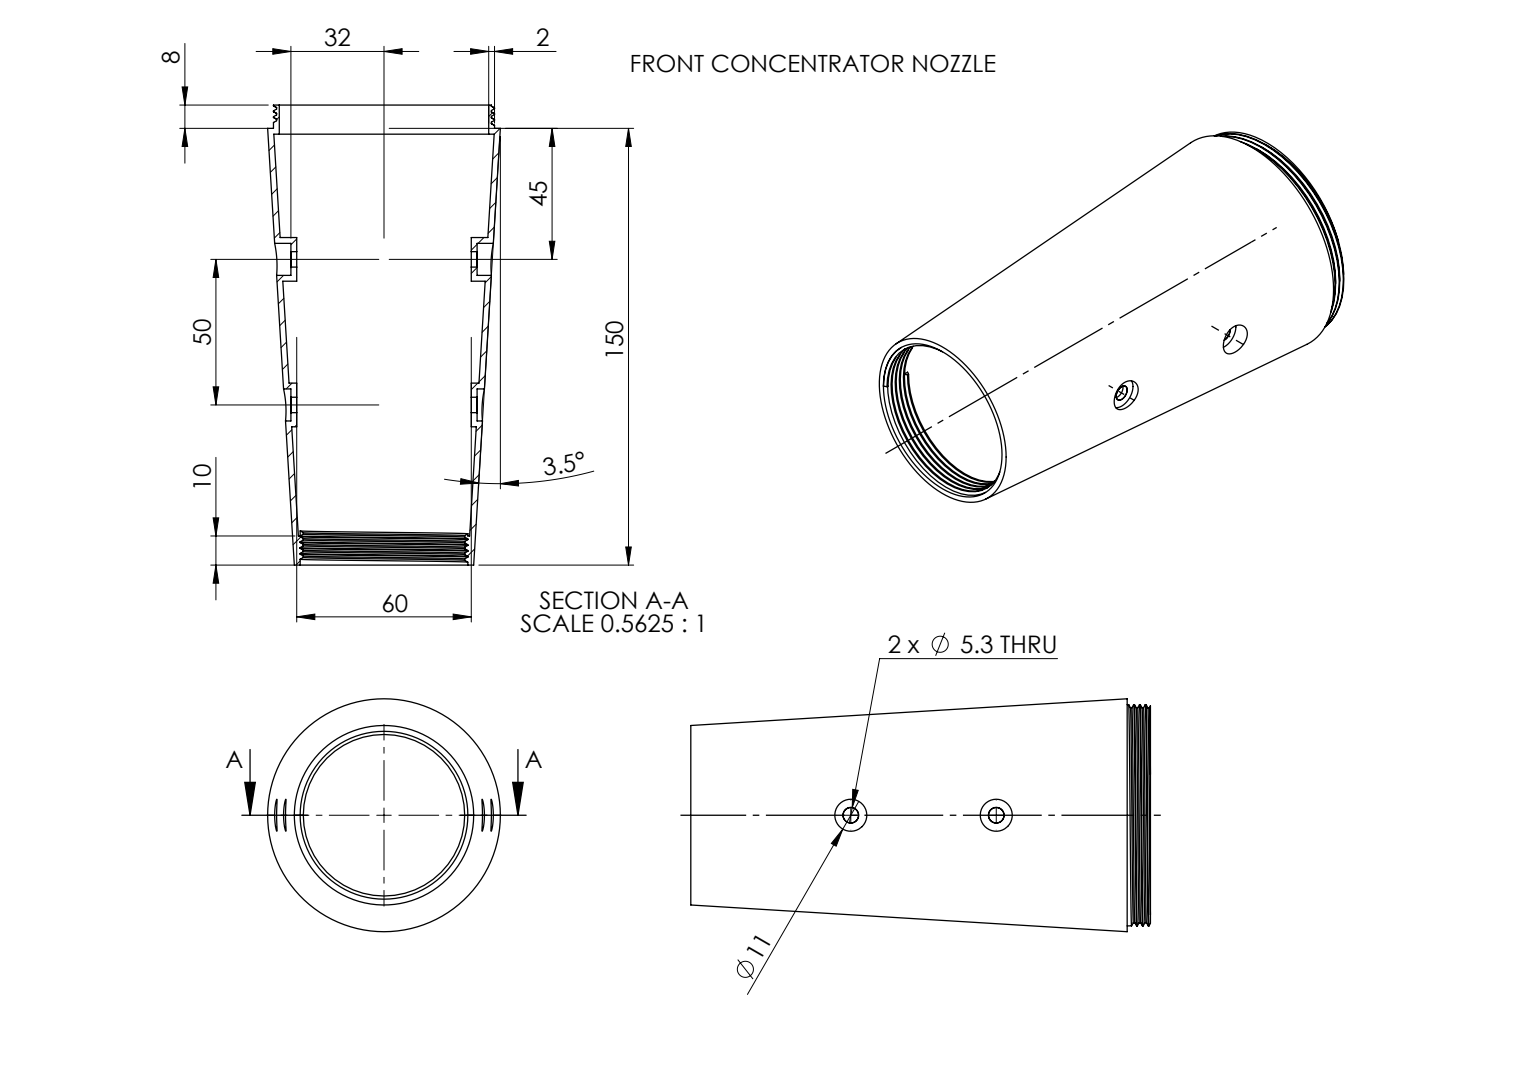
ISO-10303-21;
HEADER;
FILE_DESCRIPTION (('STEP AP214'),
    '1' );
FILE_NAME ('Front Concentrator Nozzle.step',
    '2026-10-04T13:31:42',
    ( '' ),
    ( '' ),
    'SwSTEP 2.0',
    'SolidWorks 2026',
    '' );
FILE_SCHEMA (( 'AUTOMOTIVE_DESIGN' ));
ENDSEC;

DATA;
#86=CARTESIAN_POINT ( 'NONE',  ( -31.23840969660177791, 7.314650797970922547, 96.67552899226033958 ) ) ;
#172=CARTESIAN_POINT ( 'NONE',  ( -11.40812507854755609, 35.11059874428196537, -7.524999997268813523 ) ) ;
#257=CARTESIAN_POINT ( 'NONE',  ( -36.88729982035408739, 1.776435236410510043, 50.21758054017369233 ) ) ;
#263=CARTESIAN_POINT ( 'NONE',  ( 22.44159573604009239, 16.30477369853692693, 146.0750000027311728 ) ) ;
#268=CARTESIAN_POINT ( 'NONE',  ( -5.359611314223446995E-15, 29.16686587814335496, 140.3750000027311842 ) ) ;
#301=EDGE_LOOP ( 'NONE', ( #33851, #130611, #76912, #84363 ) ) ;
#356=CARTESIAN_POINT ( 'NONE',  ( -23.31738231874055245, -16.94106989632524574, 144.4500000054623854 ) ) ;
#375=CYLINDRICAL_SURFACE ( 'NONE', #121053, 37.99626262588765968 ) ;
#425=CARTESIAN_POINT ( 'NONE',  ( 35.67631076299766590, 1.230297745838647261, 37.59750771353019871 ) ) ;
#465=DIRECTION ( 'NONE',  ( 0.000000000000000000, 0.000000000000000000, -1.000000000000000000 ) ) ;
#483=EDGE_LOOP ( 'NONE', ( #165279, #110182, #164294, #124142 ) ) ;
#616=CARTESIAN_POINT ( 'NONE',  ( 36.91746825000000598, -11.99521256947793546, -3.724999997268812812 ) ) ;
#704=CARTESIAN_POINT ( 'NONE',  ( -36.77423900702709858, -4.677204790287845526, 47.89930394225362420 ) ) ;
#735=CARTESIAN_POINT ( 'NONE',  ( 17.14385361876520264, -23.59649016807271238, 146.0750000027311728 ) ) ;
#760=CARTESIAN_POINT ( 'NONE',  ( 28.82186960331499392, -9.364793116373510529, 145.1500000054623456 ) ) ;
#773=EDGE_LOOP ( 'NONE', ( #134371, #137023, #169429, #7764 ) ) ;
#781=CARTESIAN_POINT ( 'NONE',  ( 8.906447517083057264, -27.41122689804191026, 142.5999999999999943 ) ) ;
#823=CARTESIAN_POINT ( 'NONE',  ( 37.99626262588763836, 12.34573411038918955, -2.647842220587803386 ) ) ;
#850=CARTESIAN_POINT ( 'NONE',  ( 8.571926809382603096, -26.38167802310801235, 145.4750000027311785 ) ) ;
#868=CARTESIAN_POINT ( 'NONE',  ( 11.74149087413294268, 36.13659316521247433, -6.602157773949822506 ) ) ;
#904=CARTESIAN_POINT ( 'NONE',  ( -8.906447517083060816, 27.41122689804195645, 149.5999999999999943 ) ) ;
#973=CARTESIAN_POINT ( 'NONE',  ( 3.556970738554033499E-15, -38.81732327939057825, -2.124999997268813612 ) ) ;
#974=CARTESIAN_POINT ( 'NONE',  ( -34.51819068884489639, 0.7175229865516564720, 89.53493623002425750 ) ) ;
#991=CARTESIAN_POINT ( 'NONE',  ( 29.86685920354754487, 21.69954338932564752, -3.924999997268812990 ) ) ;
#1033=ORIENTED_EDGE ( 'NONE', *, *, #63840, .F. ) ;
#1078=CARTESIAN_POINT ( 'NONE',  ( -32.23033374730685807, 4.573250637950163622, 89.03582022910542548 ) ) ;
#1088=CARTESIAN_POINT ( 'NONE',  ( -28.82186960331480208, 9.364793116373830273, 140.1500000054623740 ) ) ;
#1099=CYLINDRICAL_SURFACE ( 'NONE', #19317, 2.649999999999999467 ) ;
#1105=AXIS2_PLACEMENT_3D ( 'NONE', #147719, #164887, #181061 ) ;
#1163=CARTESIAN_POINT ( 'NONE',  ( -36.91746825000000598, 2.428612866367529932E-14, -7.124999997268813168 ) ) ;
#1250=AXIS2_PLACEMENT_3D ( 'NONE', #88283, #13443, #89288 ) ;
#1253=CARTESIAN_POINT ( 'NONE',  ( 22.44159573604009594, -16.30477369853687364, 148.1750000027311671 ) ) ;
#1258=CARTESIAN_POINT ( 'NONE',  ( -27.73933785331498925, -9.013057229001049109, 140.9750000027311501 ) ) ;
#1302=DIRECTION ( 'NONE',  ( 0.000000000000000000, 0.000000000000000000, 1.000000000000000000 ) ) ;
#1348=LINE ( 'NONE', #110523, #66983 ) ;
#1420=CARTESIAN_POINT ( 'NONE',  ( 34.67490207739297148, 3.335485537672782552, 51.73549893453298409 ) ) ;
#1511=ORIENTED_EDGE ( 'NONE', *, *, #22791, .F. ) ;
#1579=DIRECTION ( 'NONE',  ( 1.000000000000000000, -0.000000000000000000, 6.982962677686266711E-15 ) ) ;
#1583=CARTESIAN_POINT ( 'NONE',  ( 34.02657648861390527, -4.769071838117370454, 92.23683055719311596 ) ) ;
#1616=CARTESIAN_POINT ( 'NONE',  ( -29.86685920354755197, -21.69954338932560134, -4.424999997268812990 ) ) ;
#1692=DIRECTION ( 'NONE',  ( 0.000000000000000000, 0.000000000000000000, -1.000000000000000000 ) ) ;
#1709=CARTESIAN_POINT ( 'NONE',  ( -36.91128768240056957, -0.3593773198236934197, 50.50000000000003553 ) ) ;
#1739=CARTESIAN_POINT ( 'NONE',  ( -28.82186960331499037, 2.428612866367529932E-14, 150.0000000000000000 ) ) ;
#1764=CARTESIAN_POINT ( 'NONE',  ( -8.906447517083060816, 27.41122689804195645, 147.8500000054623627 ) ) ;
#1781=DIRECTION ( 'NONE',  ( 0.000000000000000000, -0.000000000000000000, -1.000000000000000000 ) ) ;
#1853=CARTESIAN_POINT ( 'NONE',  ( 27.73933785331498569, 2.768321779492822058E-14, 145.8750000027311842 ) ) ;
#1864=ADVANCED_FACE ( 'NONE', ( #142724 ), #159574, .T. ) ;
#1947=VERTEX_POINT ( 'NONE', #111400 ) ;
#1982=CARTESIAN_POINT ( 'NONE',  ( 11.40812507854755253, -35.11059874428192273, -10.52499999726881263 ) ) ;
#1987=EDGE_CURVE ( 'NONE', #137596, #48134, #24393, .T. ) ;
#1988=CARTESIAN_POINT ( 'NONE',  ( 33.68482864984028424, 4.779698632210292786, 97.74495643025990432 ) ) ;
#1999=CARTESIAN_POINT ( 'NONE',  ( -29.86685920354755552, 21.69954338932564397, -5.324999997268814234 ) ) ;
#2032=CARTESIAN_POINT ( 'NONE',  ( 34.45224964297659653, -5.970420695714325099, 49.56603145559587631 ) ) ;
#2046=AXIS2_PLACEMENT_3D ( 'NONE', #73162, #149985, #85294 ) ;
#2171=CARTESIAN_POINT ( 'NONE',  ( 11.40812507854754365, 35.11059874428196537, -7.724999997268813701 ) ) ;
#2215=DIRECTION ( 'NONE',  ( 0.000000000000000000, 0.000000000000000000, 1.000000000000000000 ) ) ;
#2256=CARTESIAN_POINT ( 'NONE',  ( 8.571926809382597767, 26.38167802310806209, 142.2750000027311899 ) ) ;
#2261=CARTESIAN_POINT ( 'NONE',  ( 1.784210473542230573E-15, -29.16686587814331588, 139.3750000027311842 ) ) ;
#2283=CIRCLE ( 'NONE', #5446, 0.2000000000000057288 ) ;
#2296=VERTEX_POINT ( 'NONE', #80063 ) ;
#2331=CARTESIAN_POINT ( 'NONE',  ( 8.571926809382603096, -26.38167802310801235, 143.9750000027312069 ) ) ;
#2582=CARTESIAN_POINT ( 'NONE',  ( 34.37111623004059169, -2.754365613946268443, 90.23597232697532888 ) ) ;
#2613=ORIENTED_EDGE ( 'NONE', *, *, #47794, .T. ) ;
#2618=CARTESIAN_POINT ( 'NONE',  ( -11.40812507854755609, 35.11059874428196537, -3.024999997268813523 ) ) ;
#2707=CARTESIAN_POINT ( 'NONE',  ( -37.99626262588766679, 2.428612866367529932E-14, -5.747842220587803475 ) ) ;
#2708=CARTESIAN_POINT ( 'NONE',  ( -37.19790397533368775, -4.369830079088519170, 41.64077531718623248 ) ) ;
#2736=CARTESIAN_POINT ( 'NONE',  ( 28.82186960331499392, -9.364793116373510529, 148.9000000000000057 ) ) ;
#2760=CARTESIAN_POINT ( 'NONE',  ( -27.73933785331498925, 9.013057229001089965, 148.7750000027311899 ) ) ;
#2851=CARTESIAN_POINT ( 'NONE',  ( -5.359611314223446995E-15, 29.16686587814335851, 144.3750000027311842 ) ) ;
#2869=CARTESIAN_POINT ( 'NONE',  ( 28.82186960331518222, 9.364793116373306248, 141.3500000054623911 ) ) ;
#2899=ORIENTED_EDGE ( 'NONE', *, *, #115308, .F. ) ;
#2975=CARTESIAN_POINT ( 'NONE',  ( 29.86685920354754487, 21.69954338932564752, -5.424999997268813878 ) ) ;
#2987=EDGE_CURVE ( 'NONE', #118975, #96409, #59563, .T. ) ;
#2993=CARTESIAN_POINT ( 'NONE',  ( 22.81625015709509441, 31.40387420917330275, -7.824999997268813345 ) ) ;
#3002=EDGE_LOOP ( 'NONE', ( #73351, #153883, #149706, #79021 ) ) ;
#3031=CARTESIAN_POINT ( 'NONE',  ( 34.75592306271658316, -1.707766843171824478, 52.30709029423474732 ) ) ;
#3169=CARTESIAN_POINT ( 'NONE',  ( 11.40812507854755253, -35.11059874428192273, -10.52499999726881263 ) ) ;
#3184=ORIENTED_EDGE ( 'NONE', *, *, #51790, .T. ) ;
#3210=CARTESIAN_POINT ( 'NONE',  ( -28.82186960331499037, 2.428612866367529932E-14, 149.1250000027311842 ) ) ;
#3216=CARTESIAN_POINT ( 'NONE',  ( -33.83559363775140838, -1.430799499857056789, 100.3228003899267975 ) ) ;
#3219=LINE ( 'NONE', #11975, #188941 ) ;
#3253=CARTESIAN_POINT ( 'NONE',  ( 17.14385361876520264, 23.59649016807275856, 148.6750000027311387 ) ) ;
#3325=CARTESIAN_POINT ( 'NONE',  ( -22.44159573604010305, 16.30477369853692338, 145.1750000027311671 ) ) ;
#3369=CARTESIAN_POINT ( 'NONE',  ( -28.82186960331494419, 9.364793116373629545, 147.8999999999999773 ) ) ;
#3373=DIRECTION ( 'NONE',  ( -1.000000000000000000, 0.000000000000000000, 0.000000000000000000 ) ) ;
#3407=ORIENTED_EDGE ( 'NONE', *, *, #43390, .F. ) ;
#3481=CARTESIAN_POINT ( 'NONE',  ( -36.91746825000000598, 2.428612866367529932E-14, -4.624999997268814056 ) ) ;
#3519=DIRECTION ( 'NONE',  ( 0.000000000000000000, 0.000000000000000000, 1.000000000000000000 ) ) ;
#3567=CARTESIAN_POINT ( 'NONE',  ( 33.68444218968561188, -5.327119193238885053, 96.41491933019777605 ) ) ;
#3600=CARTESIAN_POINT ( 'NONE',  ( 3.556970738554033499E-15, -38.81732327939057825, -8.124999997268814056 ) ) ;
#3673=CARTESIAN_POINT ( 'NONE',  ( -3.573655867282028392E-15, 2.428612866367529932E-14, 2.000000000000000000 ) ) ;
#3703=EDGE_CURVE ( 'NONE', #70870, #68071, #179075, .T. ) ;
#3721=CARTESIAN_POINT ( 'NONE',  ( -28.82186960331499037, 2.428612866367529932E-14, 148.0000000000000000 ) ) ;
#3743=CARTESIAN_POINT ( 'NONE',  ( 27.73933785331498569, 2.768321779492822058E-14, 147.8750000027311842 ) ) ;
#3833=CARTESIAN_POINT ( 'NONE',  ( 22.44159573604009594, -16.30477369853687364, 145.6750000027311671 ) ) ;
#3852=LINE ( 'NONE', #20027, #140137 ) ;
#3854=CARTESIAN_POINT ( 'NONE',  ( -37.99626262588766679, 2.428612866367529932E-14, -6.002157773949822861 ) ) ;
#3890=CARTESIAN_POINT ( 'NONE',  ( 23.31738231874054534, 16.94106989632529192, 149.1999999999999886 ) ) ;
#3957=CARTESIAN_POINT ( 'NONE',  ( 36.91746824999999887, 11.99521256947799053, -3.524999997268813079 ) ) ;
#3958=CARTESIAN_POINT ( 'NONE',  ( -33.83915642739259511, 1.250096592814743612, 100.3591031859434395 ) ) ;
#4011=CARTESIAN_POINT ( 'NONE',  ( 34.36934878537046956, -7.254149193659900519, 46.92043707032848943 ) ) ;
#4175=FACE_OUTER_BOUND ( 'NONE', #83053, .T. ) ;
#4234=CARTESIAN_POINT ( 'NONE',  ( -27.73933785331498925, 2.428612866367529932E-14, 138.8750000027311842 ) ) ;
#4242=CARTESIAN_POINT ( 'NONE',  ( -67.00000000000000000, -1.096058885236868847E-14, 100.5000000000010232 ) ) ;
#4305=CARTESIAN_POINT ( 'NONE',  ( 27.73933785331498569, 9.013057229001093518, 142.4750000027312069 ) ) ;
#4359=EDGE_CURVE ( 'NONE', #122084, #114881, #130090, .T. ) ;
#4381=CARTESIAN_POINT ( 'NONE',  ( 30.74264578624799782, 22.33583958711400541, -2.549999994537626602 ) ) ;
#4431=CARTESIAN_POINT ( 'NONE',  ( 32.00000000000000000, -1.230770033143102596E-14, 100.5000000000010232 ) ) ;
#4461=CARTESIAN_POINT ( 'NONE',  ( -22.81625015709510507, 31.40387420917330275, -6.924999997268812990 ) ) ;
#4548=CARTESIAN_POINT ( 'NONE',  ( 34.11707783341799427, -4.368959606072635005, 91.63974055655047835 ) ) ;
#4555=CLOSED_SHELL ( 'NONE', ( #90232, #12376, #39790, #49765, #196807, #195802, #5067, #178847, #90906, #29062, #71683, #37608, #132806, #83460, #86746, #142950, #9900, #188345, #21736, #102737, #129324, #36223, #83487, #180359, #110651, #151179, #135829, #116056, #163838, #21395, #184629, #66098, #113969, #161198, #91600, #44781, #54625, #152525, #139324, #99460, #181205, #19000, #32262, #11988, #77426, #192893, #49369, #139173, #138390, #165381, #24013, #108264, #157224, #194354, #83980, #9700, #103342, #135698, #72433, #186703, #66135, #146997, #103745, #47351, #199677, #22379, #63505, #38617, #191100, #189772, #111561, #137258, #44759, #98675, #18130, #51870, #110625, #156274, #9092, #133714, #77296, #1864 ) ) ;
#4582=CARTESIAN_POINT ( 'NONE',  ( -36.91746825000001309, 11.99521256947798342, -6.724999997268813701 ) ) ;
#4674=CARTESIAN_POINT ( 'NONE',  ( 31.26372923869871201, -6.750542664803641735, 98.30470173274461843 ) ) ;
#4689=VERTEX_POINT ( 'NONE', #24962 ) ;
#4691=AXIS2_PLACEMENT_3D ( 'NONE', #148800, #166959, #28461 ) ;
#4705=CARTESIAN_POINT ( 'NONE',  ( -28.82186960331499392, -9.364793116373526516, 146.1000000000000227 ) ) ;
#4727=CARTESIAN_POINT ( 'NONE',  ( -8.571926809382608425, 26.38167802310805854, 148.4750000027311785 ) ) ;
#4754=CARTESIAN_POINT ( 'NONE',  ( -28.82186960331499037, 2.428612866367529932E-14, 146.2500000054623683 ) ) ;
#4758=EDGE_CURVE ( 'NONE', #21601, #200018, #57632, .T. ) ;
#4944=CARTESIAN_POINT ( 'NONE',  ( 11.40812507854755253, -35.11059874428192273, -8.024999997268814411 ) ) ;
#4945=CARTESIAN_POINT ( 'NONE',  ( -33.81930014798969353, 1.942787237620518859, 100.1485738335251341 ) ) ;
#5003=ORIENTED_EDGE ( 'NONE', *, *, #126225, .F. ) ;
#5021=PLANE ( 'NONE',  #137868 ) ;
#5067=ADVANCED_FACE ( 'NONE', ( #165492 ), #104804, .F. ) ;
#5133=B_SPLINE_CURVE_WITH_KNOTS ( 'NONE', 3,
 ( #22604, #131776, #54935, #86265, #72103, #147955, #191443, #116607, #40770, #39759, #83256, #37764, #55931, #53938, #100430, #146946, #84250, #144931, #164126, #101422, #38774, #161108, #145931, #9442, #71107, #117606, #162111, #23608, #7413, #163114, #115613, #85254, #24617, #69096, #148953, #133776, #180309, #132773, #8435, #194460, #179306, #103443, #102439, #68094 ),
 .UNSPECIFIED., .F., .F.,
 ( 4, 2, 2, 2, 2, 2, 2, 2, 2, 2, 2, 2, 2, 2, 2, 2, 2, 2, 2, 2, 2, 4 ),
 ( 0.01750047681075387815, 0.01897230708297379873, 0.01970822221908375901, 0.02044413735519371930, 0.02191596762741363988, 0.02338779789963356393, 0.02485962817185348450, 0.02559554330796346561, 0.02633145844407343977, 0.02706737358018342088, 0.02780328871629339851, 0.02927511898851335725, 0.03074694926073331253, 0.03221877953295326780, 0.03295469466906326972, 0.03369060980517327164, 0.03516244007739326854, 0.03663427034961326545, 0.03737018548572325349, 0.03810610062183324154, 0.03957793089405323150, 0.04104976116627322147 ),
 .UNSPECIFIED. ) ;
#5169=DIRECTION ( 'NONE',  ( -1.000000000000000000, 0.000000000000000000, 0.000000000000000000 ) ) ;
#5174=EDGE_CURVE ( 'NONE', #71503, #154069, #101569, .T. ) ;
#5201=AXIS2_PLACEMENT_3D ( 'NONE', #184358, #1302, #42874 ) ;
#5229=CARTESIAN_POINT ( 'NONE',  ( 17.14385361876520264, -23.59649016807271238, 141.5750000027312012 ) ) ;
#5242=ORIENTED_EDGE ( 'NONE', *, *, #113163, .T. ) ;
#5303=CARTESIAN_POINT ( 'NONE',  ( -17.14385361876520975, 23.59649016807275856, 147.0750000027312012 ) ) ;
#5382=CARTESIAN_POINT ( 'NONE',  ( 23.48529157249600630, -32.32473071737749137, -7.049999994537626158 ) ) ;
#5402=ORIENTED_EDGE ( 'NONE', *, *, #181788, .T. ) ;
#5432=CARTESIAN_POINT ( 'NONE',  ( 11.40812507854754365, 35.11059874428196537, -3.724999997268813701 ) ) ;
#5446=AXIS2_PLACEMENT_3D ( 'NONE', #181467, #58113, #41956 ) ;
#5466=CARTESIAN_POINT ( 'NONE',  ( 11.40812507854755253, -35.11059874428192273, -2.024999997268813079 ) ) ;
#5554=CARTESIAN_POINT ( 'NONE',  ( 33.67956615508441587, -5.223713096473153072, 96.75862529643663379 ) ) ;
#5586=CARTESIAN_POINT ( 'NONE',  ( -29.86685920354755552, 21.69954338932564397, -8.824999997268815122 ) ) ;
#5680=CARTESIAN_POINT ( 'NONE',  ( 31.34418352700886601, -5.970234417100042101, 99.56646813413777863 ) ) ;
#5710=CARTESIAN_POINT ( 'NONE',  ( -23.31738231874055600, 16.94106989632528837, 149.7999999999999829 ) ) ;
#5731=CARTESIAN_POINT ( 'NONE',  ( -8.906447517083060816, 27.41122689804195645, 139.8500000054623911 ) ) ;
#5760=CARTESIAN_POINT ( 'NONE',  ( -17.81289503416611097, -24.51734667627696496, 146.5500000054623513 ) ) ;
#5769=ORIENTED_EDGE ( 'NONE', *, *, #148652, .F. ) ;
#5827=CARTESIAN_POINT ( 'NONE',  ( -17.14385361876520264, -23.59649016807271238, 139.1750000027311671 ) ) ;
#5946=CARTESIAN_POINT ( 'NONE',  ( 36.91746825000000598, -11.99521256947793546, -5.724999997268813701 ) ) ;
#5947=CARTESIAN_POINT ( 'NONE',  ( -33.90110335395768715, 5.206480924673157595, 93.21819085016213080 ) ) ;
#6003=DIRECTION ( 'NONE',  ( -7.709882115452472644E-15, 0.000000000000000000, 1.000000000000000000 ) ) ;
#6011=ORIENTED_EDGE ( 'NONE', *, *, #13792, .F. ) ;
#6026=CARTESIAN_POINT ( 'NONE',  ( -30.73962218707678673, 22.33364281372846705, -4.202157773949823927 ) ) ;
#6033=CARTESIAN_POINT ( 'NONE',  ( -40.00200000000003087, -1.071565949253934124E-14, 102.5000000000000142 ) ) ;
#6193=CARTESIAN_POINT ( 'NONE',  ( 14.18669005401828187, -34.08280046153741694, -8.000000000000001776 ) ) ;
#6232=CARTESIAN_POINT ( 'NONE',  ( 22.44159573604009239, 16.30477369853692693, 146.5750000027312012 ) ) ;
#6301=CARTESIAN_POINT ( 'NONE',  ( -32.00000000000000711, -5.510910596163089556E-15, 45.00000000000000000 ) ) ;
#6303=CARTESIAN_POINT ( 'NONE',  ( -5.359611314223446995E-15, 29.16686587814335851, 144.8750000027311842 ) ) ;
#6343=CARTESIAN_POINT ( 'NONE',  ( -31.80000000000000782, -1.130348995613007185E-14, 97.69999999999998863 ) ) ;
#6378=CARTESIAN_POINT ( 'NONE',  ( 30.74264578624799782, 22.33583958711400541, -6.549999994537627046 ) ) ;
#6427=CARTESIAN_POINT ( 'NONE',  ( -22.81625015709509441, -31.40387420917324590, -6.824999997268814234 ) ) ;
#6429=DIRECTION ( 'NONE',  ( 0.000000000000000000, 0.000000000000000000, -1.000000000000000000 ) ) ;
#6440=AXIS2_PLACEMENT_3D ( 'NONE', #168862, #94012, #61681 ) ;
#6459=CARTESIAN_POINT ( 'NONE',  ( -29.86685920354755552, 21.69954338932564397, -2.824999997268813345 ) ) ;
#6551=EDGE_CURVE ( 'NONE', #147696, #97386, #74235, .T. ) ;
#6582=CARTESIAN_POINT ( 'NONE',  ( -22.81625015709510507, 31.40387420917330275, -6.924999997268812990 ) ) ;
#6646=ORIENTED_EDGE ( 'NONE', *, *, #14461, .F. ) ;
#6703=CARTESIAN_POINT ( 'NONE',  ( -8.906447517083053711, -27.41122689804191026, 144.4000000000000057 ) ) ;
#6726=CARTESIAN_POINT ( 'NONE',  ( -8.906447517083053711, -27.41122689804191026, 142.6500000054623740 ) ) ;
#6736=SURFACE_STYLE_FILL_AREA ( #179627 ) ;
#6834=CARTESIAN_POINT ( 'NONE',  ( 23.31738231874054890, -16.94106989632523508, 148.7999999999999829 ) ) ;
#6838=CARTESIAN_POINT ( 'NONE',  ( 32.00000000000000000, -1.163414459189985801E-14, 92.35000000000000853 ) ) ;
#6875=ORIENTED_EDGE ( 'NONE', *, *, #116835, .F. ) ;
#6939=CARTESIAN_POINT ( 'NONE',  ( -29.86685920354755552, 21.69954338932564397, -8.824999997268815122 ) ) ;
#7104=ORIENTED_EDGE ( 'NONE', *, *, #128488, .T. ) ;
#7139=DIRECTION ( 'NONE',  ( 1.000000000000000000, 0.000000000000000000, 0.000000000000000000 ) ) ;
#7143=CARTESIAN_POINT ( 'NONE',  ( 36.44859680441125960, 5.987861874135487206, -7.999999999999996447 ) ) ;
#7191=CARTESIAN_POINT ( 'NONE',  ( 9.138071159678322175, -35.85733837751254782, -7.999999999999996447 ) ) ;
#7202=ORIENTED_EDGE ( 'NONE', *, *, #67479, .F. ) ;
#7228=CARTESIAN_POINT ( 'NONE',  ( 27.73933785331498214, 9.013057229001095294, 142.4750000027311785 ) ) ;
#7301=CARTESIAN_POINT ( 'NONE',  ( 17.14385361876520264, -23.59649016807270883, 142.0750000027311444 ) ) ;
#7304=DIRECTION ( 'NONE',  ( -1.000000000000000000, 0.000000000000000000, 0.000000000000000000 ) ) ;
#7377=CARTESIAN_POINT ( 'NONE',  ( -11.74264578624799782, -36.14014761921581709, -3.349999994537626868 ) ) ;
#7392=ORIENTED_EDGE ( 'NONE', *, *, #132031, .F. ) ;
#7413=CARTESIAN_POINT ( 'NONE',  ( 31.68669428337295102, 6.716517432552111977, 91.65365426639641555 ) ) ;
#7416=ORIENTED_EDGE ( 'NONE', *, *, #68419, .F. ) ;
#7428=CARTESIAN_POINT ( 'NONE',  ( -36.91746825000000598, 2.428612866367529932E-14, -5.124999997268813168 ) ) ;
#7459=CARTESIAN_POINT ( 'NONE',  ( -22.81625015709509441, -31.40387420917324590, -2.324999997268813345 ) ) ;
#7498=CARTESIAN_POINT ( 'NONE',  ( -30.00000000000000000, -1.130961319012580892E-14, 92.35000000000000853 ) ) ;
#7581=CARTESIAN_POINT ( 'NONE',  ( 36.91746825000000598, -11.99521256947793546, -5.724999997268813701 ) ) ;
#7615=AXIS2_PLACEMENT_3D ( 'NONE', #110151, #93979, #124319 ) ;
#7703=CARTESIAN_POINT ( 'NONE',  ( -28.82186960331499037, 2.428612866367529932E-14, 139.9999999999999716 ) ) ;
#7762=SHAPE_DEFINITION_REPRESENTATION ( #187433, #31381 ) ;
#7764=ORIENTED_EDGE ( 'NONE', *, *, #187248, .F. ) ;
#7876=DIRECTION ( 'NONE',  ( 0.000000000000000000, 0.000000000000000000, -1.000000000000000000 ) ) ;
#7934=EDGE_CURVE ( 'NONE', #98202, #176832, #121982, .T. ) ;
#7945=CARTESIAN_POINT ( 'NONE',  ( -17.14385361876520619, 23.59649016807275856, 149.0750000027311728 ) ) ;
#7982=CIRCLE ( 'NONE', #120998, 0.1999999999999987899 ) ;
#8002=DIRECTION ( 'NONE',  ( -0.000000000000000000, -0.000000000000000000, -1.000000000000000000 ) ) ;
#8146=CARTESIAN_POINT ( 'NONE',  ( 37.99626262588765258, -12.34573411038911672, -5.102157773949822506 ) ) ;
#8153=CARTESIAN_POINT ( 'NONE',  ( 29.32033176666156393, -22.46488766722420749, -8.000000000000003553 ) ) ;
#8154=EDGE_CURVE ( 'NONE', #53763, #106856, #120793, .T. ) ;
#8167=EDGE_LOOP ( 'NONE', ( #3184, #164472 ) ) ;
#8243=CARTESIAN_POINT ( 'NONE',  ( -22.44159573604010305, 16.30477369853692338, 143.1750000027311671 ) ) ;
#8248=CARTESIAN_POINT ( 'NONE',  ( -37.99626262588765968, -12.34573411038913626, -5.647842220587802942 ) ) ;
#8255=ORIENTED_EDGE ( 'NONE', *, *, #28811, .T. ) ;
#8281=VERTEX_POINT ( 'NONE', #97815 ) ;
#8320=CARTESIAN_POINT ( 'NONE',  ( -27.73933785331498925, 9.013057229001088189, 141.2750000027311899 ) ) ;
#8397=CARTESIAN_POINT ( 'NONE',  ( -30.74264578624800492, -22.33583958711396278, -7.549999994537627934 ) ) ;
#8406=ORIENTED_EDGE ( 'NONE', *, *, #70616, .F. ) ;
#8435=CARTESIAN_POINT ( 'NONE',  ( 32.45668260148360673, 3.101559039593180689, 88.16695215365970739 ) ) ;
#8605=CARTESIAN_POINT ( 'NONE',  ( 30.74264578624800137, -22.33583958711395212, -3.200000000000000178 ) ) ;
#8657=VECTOR ( 'NONE', #192387, 1000.000000000000000 ) ;
#8719=FACE_BOUND ( 'NONE', #63868, .T. ) ;
#8727=CARTESIAN_POINT ( 'NONE',  ( -28.82186960331499392, 9.364793116373565596, 148.1500000054624024 ) ) ;
#8729=CARTESIAN_POINT ( 'NONE',  ( 17.81289503416610742, 24.51734667627700404, 143.5500000054623513 ) ) ;
#8760=SURFACE_SIDE_STYLE ('',( #6736 ) ) ;
#8850=CIRCLE ( 'NONE', #154180, 35.99626262588765258 ) ;
#8921=EDGE_CURVE ( 'NONE', #11483, #170159, #195880, .T. ) ;
#8934=CARTESIAN_POINT ( 'NONE',  ( 28.83912964652353494, 23.35006605898203347, -8.000000000000001776 ) ) ;
#8944=AXIS2_PLACEMENT_3D ( 'NONE', #117188, #55516, #86851 ) ;
#8966=CARTESIAN_POINT ( 'NONE',  ( 11.40812507854754365, 35.11059874428196537, -9.224999997268813701 ) ) ;
#8977=AXIS2_PLACEMENT_3D ( 'NONE', #29250, #183915, #153562 ) ;
#8990=CARTESIAN_POINT ( 'NONE',  ( -34.40742850069382541, 7.501893140248845349, 45.46088305597102419 ) ) ;
#8996=CARTESIAN_POINT ( 'NONE',  ( 30.00000000000000000, -1.130961319012580892E-14, 97.65000000000000568 ) ) ;
#9032=VERTEX_POINT ( 'NONE', #57353 ) ;
#9083=AXIS2_PLACEMENT_3D ( 'NONE', #99154, #180038, #22332 ) ;
#9092=ADVANCED_FACE ( 'NONE', ( #165528 ), #46870, .T. ) ;
#9217=CARTESIAN_POINT ( 'NONE',  ( -34.40553910806575999, -2.436532241128162468, 90.06585364601160393 ) ) ;
#9219=CARTESIAN_POINT ( 'NONE',  ( -6.782741387738352223, -36.64508735834520081, -7.999999999999996447 ) ) ;
#9257=CARTESIAN_POINT ( 'NONE',  ( 17.14385361876520264, -23.59649016807271238, 146.0750000027311728 ) ) ;
#9332=CARTESIAN_POINT ( 'NONE',  ( 22.44159573604009594, -16.30477369853687364, 147.6750000027311671 ) ) ;
#9405=CARTESIAN_POINT ( 'NONE',  ( -38.00000000000001421, 12.34694845685046438, -7.849999994537626868 ) ) ;
#9442=CARTESIAN_POINT ( 'NONE',  ( 31.33330333603523954, 7.497710212630238402, 94.47580324309009825 ) ) ;
#9445=ORIENTED_EDGE ( 'NONE', *, *, #103944, .F. ) ;
#9449=CARTESIAN_POINT ( 'NONE',  ( 31.31738933903719513, -7.498949511226639331, 94.72411213025004884 ) ) ;
#9613=CARTESIAN_POINT ( 'NONE',  ( 38.00000000000000000, 12.34694845685046616, -2.900000000000000355 ) ) ;
#9665=AXIS2_PLACEMENT_3D ( 'NONE', #94111, #58812, #184156 ) ;
#9675=ORIENTED_EDGE ( 'NONE', *, *, #13792, .T. ) ;
#9700=ADVANCED_FACE ( 'NONE', ( #80442 ), #71788, .T. ) ;
#9732=CARTESIAN_POINT ( 'NONE',  ( -23.31738231874055600, 16.94106989632528837, 143.7999999999999829 ) ) ;
#9785=CARTESIAN_POINT ( 'NONE',  ( -6.019987952026120409E-15, 39.95163481335720235, -0.5021577739498228610 ) ) ;
#9796=ORIENTED_EDGE ( 'NONE', *, *, #93300, .F. ) ;
#9847=CARTESIAN_POINT ( 'NONE',  ( -28.82186960331499037, 2.781578969918950771E-14, 139.9999999999999716 ) ) ;
#9900=ADVANCED_FACE ( 'NONE', ( #169233 ), #375, .T. ) ;
#9940=CARTESIAN_POINT ( 'NONE',  ( 8.906447517083057264, -27.41122689804191026, 144.5999999999999943 ) ) ;
#9967=CARTESIAN_POINT ( 'NONE',  ( -11.40812507854754720, -35.11059874428192273, -10.22499999726881548 ) ) ;
#9990=CARTESIAN_POINT ( 'NONE',  ( -34.57898328185102343, 4.579095689294062410, 50.94499274836915248 ) ) ;
#10067=CARTESIAN_POINT ( 'NONE',  ( 32.00000000000000000, -6.184466335694137604E-15, 50.50000000000002842 ) ) ;
#10100=CARTESIAN_POINT ( 'NONE',  ( 11.74149087413294268, 36.13659316521247433, -2.602157773949823394 ) ) ;
#10216=CARTESIAN_POINT ( 'NONE',  ( -34.48725679702496194, -1.430676605895445430, 89.67714645826994513 ) ) ;
#10218=CARTESIAN_POINT ( 'NONE',  ( -34.63926591227897234, -15.08268834117409973, -8.000000000000003553 ) ) ;
#10251=ORIENTED_EDGE ( 'NONE', *, *, #50509, .T. ) ;
#10256=CARTESIAN_POINT ( 'NONE',  ( -8.571926809382608425, 26.38167802310805854, 144.9750000027312069 ) ) ;
#10261=( NAMED_UNIT ( * ) PLANE_ANGLE_UNIT ( ) SI_UNIT ( $, .RADIAN. ) );
#10405=CARTESIAN_POINT ( 'NONE',  ( -22.81625015709510507, 31.40387420917330275, -1.424999997268813212 ) ) ;
#10499=CARTESIAN_POINT ( 'NONE',  ( -8.571926809382608425, 26.38167802310805854, 146.4750000027311785 ) ) ;
#10532=ORIENTED_EDGE ( 'NONE', *, *, #7934, .F. ) ;
#10570=CARTESIAN_POINT ( 'NONE',  ( -31.23718726401125068, 7.254977440570235636, 96.91727682732809512 ) ) ;
#10571=CARTESIAN_POINT ( 'NONE',  ( 17.81289503416611453, -24.51734667627695785, 146.6999999999999886 ) ) ;
#10614=CARTESIAN_POINT ( 'NONE',  ( -38.00000000000001421, -12.34694845685042708, -5.900000000000000355 ) ) ;
#10674=EDGE_LOOP ( 'NONE', ( #77033, #138944, #32774, #21666 ) ) ;
#10732=CARTESIAN_POINT ( 'NONE',  ( 8.906447517083057264, -27.41122689804191026, 140.5999999999999943 ) ) ;
#10829=CONICAL_SURFACE ( 'NONE', #7615, 38.00373040315628259, 0.06108652381980166773 ) ;
#10936=CARTESIAN_POINT ( 'NONE',  ( -30.00000000000000000, -1.163414459189985801E-14, 87.50000000000000000 ) ) ;
#10962=CARTESIAN_POINT ( 'NONE',  ( 8.571926809382597767, 26.38167802310806209, 148.7750000027311899 ) ) ;
#10987=CARTESIAN_POINT ( 'NONE',  ( -34.77757469352546593, 0.9858555240219201155, 52.45108825929359142 ) ) ;
#11017=FACE_OUTER_BOUND ( 'NONE', #161873, .T. ) ;
#11100=CARTESIAN_POINT ( 'NONE',  ( -23.48298174826590667, 32.32155151706776053, -2.302157773949822683 ) ) ;
#11133=ORIENTED_EDGE ( 'NONE', *, *, #149523, .F. ) ;
#11213=CARTESIAN_POINT ( 'NONE',  ( 36.91746825000000598, -11.99521256947793546, -4.224999997268812812 ) ) ;
#11221=CARTESIAN_POINT ( 'NONE',  ( -37.99533089065118219, -0.2660902954431525469, -7.999999999999996447 ) ) ;
#11262=CARTESIAN_POINT ( 'NONE',  ( 8.571926809382603096, -26.38167802310801235, 139.9750000027311785 ) ) ;
#11410=CARTESIAN_POINT ( 'NONE',  ( 23.48529157249600630, -32.32473071737749137, -11.04999999453762527 ) ) ;
#11467=CARTESIAN_POINT ( 'NONE',  ( -34.74703293042581009, -1.945922946419438082, 52.24735972161445829 ) ) ;
#11483=VERTEX_POINT ( 'NONE', #13342 ) ;
#11496=CARTESIAN_POINT ( 'NONE',  ( -37.11214605083871731, 4.768680519348648339, 42.23634591622183621 ) ) ;
#11508=CARTESIAN_POINT ( 'NONE',  ( 17.14385361876520264, -23.59649016807271238, 145.5750000027312012 ) ) ;
#11622=CARTESIAN_POINT ( 'NONE',  ( -23.48529157249600985, 32.32473071737754111, -6.300000000000000711 ) ) ;
#11628=CARTESIAN_POINT ( 'NONE',  ( -30.00000000000000000, -1.163414459189985801E-14, 95.00000000000000000 ) ) ;
#11713=LINE ( 'NONE', #73380, #83913 ) ;
#11876=CARTESIAN_POINT ( 'NONE',  ( -32.00000000000000000, -1.163414459189985801E-14, 97.65000000000000568 ) ) ;
#11878=CARTESIAN_POINT ( 'NONE',  ( 37.57652299961964104, -0.7251171387572892257, 39.53617709569549277 ) ) ;
#11945=CARTESIAN_POINT ( 'NONE',  ( -3.573655867282028392E-15, 2.428612866367529932E-14, 139.9999999999999716 ) ) ;
#11973=CARTESIAN_POINT ( 'NONE',  ( 8.571926809382603096, -26.38167802310801235, 141.9750000027312069 ) ) ;
#11975=CARTESIAN_POINT ( 'NONE',  ( 37.99626262588765258, 2.893932880411085066E-14, 2.000000000000000000 ) ) ;
#11980=CARTESIAN_POINT ( 'NONE',  ( 30.00000000000000000, -5.186379194389041255E-15, 47.64999999999999858 ) ) ;
#11988=ADVANCED_FACE ( 'NONE', ( #52612 ), #20278, .T. ) ;
#12108=CARTESIAN_POINT ( 'NONE',  ( -11.74149087413295511, 36.13659316521247433, -4.147842220587803830 ) ) ;
#12202=AXIS2_PLACEMENT_3D ( 'NONE', #109134, #184987, #46471 ) ;
#12219=CARTESIAN_POINT ( 'NONE',  ( -29.86685920354755197, -21.69954338932560134, -4.924999997268813878 ) ) ;
#12225=CARTESIAN_POINT ( 'NONE',  ( -2.219726742498586258, -37.13270733954487213, -7.999999999999996447 ) ) ;
#12284=AXIS2_PLACEMENT_3D ( 'NONE', #126369, #112200, #6003 ) ;
#12376=ADVANCED_FACE ( 'NONE', ( #83104 ), #169393, .T. ) ;
#12407=CARTESIAN_POINT ( 'NONE',  ( 11.40812507854754365, 35.11059874428196537, -1.724999997268813479 ) ) ;
#12491=CARTESIAN_POINT ( 'NONE',  ( -37.43947335741456328, 2.756686112915582854, 40.22705064412460274 ) ) ;
#12497=CARTESIAN_POINT ( 'NONE',  ( 8.571926809382603096, -26.38167802310801235, 143.4750000027312069 ) ) ;
#12502=CARTESIAN_POINT ( 'NONE',  ( -8.571926809382608425, 26.38167802310805854, 142.4750000027312069 ) ) ;
#12591=EDGE_CURVE ( 'NONE', #81412, #115964, #185427, .T. ) ;
#12610=CARTESIAN_POINT ( 'NONE',  ( -23.48529157249599919, -32.32473071737750558, -5.700000000000000178 ) ) ;
#12659=CARTESIAN_POINT ( 'NONE',  ( 34.78522506798721992, 2.428612866353961525E-14, 52.50000000000000000 ) ) ;
#12807=CARTESIAN_POINT ( 'NONE',  ( -67.00000000000000000, -5.510910596163089556E-15, 45.00000000000000000 ) ) ;
#12852=EDGE_CURVE ( 'NONE', #70870, #34628, #145778, .T. ) ;
#12924=CARTESIAN_POINT ( 'NONE',  ( -16.59625950682774231, 33.98852600706017313, -7.999999999999994671 ) ) ;
#12927=CARTESIAN_POINT ( 'NONE',  ( -28.82186960331518932, -9.364793116373263615, 140.3500000054623627 ) ) ;
#12942=ORIENTED_EDGE ( 'NONE', *, *, #95173, .F. ) ;
#12956=CARTESIAN_POINT ( 'NONE',  ( -17.14385361876520264, -23.59649016807271593, 141.6750000027311103 ) ) ;
#12981=CARTESIAN_POINT ( 'NONE',  ( 28.82186960331498327, 2.781578969918950771E-14, 145.2500000054623683 ) ) ;
#13004=CARTESIAN_POINT ( 'NONE',  ( -40.00200000000003087, -5.510910596163089556E-15, 45.00000000000000000 ) ) ;
#13057=DIRECTION ( 'NONE',  ( 1.000000000000000000, 0.000000000000000000, 3.709348145883536076E-20 ) ) ;
#13120=ORIENTED_EDGE ( 'NONE', *, *, #12852, .T. ) ;
#13198=CARTESIAN_POINT ( 'NONE',  ( 29.86685920354754842, -21.69954338932559068, -10.32499999726881335 ) ) ;
#13204=CARTESIAN_POINT ( 'NONE',  ( 34.35276339089875108, 2.907959671212061004, 90.32815265678038941 ) ) ;
#13242=CARTESIAN_POINT ( 'NONE',  ( -17.14385361876520264, -23.59649016807271593, 139.6750000027311955 ) ) ;
#13270=DIRECTION ( 'NONE',  ( 0.000000000000000000, 0.000000000000000000, -1.000000000000000000 ) ) ;
#13305=ORIENTED_EDGE ( 'NONE', *, *, #168447, .F. ) ;
#13342=CARTESIAN_POINT ( 'NONE',  ( -28.82186960331499037, 2.428612866367529932E-14, 148.0000000000000000 ) ) ;
#13380=CARTESIAN_POINT ( 'NONE',  ( -36.91746825000001309, 11.99521256947798342, -1.224999997268813035 ) ) ;
#13443=DIRECTION ( 'NONE',  ( -1.000000000000000000, 0.000000000000000000, 0.000000000000000000 ) ) ;
#13461=CARTESIAN_POINT ( 'NONE',  ( -36.90816834587730000, 0.7173862878750039140, 50.46507289210754266 ) ) ;
#13466=EDGE_CURVE ( 'NONE', #80486, #64642, #91865, .T. ) ;
#13468=CARTESIAN_POINT ( 'NONE',  ( 27.73933785331498569, 2.768321779492822058E-14, 145.8750000027311842 ) ) ;
#13473=CARTESIAN_POINT ( 'NONE',  ( 22.44159573604009594, -16.30477369853687364, 141.6750000027311671 ) ) ;
#13541=CARTESIAN_POINT ( 'NONE',  ( -23.31738231874055245, -16.94106989632524574, 146.1999999999999886 ) ) ;
#13579=CARTESIAN_POINT ( 'NONE',  ( 23.48529157249600630, -32.32473071737749137, -9.300000000000002487 ) ) ;
#13582=FACE_OUTER_BOUND ( 'NONE', #190809, .T. ) ;
#13631=CARTESIAN_POINT ( 'NONE',  ( 34.64436006561229675, 3.766901597203519803, 51.50401746017936944 ) ) ;
#13792=EDGE_CURVE ( 'NONE', #56681, #90959, #182815, .T. ) ;
#13885=CIRCLE ( 'NONE', #126873, 37.87393738558669298 ) ;
#13929=CARTESIAN_POINT ( 'NONE',  ( -5.359611314223446995E-15, 29.16686587814335496, 144.8750000027311557 ) ) ;
#13953=CARTESIAN_POINT ( 'NONE',  ( 17.81289503416611453, -24.51734667627695785, 144.9500000054623854 ) ) ;
#13961=EDGE_CURVE ( 'NONE', #82818, #68886, #72967, .T. ) ;
#13982=CARTESIAN_POINT ( 'NONE',  ( -37.99626262588766679, 2.428612866367529932E-14, -1.747842220587805251 ) ) ;
#14016=CARTESIAN_POINT ( 'NONE',  ( -40.00200000000003087, -1.071565949253934124E-14, 102.5000000000000142 ) ) ;
#14041=CARTESIAN_POINT ( 'NONE',  ( -17.14385361876520975, 23.59649016807275856, 141.0750000027311728 ) ) ;
#14053=CIRCLE ( 'NONE', #127048, 2.700000000000001066 ) ;
#14075=B_SPLINE_CURVE_WITH_KNOTS ( 'NONE', 3,
 ( #94989, #75843, #108166, #63667, #47511, #78820, #74867, #169848, #13204, #167868, #137520, #199202, #186029, #198210, #184033, #14174, #59681, #77829, #140499, #168841, #155672, #44530, #123327, #60669, #122344, #93991, #1988, #31342, #109167, #106185, #183046, #138508, #45515, #92993, #121353, #29368, #17167, #154679, #30346, #90999 ),
 .UNSPECIFIED., .F., .F.,
 ( 4, 2, 2, 2, 2, 2, 2, 2, 2, 2, 2, 2, 2, 2, 2, 2, 2, 2, 2, 4 ),
 ( 0.004339806180219612543, 0.005417599276633671204, 0.006495392373047728998, 0.007034288921254766569, 0.007573185469461804140, 0.008650978565875881016, 0.009728771662289961361, 0.01080656475870404171, 0.01134546130691106020, 0.01188435785511808215, 0.01296215095153212260, 0.01403994404794615958, 0.01511773714436020002, 0.01619553024077424047, 0.01727332333718827745, 0.01835111643360231790, 0.01942890953001635487, 0.01996780607822336642, 0.02050670262643038144, 0.02158449572284441148 ),
 .UNSPECIFIED. ) ;
#14124=CARTESIAN_POINT ( 'NONE',  ( -37.58407650405589351, 1.968340676919130544E-14, 39.49999999999996447 ) ) ;
#14168=CARTESIAN_POINT ( 'NONE',  ( -22.81625015709510507, 31.40387420917330275, -9.424999997268812990 ) ) ;
#14174=CARTESIAN_POINT ( 'NONE',  ( 33.92112623720979059, 5.144804392130072124, 93.04721607740081879 ) ) ;
#14186=CARTESIAN_POINT ( 'NONE',  ( 11.40812507854754365, 35.11059874428196537, -5.724999997268812812 ) ) ;
#14250=VERTEX_POINT ( 'NONE', #128020 ) ;
#14259=( BOUNDED_CURVE ( )  B_SPLINE_CURVE ( 2, ( #54227, #8727, #193753, #106697, #135079, #181576, #168370, #91503, #150246, #45039, #29866 ),
 .UNSPECIFIED., .F., .F. ) 
 B_SPLINE_CURVE_WITH_KNOTS ( ( 3, 2, 2, 2, 2, 3 ),
 ( 0.000000000000000000, 0.02000000000000001776, 0.04000000000000003553, 0.06000000000000005329, 0.08000000000000007105, 0.1000000000000000888 ),
 .UNSPECIFIED. ) 
 CURVE ( )  GEOMETRIC_REPRESENTATION_ITEM ( )  RATIONAL_B_SPLINE_CURVE ( ( 1.000000000000000000, 0.9510565162951535312, 1.000000000000000000, 0.9510565162951535312, 1.000000000000000000, 0.9510565162951535312, 1.000000000000000000, 0.9510565162951535312, 1.000000000000000000, 0.9510565162951533091, 1.000000000000000222 ) ) 
 REPRESENTATION_ITEM ( '' )  );
#14262=CARTESIAN_POINT ( 'NONE',  ( -28.82186960331514669, -9.364793116373306248, 142.3500000054623911 ) ) ;
#14274=CARTESIAN_POINT ( 'NONE',  ( -31.64616484836360755, 2.655180720736634026, 102.0186121717492824 ) ) ;
#14328=CARTESIAN_POINT ( 'NONE',  ( -30.00000000000000000, -5.510910596163089556E-15, 45.00000000000000000 ) ) ;
#14363=CARTESIAN_POINT ( 'NONE',  ( 11.40812507854755253, -35.11059874428192273, -6.524999997268813523 ) ) ;
#14453=CARTESIAN_POINT ( 'NONE',  ( -5.359611314223446995E-15, 29.16686587814335496, 146.3750000027311842 ) ) ;
#14458=CARTESIAN_POINT ( 'NONE',  ( 17.14385361876520264, 23.59649016807275856, 142.1750000027311671 ) ) ;
#14461=EDGE_CURVE ( 'NONE', #89527, #45563, #88726, .T. ) ;
#14676=AXIS2_PLACEMENT_3D ( 'NONE', #64731, #192053, #127378 ) ;
#14682=EDGE_LOOP ( 'NONE', ( #50120, #17366 ) ) ;
#14703=AXIS2_PLACEMENT_3D ( 'NONE', #109409, #112392, #48747 ) ;
#14781=DIRECTION ( 'NONE',  ( -1.000000000000000000, -0.000000000000000000, -3.709348145883536076E-20 ) ) ;
#14817=CARTESIAN_POINT ( 'NONE',  ( 36.91746824999999887, 11.99521256947799053, -1.524999997268813745 ) ) ;
#14934=CARTESIAN_POINT ( 'NONE',  ( 27.73933785331498569, 2.768321779492822058E-14, 144.3750000027311842 ) ) ;
#14957=CARTESIAN_POINT ( 'NONE',  ( -35.68624576866248788, 0.9837712456775835612, 37.56068211393102274 ) ) ;
#15045=CARTESIAN_POINT ( 'NONE',  ( -17.14385361876520264, -23.59649016807271238, 141.1750000027311671 ) ) ;
#15089=( BOUNDED_SURFACE ( )  B_SPLINE_SURFACE ( 1, 2, ( 
 ( #135831, #169116, #91264, #151979, #58967, #46786, #104489, #42825, #166172, #106456, #92274, #61931, #199478, #78096, #44801, #152955, #15455, #151006, #28660, #197500, #182332, #119664, #153958, #77112, #43811, #14453, #45790, #105474, #263, #123600, #13468, #168135, #29631, #167161, #74159, #76116, #27673, #198485, #137793, #30621, #185295, #108445, #60944, #170121, #107442, #31616, #89313, #75131, #90295, #59957, #121624, #93265, #154951, #122619, #12497, #184309, #183320, #139765, #65914, #111430, #32609, #172112, #79094, #112422, #34592, #95262, #2256, #190269, #47786, #186305, #109437, #49764, #35583, #5229, #142754, #21413, #188288, #96250, #158917, #94262, #33599, #140767, #63939, #62930, #97229, #20407, #187306, #157937, #189286, #48776, #82056, #143750, #156945, #173117, #19428, #125607, #17438, #81075, #171119, #80093, #4234 ),
 ( #113407, #50764, #174113, #124610, #18442, #110431, #141761, #3253, #175098, #64926, #126586, #127586, #1253, #66911, #155942, #128575, #51746, #36566, #98221, #159924, #83070, #23418, #179118, #195278, #69921, #131587, #180125, #86079, #6232, #70923, #41593, #67911, #101234, #9257, #26432, #129564, #176105, #54745, #87082, #191262, #52737, #40586, #117420, #114404, #10256, #146748, #39575, #103257, #22418, #37575, #116418, #115426, #193272, #132590, #102257, #99238, #85066, #25442, #178107, #24431, #144747, #160926, #8243, #84068, #147770, #55746, #162923, #145747, #194279, #7228, #56760, #118432, #130575, #163944, #68913, #164939, #192270, #148767, #71915, #53752, #177116, #38586, #133587, #100242, #161924, #149758, #184072, #60707, #57759, #153722, #90067, #183086, #46549, #165933, #11262, #198249, #58730, #13242, #152725, #45556, #72934 ) ),
 .UNSPECIFIED., .F., .F., .F. ) 
 B_SPLINE_SURFACE_WITH_KNOTS ( ( 2, 2 ),
 ( 3, 2, 2, 2, 2, 2, 2, 2, 2, 2, 2, 2, 2, 2, 2, 2, 2, 2, 2, 2, 2, 2, 2, 2, 2, 2, 2, 2, 2, 2, 2, 2, 2, 2, 2, 2, 2, 2, 2, 2, 2, 2, 2, 2, 2, 2, 2, 2, 2, 2, 3 ),
 ( 0.000000000000000000, 1.000000000000000000 ),
 ( 0.000000000000000000, 0.02000000000000000042, 0.04000000000000000083, 0.05999999999999999778, 0.08000000000000000167, 0.1000000000000000056, 0.1199999999999999956, 0.1400000000000000133, 0.1600000000000000033, 0.1799999999999999933, 0.2000000000000000111, 0.2200000000000000011, 0.2399999999999999911, 0.2600000000000000089, 0.2800000000000000266, 0.2999999999999999889, 0.3200000000000000067, 0.3400000000000000244, 0.3599999999999999867, 0.3800000000000000044, 0.4000000000000000222, 0.4199999999999999845, 0.4400000000000000022, 0.4600000000000000200, 0.4799999999999999822, 0.5000000000000000000, 0.5200000000000000178, 0.5400000000000000355, 0.5600000000000000533, 0.5799999999999999600, 0.5999999999999999778, 0.6199999999999999956, 0.6400000000000000133, 0.6600000000000000311, 0.6800000000000000488, 0.6999999999999999556, 0.7199999999999999734, 0.7399999999999999911, 0.7600000000000000089, 0.7800000000000000266, 0.8000000000000000444, 0.8199999999999999512, 0.8399999999999999689, 0.8599999999999999867, 0.8800000000000000044, 0.9000000000000000222, 0.9200000000000000400, 0.9399999999999999467, 0.9599999999999999645, 0.9799999999999999822, 1.000000000000000000 ),
 .UNSPECIFIED. ) 
 GEOMETRIC_REPRESENTATION_ITEM ( )  RATIONAL_B_SPLINE_SURFACE ( (
 ( 1.000000000000000000, 0.9510565162951535312, 1.000000000000000000, 0.9510565162951535312, 1.000000000000000000, 0.9510565162951535312, 1.000000000000000000, 0.9510565162951535312, 1.000000000000000000, 0.9510565162951535312, 1.000000000000000000, 0.9510565162951535312, 1.000000000000000000, 0.9510565162951535312, 1.000000000000000000, 0.9510565162951535312, 1.000000000000000000, 0.9510565162951535312, 1.000000000000000000, 0.9510565162951535312, 1.000000000000000000, 0.9510565162951535312, 1.000000000000000000, 0.9510565162951535312, 1.000000000000000000, 0.9510565162951535312, 1.000000000000000000, 0.9510565162951535312, 1.000000000000000000, 0.9510565162951535312, 1.000000000000000000, 0.9510565162951535312, 1.000000000000000000, 0.9510565162951535312, 1.000000000000000000, 0.9510565162951535312, 1.000000000000000000, 0.9510565162951535312, 1.000000000000000000, 0.9510565162951535312, 1.000000000000000000, 0.9510565162951535312, 1.000000000000000000, 0.9510565162951535312, 1.000000000000000000, 0.9510565162951535312, 1.000000000000000000, 0.9510565162951535312, 1.000000000000000000, 0.9510565162951535312, 1.000000000000000000, 0.9510565162951535312, 1.000000000000000000, 0.9510565162951535312, 1.000000000000000000, 0.9510565162951535312, 1.000000000000000000, 0.9510565162951535312, 1.000000000000000000, 0.9510565162951535312, 1.000000000000000000, 0.9510565162951535312, 1.000000000000000000, 0.9510565162951535312, 1.000000000000000000, 0.9510565162951535312, 1.000000000000000000, 0.9510565162951535312, 1.000000000000000000, 0.9510565162951535312, 1.000000000000000000, 0.9510565162951535312, 1.000000000000000000, 0.9510565162951535312, 1.000000000000000000, 0.9510565162951535312, 1.000000000000000000, 0.9510565162951535312, 1.000000000000000000, 0.9510565162951535312, 1.000000000000000000, 0.9510565162951535312, 1.000000000000000000, 0.9510565162951535312, 1.000000000000000000, 0.9510565162951535312, 1.000000000000000000, 0.9510565162951535312, 1.000000000000000000, 0.9510565162951535312, 1.000000000000000000, 0.9510565162951535312, 1.000000000000000000, 0.9510565162951535312, 1.000000000000000000, 0.9510565162951535312, 1.000000000000000000, 0.9510565162951535312, 1.000000000000000000, 0.9510565162951535312, 1.000000000000000000),
 ( 1.000000000000000000, 0.9510565162951535312, 1.000000000000000000, 0.9510565162951535312, 1.000000000000000000, 0.9510565162951535312, 1.000000000000000000, 0.9510565162951535312, 1.000000000000000000, 0.9510565162951535312, 1.000000000000000000, 0.9510565162951535312, 1.000000000000000000, 0.9510565162951535312, 1.000000000000000000, 0.9510565162951535312, 1.000000000000000000, 0.9510565162951535312, 1.000000000000000000, 0.9510565162951535312, 1.000000000000000000, 0.9510565162951535312, 1.000000000000000000, 0.9510565162951535312, 1.000000000000000000, 0.9510565162951535312, 1.000000000000000000, 0.9510565162951535312, 1.000000000000000000, 0.9510565162951535312, 1.000000000000000000, 0.9510565162951535312, 1.000000000000000000, 0.9510565162951535312, 1.000000000000000000, 0.9510565162951535312, 1.000000000000000000, 0.9510565162951535312, 1.000000000000000000, 0.9510565162951535312, 1.000000000000000000, 0.9510565162951535312, 1.000000000000000000, 0.9510565162951535312, 1.000000000000000000, 0.9510565162951535312, 1.000000000000000000, 0.9510565162951535312, 1.000000000000000000, 0.9510565162951535312, 1.000000000000000000, 0.9510565162951535312, 1.000000000000000000, 0.9510565162951535312, 1.000000000000000000, 0.9510565162951535312, 1.000000000000000000, 0.9510565162951535312, 1.000000000000000000, 0.9510565162951535312, 1.000000000000000000, 0.9510565162951535312, 1.000000000000000000, 0.9510565162951535312, 1.000000000000000000, 0.9510565162951535312, 1.000000000000000000, 0.9510565162951535312, 1.000000000000000000, 0.9510565162951535312, 1.000000000000000000, 0.9510565162951535312, 1.000000000000000000, 0.9510565162951535312, 1.000000000000000000, 0.9510565162951535312, 1.000000000000000000, 0.9510565162951535312, 1.000000000000000000, 0.9510565162951535312, 1.000000000000000000, 0.9510565162951535312, 1.000000000000000000, 0.9510565162951535312, 1.000000000000000000, 0.9510565162951535312, 1.000000000000000000, 0.9510565162951535312, 1.000000000000000000, 0.9510565162951535312, 1.000000000000000000, 0.9510565162951535312, 1.000000000000000000, 0.9510565162951535312, 1.000000000000000000, 0.9510565162951535312, 1.000000000000000000, 0.9510565162951535312, 1.000000000000000000, 0.9510565162951535312, 1.000000000000000000) ) ) 
 REPRESENTATION_ITEM ( '' )  SURFACE ( )  );
#15172=CARTESIAN_POINT ( 'NONE',  ( 22.81625015709509441, 31.40387420917330275, -7.824999997268813345 ) ) ;
#15173=CARTESIAN_POINT ( 'NONE',  ( -33.92112623720979059, 5.144804392130072124, 93.04721607740081879 ) ) ;
#15189=CARTESIAN_POINT ( 'NONE',  ( 29.86685920354754487, 21.69954338932564752, -7.924999997268814766 ) ) ;
#15197=ORIENTED_EDGE ( 'NONE', *, *, #79032, .F. ) ;
#15250=EDGE_CURVE ( 'NONE', #50775, #1947, #163067, .T. ) ;
#15363=CARTESIAN_POINT ( 'NONE',  ( 29.86685920354754487, 21.69954338932564752, -7.924999997268814766 ) ) ;
#15413=CARTESIAN_POINT ( 'NONE',  ( -5.429308488886486681E-15, 30.30510711980690175, 143.4999999999999716 ) ) ;
#15415=CARTESIAN_POINT ( 'NONE',  ( 17.81289503416610742, 24.51734667627700404, 145.5500000054623797 ) ) ;
#15454=AXIS2_PLACEMENT_3D ( 'NONE', #90767, #73645, #87788 ) ;
#15455=CARTESIAN_POINT ( 'NONE',  ( -8.571926809382601320, -26.38167802310801591, 147.2750000027311899 ) ) ;
#15568=DIRECTION ( 'NONE',  ( 0.000000000000000000, 0.000000000000000000, -1.000000000000000000 ) ) ;
#15618=ORIENTED_EDGE ( 'NONE', *, *, #124331, .F. ) ;
#15731=ORIENTED_EDGE ( 'NONE', *, *, #141788, .F. ) ;
#15808=CARTESIAN_POINT ( 'NONE',  ( -29.86685920354755197, -21.69954338932560134, -2.424999997268813434 ) ) ;
#15853=EDGE_LOOP ( 'NONE', ( #182017, #104263, #40510 ) ) ;
#15899=CARTESIAN_POINT ( 'NONE',  ( -36.85371136276476278, -2.758154363750441096, 49.76185830465988147 ) ) ;
#15929=CARTESIAN_POINT ( 'NONE',  ( 8.571926809382603096, -26.38167802310801235, 143.9750000027312069 ) ) ;
#15953=FACE_OUTER_BOUND ( 'NONE', #53154, .T. ) ;
#15991=VERTEX_POINT ( 'NONE', #158132 ) ;
#15998=ORIENTED_EDGE ( 'NONE', *, *, #8921, .F. ) ;
#16043=CARTESIAN_POINT ( 'NONE',  ( 8.571926809382597767, 26.38167802310806209, 142.2750000027311899 ) ) ;
#16080=CYLINDRICAL_SURFACE ( 'NONE', #60174, 28.82186960331498682 ) ;
#16140=CARTESIAN_POINT ( 'NONE',  ( 30.00000000000000000, -1.163414459189985801E-14, 92.35000000000000853 ) ) ;
#16168=CARTESIAN_POINT ( 'NONE',  ( -36.91746825000000598, 2.428612866367529932E-14, -9.124999997268814056 ) ) ;
#16186=CARTESIAN_POINT ( 'NONE',  ( 11.40812507854755253, -35.11059874428192273, -6.524999997268813523 ) ) ;
#16222=CARTESIAN_POINT ( 'NONE',  ( 28.82186960331498327, 2.781578969918950771E-14, 149.0000000000000000 ) ) ;
#16273=DIRECTION ( 'NONE',  ( 1.000000000000000000, 0.000000000000000000, 0.000000000000000000 ) ) ;
#16286=EDGE_CURVE ( 'NONE', #15991, #14250, #130721, .T. ) ;
#16348=AXIS2_PLACEMENT_3D ( 'NONE', #65120, #110626, #168334 ) ;
#16360=CARTESIAN_POINT ( 'NONE',  ( 29.86685920354754842, -21.69954338932559068, -6.324999997268814234 ) ) ;
#16452=CARTESIAN_POINT ( 'NONE',  ( -8.571926809382601320, -26.38167802310801591, 139.2750000027311899 ) ) ;
#16497=CARTESIAN_POINT ( 'NONE',  ( 28.82186960331498327, 2.428612866367529932E-14, 139.9999999999999716 ) ) ;
#16611=FACE_OUTER_BOUND ( 'NONE', #95008, .T. ) ;
#16626=EDGE_CURVE ( 'NONE', #184655, #68071, #74756, .T. ) ;
#16667=ORIENTED_EDGE ( 'NONE', *, *, #171253, .T. ) ;
#16767=DIRECTION ( 'NONE',  ( 0.000000000000000000, 0.000000000000000000, -1.000000000000000000 ) ) ;
#16801=CARTESIAN_POINT ( 'NONE',  ( -36.91746825000000598, 2.428612866367529932E-14, -2.624999997268813168 ) ) ;
#16890=CARTESIAN_POINT ( 'NONE',  ( -36.88736642480385797, -1.774289666830922485, 50.21844423102493948 ) ) ;
#16920=CARTESIAN_POINT ( 'NONE',  ( -5.429308488886486681E-15, 30.30510711980690175, 147.5000000000000000 ) ) ;
#16944=CARTESIAN_POINT ( 'NONE',  ( 23.31738231874054890, -16.94106989632523508, 145.0500000054623513 ) ) ;
#17010=CARTESIAN_POINT ( 'NONE',  ( 23.48298174826589246, 32.32155151706776053, -2.447842220587803652 ) ) ;
#17035=CARTESIAN_POINT ( 'NONE',  ( -27.73933785331498925, 9.013057229001088189, 144.7750000027311614 ) ) ;
#17049=CARTESIAN_POINT ( 'NONE',  ( 32.00000000000000000, -5.186379194389041255E-15, 47.64999999999999858 ) ) ;
#17098=AXIS2_PLACEMENT_3D ( 'NONE', #199310, #153787, #73992 ) ;
#17134=FACE_OUTER_BOUND ( 'NONE', #126071, .T. ) ;
#17162=CARTESIAN_POINT ( 'NONE',  ( 22.81625015709509441, 31.40387420917330275, -9.824999997268811569 ) ) ;
#17167=CARTESIAN_POINT ( 'NONE',  ( 33.83915642739259511, 1.250096592814747165, 100.3591031859434395 ) ) ;
#17203=AXIS2_PLACEMENT_3D ( 'NONE', #13004, #46305, #77633 ) ;
#17306=LINE ( 'NONE', #170983, #63499 ) ;
#17349=CARTESIAN_POINT ( 'NONE',  ( -11.40812507854755609, 35.11059874428196537, -3.524999997268813523 ) ) ;
#17366=ORIENTED_EDGE ( 'NONE', *, *, #64977, .T. ) ;
#17413=CARTESIAN_POINT ( 'NONE',  ( -37.90990184318192036, -12.46459953034305101, -7.900967680773318236 ) ) ;
#17438=CARTESIAN_POINT ( 'NONE',  ( -8.571926809382601320, -26.38167802310801591, 139.2750000027311899 ) ) ;
#17451=ORIENTED_EDGE ( 'NONE', *, *, #68080, .T. ) ;
#17552=CARTESIAN_POINT ( 'NONE',  ( 3.766062262543149401E-15, -39.95556452105413570, -9.500000000000001776 ) ) ;
#17662=EDGE_CURVE ( 'NONE', #60305, #126834, #52285, .T. ) ;
#17663=VERTEX_POINT ( 'NONE', #183281 ) ;
#17679=CARTESIAN_POINT ( 'NONE',  ( 28.82186960331498327, 2.781578969918950771E-14, 145.0000000000000000 ) ) ;
#17723=VERTEX_POINT ( 'NONE', #29596 ) ;
#17768=CARTESIAN_POINT ( 'NONE',  ( 34.35275354914907098, -2.907972467998146460, 90.32821402270533895 ) ) ;
#17802=CARTESIAN_POINT ( 'NONE',  ( -5.950531402560715689E-15, 38.81732327939063509, -1.124999997268812946 ) ) ;
#17879=CYLINDRICAL_SURFACE ( 'NONE', #60326, 28.82186960331498682 ) ;
#17911=ORIENTED_EDGE ( 'NONE', *, *, #27194, .F. ) ;
#17923=CARTESIAN_POINT ( 'NONE',  ( -8.906447517083060816, 27.41122689804195645, 145.5999999999999943 ) ) ;
#17948=CARTESIAN_POINT ( 'NONE',  ( 23.31738231874054890, -16.94106989632523508, 139.0500000054623513 ) ) ;
#18040=CARTESIAN_POINT ( 'NONE',  ( 27.73933785331498569, 2.768321779492822058E-14, 141.8750000027311842 ) ) ;
#18043=ORIENTED_EDGE ( 'NONE', *, *, #68656, .F. ) ;
#18090=CIRCLE ( 'NONE', #2046, 7.500000000000007105 ) ;
#18130=ADVANCED_FACE ( 'NONE', ( #67874 ), #173079, .F. ) ;
#18158=CARTESIAN_POINT ( 'NONE',  ( -31.99364916731038022, -1.163414459189985801E-14, 95.00000000000000000 ) ) ;
#18164=CARTESIAN_POINT ( 'NONE',  ( 11.40812507854755253, -35.11059874428192273, -6.024999997268814411 ) ) ;
#18167=CARTESIAN_POINT ( 'NONE',  ( 23.48298174826590667, -32.32155151706770368, -3.047842220587803741 ) ) ;
#18181=CARTESIAN_POINT ( 'NONE',  ( 22.81625015709510151, -31.40387420917324590, -6.424999997268811214 ) ) ;
#18216=CARTESIAN_POINT ( 'NONE',  ( 34.71415419550759651, -2.652640888949069797, 52.01956328305328014 ) ) ;
#18351=CARTESIAN_POINT ( 'NONE',  ( 67.00000000000000000, -6.184466335694137604E-15, 50.50000000000002842 ) ) ;
#18354=CARTESIAN_POINT ( 'NONE',  ( -22.81625015709510507, 31.40387420917330275, -5.424999997268812990 ) ) ;
#18367=EDGE_CURVE ( 'NONE', #43523, #157920, #76737, .T. ) ;
#18382=AXIS2_PLACEMENT_3D ( 'NONE', #66188, #143019, #3519 ) ;
#18408=CARTESIAN_POINT ( 'NONE',  ( -23.31738231874055600, 16.94106989632528837, 146.0500000054623797 ) ) ;
#18419=CARTESIAN_POINT ( 'NONE',  ( 11.74149087413295156, -36.13659316521243881, -7.402157773949824104 ) ) ;
#18442=CARTESIAN_POINT ( 'NONE',  ( -8.571926809382608425, 26.38167802310805854, 148.9750000027311785 ) ) ;
#18446=CARTESIAN_POINT ( 'NONE',  ( 27.73933785331498925, -9.013057229001033122, 139.7750000027311899 ) ) ;
#18454=ORIENTED_EDGE ( 'NONE', *, *, #40331, .T. ) ;
#18512=DIRECTION ( 'NONE',  ( 0.000000000000000000, 0.000000000000000000, -1.000000000000000000 ) ) ;
#18514=CARTESIAN_POINT ( 'NONE',  ( 27.73933785331498569, 9.013057229001093518, 144.4750000027311785 ) ) ;
#18559=CARTESIAN_POINT ( 'NONE',  ( -5.429308488886486681E-15, 30.30510711980690175, 147.5000000000000000 ) ) ;
#18566=EDGE_CURVE ( 'NONE', #4689, #117112, #165893, .T. ) ;
#18654=DIRECTION ( 'NONE',  ( -1.000000000000000000, 0.000000000000000000, 0.000000000000000000 ) ) ;
#18674=CARTESIAN_POINT ( 'NONE',  ( 22.81625015709509441, 31.40387420917330275, -3.324999997268812901 ) ) ;
#18782=DIRECTION ( 'NONE',  ( 0.000000000000000000, 0.000000000000000000, 1.000000000000000000 ) ) ;
#18797=CARTESIAN_POINT ( 'NONE',  ( 22.81625015709509441, 31.40387420917330275, -5.324999997268812457 ) ) ;
#18810=EDGE_CURVE ( 'NONE', #189055, #21601, #98913, .T. ) ;
#18887=CARTESIAN_POINT ( 'NONE',  ( 31.99650548583503351, -5.647492055662687527, 90.04056618753070040 ) ) ;
#18916=CARTESIAN_POINT ( 'NONE',  ( 1.784210473542230573E-15, -29.16686587814331588, 139.8750000027311842 ) ) ;
#18940=CARTESIAN_POINT ( 'NONE',  ( -17.81289503416611097, -24.51734667627696496, 138.5500000054623229 ) ) ;
#19000=ADVANCED_FACE ( 'NONE', ( #147732 ), #194242, .F. ) ;
#19031=CARTESIAN_POINT ( 'NONE',  ( -17.14385361876520264, -23.59649016807271238, 145.1750000027311387 ) ) ;
#19152=CARTESIAN_POINT ( 'NONE',  ( 29.86685920354754487, 21.69954338932564752, -3.424999997268813434 ) ) ;
#19153=CARTESIAN_POINT ( 'NONE',  ( -33.86350577294170705, 5.311679113341315706, 93.56182321589967898 ) ) ;
#19196=ORIENTED_EDGE ( 'NONE', *, *, #82089, .T. ) ;
#19206=CARTESIAN_POINT ( 'NONE',  ( 34.80541354469661286, -6.720605140086532536, 41.66184804092134186 ) ) ;
#19230=CARTESIAN_POINT ( 'NONE',  ( 30.73962218707677607, 22.33364281372847060, -4.802157773949822683 ) ) ;
#19233=EDGE_CURVE ( 'NONE', #70870, #163891, #14075, .T. ) ;
#19317=AXIS2_PLACEMENT_3D ( 'NONE', #122463, #154798, #153803 ) ;
#19392=CARTESIAN_POINT ( 'NONE',  ( -33.85315667487628843, -0.3599896029658122276, 100.5000000000010232 ) ) ;
#19422=AXIS2_PLACEMENT_3D ( 'NONE', #80291, #465, #79307 ) ;
#19428=CARTESIAN_POINT ( 'NONE',  ( 8.571926809382603096, -26.38167802310801235, 139.4750000027311785 ) ) ;
#19432=CARTESIAN_POINT ( 'NONE',  ( 27.73933785331498569, 2.768321779492822058E-14, 139.8750000027311842 ) ) ;
#19440=ORIENTED_EDGE ( 'NONE', *, *, #127434, .F. ) ;
#19453=AXIS2_PLACEMENT_3D ( 'NONE', #116758, #151103, #71263 ) ;
#19463=ORIENTED_EDGE ( 'NONE', *, *, #40331, .F. ) ;
#19474=LINE ( 'NONE', #109491, #182511 ) ;
#19499=CARTESIAN_POINT ( 'NONE',  ( 27.73933785331498569, 9.013057229001093518, 146.4750000027311501 ) ) ;
#19575=CARTESIAN_POINT ( 'NONE',  ( -38.00000000000000711, 2.428612866367529932E-14, -3.749999994537626780 ) ) ;
#19594=AXIS2_PLACEMENT_3D ( 'NONE', #124218, #65533, #93882 ) ;
#19597=ORIENTED_EDGE ( 'NONE', *, *, #112389, .F. ) ;
#19627=CARTESIAN_POINT ( 'NONE',  ( -35.31558682697089324, -4.577067960279682879, 39.03840433125809994 ) ) ;
#19658=CARTESIAN_POINT ( 'NONE',  ( 11.40812507854754365, 35.11059874428196537, -5.224999997268813701 ) ) ;
#19776=CARTESIAN_POINT ( 'NONE',  ( -11.40812507854754720, -35.11059874428192273, -8.224999997268813701 ) ) ;
#19875=CARTESIAN_POINT ( 'NONE',  ( -3.573655867282028392E-15, 2.428612866367529932E-14, 0.000000000000000000 ) ) ;
#19895=CARTESIAN_POINT ( 'NONE',  ( 8.906447517083057264, -27.41122689804191026, 146.5999999999999943 ) ) ;
#19916=CARTESIAN_POINT ( 'NONE',  ( -22.44159573604010305, 16.30477369853692338, 148.6750000027311671 ) ) ;
#19938=CARTESIAN_POINT ( 'NONE',  ( -8.906447517083053711, -27.41122689804191026, 142.4000000000000057 ) ) ;
#19984=CARTESIAN_POINT ( 'NONE',  ( -67.00000000000000000, -4.837354856632041508E-15, 50.50000000000002842 ) ) ;
#20025=CARTESIAN_POINT ( 'NONE',  ( -23.31738231874055245, -16.94106989632524574, 148.1999999999999886 ) ) ;
#20027=CARTESIAN_POINT ( 'NONE',  ( -38.00373040315628970, 1.963201398428686990E-14, -0.1220970790697140096 ) ) ;
#20086=DIRECTION ( 'NONE',  ( -1.000000000000000000, 0.000000000000000000, -6.982962677686266711E-15 ) ) ;
#20128=CARTESIAN_POINT ( 'NONE',  ( 11.40812507854754365, 35.11059874428196537, -5.224999997268813701 ) ) ;
#20181=CARTESIAN_POINT ( 'NONE',  ( 35.70266437024449147, -0.4905633046376201012, 37.50000000000000000 ) ) ;
#20209=DIRECTION ( 'NONE',  ( -1.000000000000000000, 0.000000000000000000, 0.000000000000000000 ) ) ;
#20250=VECTOR ( 'NONE', #119732, 1000.000000000000000 ) ;
#20278=CYLINDRICAL_SURFACE ( 'NONE', #162906, 7.500000000000000000 ) ;
#20372=( BOUNDED_CURVE ( )  B_SPLINE_CURVE ( 2, ( #65569, #76761, #80733, #138435, #904, #139422, #123253, #140422, #3890, #200116, #50421 ),
 .UNSPECIFIED., .F., .T. ) 
 B_SPLINE_CURVE_WITH_KNOTS ( ( 3, 2, 2, 2, 2, 3 ),
 ( 0.000000000000000000, 0.02000000000000001776, 0.04000000000000003553, 0.06000000000000005329, 0.08000000000000007105, 0.1000000000000000888 ),
 .UNSPECIFIED. ) 
 CURVE ( )  GEOMETRIC_REPRESENTATION_ITEM ( )  RATIONAL_B_SPLINE_CURVE ( ( 1.000000000000000000, 0.9510565162951535312, 1.000000000000000000, 0.9510565162951535312, 1.000000000000000000, 0.9510565162951535312, 1.000000000000000000, 0.9510565162951535312, 1.000000000000000000, 0.9510565162951533091, 1.000000000000000222 ) ) 
 REPRESENTATION_ITEM ( '' )  );
#20407=CARTESIAN_POINT ( 'NONE',  ( -5.359611314223446995E-15, 29.16686587814335496, 140.3750000027311842 ) ) ;
#20418=ORIENTED_EDGE ( 'NONE', *, *, #116795, .T. ) ;
#20479=CARTESIAN_POINT ( 'NONE',  ( -8.571926809382601320, -26.38167802310801591, 147.7750000027311899 ) ) ;
#20529=FACE_OUTER_BOUND ( 'NONE', #10674, .T. ) ;
#20558=CARTESIAN_POINT ( 'NONE',  ( 11.74264578624799427, 36.14014761921585972, -6.349999994537625980 ) ) ;
#20598=DIRECTION ( 'NONE',  ( 1.000000000000000000, 0.000000000000000000, 0.000000000000000000 ) ) ;
#20606=DIRECTION ( 'NONE',  ( 0.000000000000000000, 0.000000000000000000, -1.000000000000000000 ) ) ;
#20608=CARTESIAN_POINT ( 'NONE',  ( -22.81625015709510507, 31.40387420917330275, -5.424999997268812990 ) ) ;
#20641=CARTESIAN_POINT ( 'NONE',  ( 22.81625015709510151, -31.40387420917324590, -5.924999997268812990 ) ) ;
#20728=CARTESIAN_POINT ( 'NONE',  ( 33.98208146068711244, -4.940236926081949420, 92.55634382532313964 ) ) ;
#20762=CARTESIAN_POINT ( 'NONE',  ( -36.91746825000001309, -11.99521256947794789, -6.524999997268810858 ) ) ;
#20855=CARTESIAN_POINT ( 'NONE',  ( 32.33375351741884174, -3.966103829525456259, 88.62974963220464986 ) ) ;
#20886=CARTESIAN_POINT ( 'NONE',  ( -8.571926809382608425, 26.38167802310805854, 140.9750000027312069 ) ) ;
#20907=CARTESIAN_POINT ( 'NONE',  ( -23.31738231874055600, 16.94106989632528837, 142.0500000054623513 ) ) ;
#21015=CARTESIAN_POINT ( 'NONE',  ( 28.82186960331496905, -9.364793116373544279, 148.8999999999999773 ) ) ;
#21020=CARTESIAN_POINT ( 'NONE',  ( 37.11169547541890523, -4.770708601134445281, 42.23953901806349620 ) ) ;
#21080=DIRECTION ( 'NONE',  ( 1.000000000000000000, -0.000000000000000000, -0.000000000000000000 ) ) ;
#21124=CARTESIAN_POINT ( 'NONE',  ( -36.91746825000001309, 11.99521256947798342, -4.724999997268811924 ) ) ;
#21176=LINE ( 'NONE', #82831, #188792 ) ;
#21183=DIRECTION ( 'NONE',  ( 0.000000000000000000, 0.000000000000000000, -1.000000000000000000 ) ) ;
#21201=FACE_OUTER_BOUND ( 'NONE', #139480, .T. ) ;
#21326=CARTESIAN_POINT ( 'NONE',  ( -36.91746825000001309, -11.99521256947794789, -11.02499999726881263 ) ) ;
#21353=AXIS2_PLACEMENT_3D ( 'NONE', #190463, #159104, #20598 ) ;
#21375=CARTESIAN_POINT ( 'NONE',  ( -33.67973855159211638, -4.949490125723493783, 97.42538428767439029 ) ) ;
#21395=ADVANCED_FACE ( 'NONE', ( #80861 ), #48559, .F. ) ;
#21407=EDGE_LOOP ( 'NONE', ( #199457, #55147, #162322, #160514, #189917, #90510 ) ) ;
#21413=CARTESIAN_POINT ( 'NONE',  ( 1.784210473542230573E-15, -29.16686587814331588, 141.3750000027311557 ) ) ;
#21447=VERTEX_POINT ( 'NONE', #110212 ) ;
#21468=EDGE_CURVE ( 'NONE', #17663, #172412, #30396, .T. ) ;
#21483=CARTESIAN_POINT ( 'NONE',  ( 22.44159573604009594, -16.30477369853687364, 142.1750000027311671 ) ) ;
#21561=CARTESIAN_POINT ( 'NONE',  ( 38.00000000000000000, 12.34694845685046616, -2.649999994537626247 ) ) ;
#21601=VERTEX_POINT ( 'NONE', #124386 ) ;
#21612=CARTESIAN_POINT ( 'NONE',  ( 37.57676386873052365, 0.7175261378074928587, 39.53500980800842513 ) ) ;
#21614=CARTESIAN_POINT ( 'NONE',  ( 11.40812507854755253, -35.11059874428192273, -6.524999997268813523 ) ) ;
#21628=AXIS2_PLACEMENT_3D ( 'NONE', #11628, #163294, #150127 ) ;
#21649=CARTESIAN_POINT ( 'NONE',  ( -36.91746825000000598, -11.99521256947794789, -2.524999997268813523 ) ) ;
#21666=ORIENTED_EDGE ( 'NONE', *, *, #68776, .T. ) ;
#21736=ADVANCED_FACE ( 'NONE', ( #79878 ), #141547, .T. ) ;
#21771=CARTESIAN_POINT ( 'NONE',  ( -23.48529157249600985, 32.32473071737754111, -0.2999999999999999334 ) ) ;
#21832=ORIENTED_EDGE ( 'NONE', *, *, #168639, .T. ) ;
#21892=CARTESIAN_POINT ( 'NONE',  ( 17.81289503416610742, 24.51734667627700404, 145.2999999999999829 ) ) ;
#21914=CARTESIAN_POINT ( 'NONE',  ( 28.82186960331498327, 2.781578969918950771E-14, 141.2500000054623683 ) ) ;
#21921=DIRECTION ( 'NONE',  ( 0.000000000000000000, 0.000000000000000000, -1.000000000000000000 ) ) ;
#22085=AXIS2_PLACEMENT_3D ( 'NONE', #187246, #127524, #5169 ) ;
#22127=CARTESIAN_POINT ( 'NONE',  ( -36.91746825000001309, -11.99521256947794789, -6.524999997268810858 ) ) ;
#22178=FACE_OUTER_BOUND ( 'NONE', #67549, .T. ) ;
#22263=DIRECTION ( 'NONE',  ( -1.000000000000000000, -0.000000000000000000, -0.000000000000000000 ) ) ;
#22332=DIRECTION ( 'NONE',  ( 1.000000000000000000, 0.000000000000000000, 0.000000000000000000 ) ) ;
#22358=CARTESIAN_POINT ( 'NONE',  ( -3.573655867282028392E-15, 2.428612866367529932E-14, 139.9999999999999716 ) ) ;
#22366=ORIENTED_EDGE ( 'NONE', *, *, #158172, .F. ) ;
#22379=ADVANCED_FACE ( 'NONE', ( #45321 ), #74667, .T. ) ;
#22380=CARTESIAN_POINT ( 'NONE',  ( -33.71409597518589152, -4.151718627496499892, 98.62556914322647117 ) ) ;
#22414=CARTESIAN_POINT ( 'NONE',  ( -31.40318257579882655, -7.397807925419286335, 93.74221852110633790 ) ) ;
#22418=CARTESIAN_POINT ( 'NONE',  ( 22.44159573604009239, 16.30477369853692693, 144.5750000027311728 ) ) ;
#22489=ORIENTED_EDGE ( 'NONE', *, *, #137048, .F. ) ;
#22492=CARTESIAN_POINT ( 'NONE',  ( 27.73933785331498569, 2.768321779492822058E-14, 144.3750000027311842 ) ) ;
#22537=CARTESIAN_POINT ( 'NONE',  ( -3.573655867282028392E-15, 2.428612866367529932E-14, 2.000000000000000000 ) ) ;
#22568=CARTESIAN_POINT ( 'NONE',  ( -38.00000000000001421, 12.34694845685046438, -3.849999994537626868 ) ) ;
#22604=CARTESIAN_POINT ( 'NONE',  ( 31.72709406046299918, -1.071565338629617092E-14, 102.5000000000000142 ) ) ;
#22621=CARTESIAN_POINT ( 'NONE',  ( -34.87614885797844977, -6.488895056989333554, 41.23117619273099876 ) ) ;
#22651=CARTESIAN_POINT ( 'NONE',  ( -36.91746825000000598, 2.428612866367529932E-14, -6.624999997268814056 ) ) ;
#22772=CARTESIAN_POINT ( 'NONE',  ( 37.99999999999999289, 2.893978650043524126E-14, -1.000000000000000000 ) ) ;
#22791=EDGE_CURVE ( 'NONE', #48134, #137596, #13885, .T. ) ;
#22892=CARTESIAN_POINT ( 'NONE',  ( 28.82186960331498327, 2.781578969918950771E-14, 141.0000000000000000 ) ) ;
#22915=CARTESIAN_POINT ( 'NONE',  ( -8.571926809382601320, -26.38167802310801591, 143.2750000027311899 ) ) ;
#22926=LINE ( 'NONE', #162427, #85530 ) ;
#23010=CARTESIAN_POINT ( 'NONE',  ( -22.44159573604010305, 16.30477369853692338, 140.6750000027311671 ) ) ;
#23024=CARTESIAN_POINT ( 'NONE',  ( -8.906447517083053711, -27.41122689804191026, 148.4000000000000057 ) ) ;
#23129=FACE_OUTER_BOUND ( 'NONE', #118201, .T. ) ;
#23131=DIRECTION ( 'NONE',  ( -0.06104853953485701173, -7.476289853398329258E-18, -0.9981347984218670311 ) ) ;
#23178=ORIENTED_EDGE ( 'NONE', *, *, #77338, .T. ) ;
#23326=CARTESIAN_POINT ( 'NONE',  ( -11.74149087413294623, -36.13659316521243881, -5.602157773949822506 ) ) ;
#23333=CARTESIAN_POINT ( 'NONE',  ( 36.62451201681301427, 4.795837538146646928, -8.000000000000001776 ) ) ;
#23414=CARTESIAN_POINT ( 'NONE',  ( -32.45678934495599322, -3.100610132747052550, 88.16656412605021842 ) ) ;
#23418=CARTESIAN_POINT ( 'NONE',  ( -27.73933785331498925, 9.013057229001089965, 147.2750000027311614 ) ) ;
#23514=DIRECTION ( 'NONE',  ( 1.000000000000000000, 0.000000000000000000, 0.000000000000000000 ) ) ;
#23569=CARTESIAN_POINT ( 'NONE',  ( -11.74264578624799782, -36.14014761921581709, -7.349999994537626868 ) ) ;
#23584=ORIENTED_EDGE ( 'NONE', *, *, #45012, .T. ) ;
#23600=VECTOR ( 'NONE', #193587, 1000.000000000000000 ) ;
#23608=CARTESIAN_POINT ( 'NONE',  ( 31.64990063023044442, 6.823060802858333496, 91.87658598274001065 ) ) ;
#23621=CARTESIAN_POINT ( 'NONE',  ( 37.55508611250748174, 1.249935417488353906, 39.64085810587564396 ) ) ;
#23777=CARTESIAN_POINT ( 'NONE',  ( 36.91746824999999177, 2.880721459617395097E-14, -7.624999997268813168 ) ) ;
#23825=DIRECTION ( 'NONE',  ( 0.000000000000000000, 0.000000000000000000, -1.000000000000000000 ) ) ;
#23896=CARTESIAN_POINT ( 'NONE',  ( -23.31738231874055600, 16.94106989632528837, 141.7999999999999829 ) ) ;
#23933=EDGE_CURVE ( 'NONE', #130647, #131569, #146223, .T. ) ;
#23998=VECTOR ( 'NONE', #40008, 1000.000000000000000 ) ;
#24013=ADVANCED_FACE ( 'NONE', ( #100706, #8719 ), #194742, .T. ) ;
#24030=CARTESIAN_POINT ( 'NONE',  ( 36.77186724307695442, -4.769522647520276770, 47.74487706083471039 ) ) ;
#24089=CARTESIAN_POINT ( 'NONE',  ( 17.81289503416610742, 24.51734667627700404, 145.2999999999999829 ) ) ;
#24105=CARTESIAN_POINT ( 'NONE',  ( 21.10861677039925866, 30.68312529381453757, -8.000000000000003553 ) ) ;
#24138=CARTESIAN_POINT ( 'NONE',  ( -17.14385361876520264, -23.59649016807271593, 147.6750000027311671 ) ) ;
#24168=DIRECTION ( 'NONE',  ( 0.000000000000000000, 0.000000000000000000, 1.000000000000000000 ) ) ;
#24198=ORIENTED_EDGE ( 'NONE', *, *, #114298, .F. ) ;
#24393=CIRCLE ( 'NONE', #14703, 37.87393738558669298 ) ;
#24406=CARTESIAN_POINT ( 'NONE',  ( -36.91746825000000598, 11.99521256947798520, -1.224999997268813257 ) ) ;
#24427=CARTESIAN_POINT ( 'NONE',  ( -31.25074303019346189, -7.456059982492099891, 95.94898436327792979 ) ) ;
#24431=CARTESIAN_POINT ( 'NONE',  ( -27.73933785331498925, -9.013057229001049109, 143.4750000027311785 ) ) ;
#24505=CARTESIAN_POINT ( 'NONE',  ( -5.359611314223446995E-15, 29.16686587814335851, 148.3750000027311842 ) ) ;
#24580=CARTESIAN_POINT ( 'NONE',  ( -6.020228577223754586E-15, 39.95556452105416412, -8.249999994537628112 ) ) ;
#24617=CARTESIAN_POINT ( 'NONE',  ( 31.99745974829802719, 5.643669518723337220, 90.03617080843918075 ) ) ;
#24630=CARTESIAN_POINT ( 'NONE',  ( 36.82860559483758323, 3.362349505172660624, 49.36759404993755851 ) ) ;
#24649=ORIENTED_EDGE ( 'NONE', *, *, #61842, .T. ) ;
#24708=VERTEX_POINT ( 'NONE', #151227 ) ;
#24744=CIRCLE ( 'NONE', #147407, 5.500000000000032863 ) ;
#24788=CARTESIAN_POINT ( 'NONE',  ( -11.74264578624800670, 36.14014761921585972, -6.400000000000000355 ) ) ;
#24907=CARTESIAN_POINT ( 'NONE',  ( 8.906447517083057264, -27.41122689804191026, 144.5999999999999943 ) ) ;
#24946=ORIENTED_EDGE ( 'NONE', *, *, #2987, .F. ) ;
#24958=CARTESIAN_POINT ( 'NONE',  ( -23.31738231874055245, -16.94106989632524574, 146.4500000054623854 ) ) ;
#24962=CARTESIAN_POINT ( 'NONE',  ( -36.91746825000000598, 2.428612866367529932E-14, -1.124999997268813390 ) ) ;
#25038=CARTESIAN_POINT ( 'NONE',  ( -37.99626262588762415, 12.34573411038923219, -7.847842220587805784 ) ) ;
#25115=DIRECTION ( 'NONE',  ( 0.000000000000000000, 0.000000000000000000, 1.000000000000000000 ) ) ;
#25118=CARTESIAN_POINT ( 'NONE',  ( -17.81289503416611097, -24.51734667627696496, 140.5500000054623513 ) ) ;
#25126=AXIS2_PLACEMENT_3D ( 'NONE', #120644, #182342, #163175 ) ;
#25147=CARTESIAN_POINT ( 'NONE',  ( 36.91746825000000598, -11.99521256947793546, -9.724999997268813701 ) ) ;
#25171=CARTESIAN_POINT ( 'NONE',  ( -34.74703179323500279, 1.946018278951686442, 52.24735473369669592 ) ) ;
#25401=CARTESIAN_POINT ( 'NONE',  ( -33.79565148458098633, -5.463178417057487302, 94.26852713616584367 ) ) ;
#25403=CARTESIAN_POINT ( 'NONE',  ( -22.19900124254457907, -30.24112288620522904, -8.000000000000000000 ) ) ;
#25415=CARTESIAN_POINT ( 'NONE',  ( -29.86685920354755197, -21.69954338932560134, -2.924999997268813878 ) ) ;
#25442=CARTESIAN_POINT ( 'NONE',  ( -17.14385361876520264, -23.59649016807271593, 143.6750000027311671 ) ) ;
#25514=CARTESIAN_POINT ( 'NONE',  ( -17.14385361876520264, -23.59649016807271238, 147.1750000027311671 ) ) ;
#25589=CARTESIAN_POINT ( 'NONE',  ( 22.81625015709509441, 31.40387420917330275, -1.824999997268813567 ) ) ;
#25600=CARTESIAN_POINT ( 'NONE',  ( -32.00000000000000000, -5.510910596163089556E-15, 47.64999999999999147 ) ) ;
#25651=CYLINDRICAL_SURFACE ( 'NONE', #1250, 5.500000000001017852 ) ;
#25751=CARTESIAN_POINT ( 'NONE',  ( -31.34393194264162830, 5.972569355670991342, 99.56318414118020144 ) ) ;
#25792=CARTESIAN_POINT ( 'NONE',  ( 30.74264578624800137, -22.33583958711395212, -5.200000000000001066 ) ) ;
#25910=CARTESIAN_POINT ( 'NONE',  ( 8.906447517083050158, 27.41122689804195645, 141.4000000000000057 ) ) ;
#25912=CARTESIAN_POINT ( 'NONE',  ( 8.906447517083057264, -27.41122689804191026, 138.8500000054623911 ) ) ;
#26109=CARTESIAN_POINT ( 'NONE',  ( 17.23098935283880095, 33.12085103290880284, -7.999999999999992895 ) ) ;
#26140=CARTESIAN_POINT ( 'NONE',  ( -8.571926809382608425, 26.38167802310805854, 148.9750000027311785 ) ) ;
#26142=CARTESIAN_POINT ( 'NONE',  ( -20.34036572606774484, 20.41983568886641365, 139.9999999999999716 ) ) ;
#26164=CARTESIAN_POINT ( 'NONE',  ( -34.98624150382332232, 6.090157606732317319, 40.61607269374898266 ) ) ;
#26243=CARTESIAN_POINT ( 'NONE',  ( 37.99626262588773074, -12.34573411038900126, -3.102157773949822062 ) ) ;
#26356=VERTEX_POINT ( 'NONE', #56796 ) ;
#26387=CARTESIAN_POINT ( 'NONE',  ( -22.81625015709510507, 31.40387420917330275, -1.424999997268813212 ) ) ;
#26394=CARTESIAN_POINT ( 'NONE',  ( -16.24461471443676430, -33.67505824103404422, -7.999999999999998224 ) ) ;
#26404=CARTESIAN_POINT ( 'NONE',  ( 67.00000000000000000, -1.230770033143102596E-14, 100.5000000000010232 ) ) ;
#26406=CARTESIAN_POINT ( 'NONE',  ( -29.86685920354755552, 21.69954338932564397, -3.324999997268813345 ) ) ;
#26427=ORIENTED_EDGE ( 'NONE', *, *, #148652, .T. ) ;
#26428=CARTESIAN_POINT ( 'NONE',  ( -31.37893600750393830, -5.659358439387607298, 99.94586368981258317 ) ) ;
#26432=CARTESIAN_POINT ( 'NONE',  ( 8.571926809382603096, -26.38167802310801235, 145.9750000027311785 ) ) ;
#26544=CARTESIAN_POINT ( 'NONE',  ( 28.82186960331507208, 9.364793116373459014, 147.1000000000000227 ) ) ;
#26576=CARTESIAN_POINT ( 'NONE',  ( 3.766062262543149401E-15, -39.95556452105413570, -9.249999994537628112 ) ) ;
#26593=CARTESIAN_POINT ( 'NONE',  ( -28.28060372831499336, 2.428612866367529932E-14, 139.6875000013656063 ) ) ;
#26617=VERTEX_POINT ( 'NONE', #188095 ) ;
#26627=CARTESIAN_POINT ( 'NONE',  ( 36.77885060843719600, 5.319724886534320518, 46.40826345025691069 ) ) ;
#26630=CARTESIAN_POINT ( 'NONE',  ( -34.64437015671237674, -3.766696895669992884, 51.50405731776596951 ) ) ;
#26673=CARTESIAN_POINT ( 'NONE',  ( 8.571926809382603096, -26.38167802310801235, 147.4750000027311785 ) ) ;
#26739=CARTESIAN_POINT ( 'NONE',  ( -3.573655867282028392E-15, 2.428612866367529932E-14, 0.000000000000000000 ) ) ;
#26743=CARTESIAN_POINT ( 'NONE',  ( -31.69373074887817765, 1.710217150889093984, 102.3065243757511098 ) ) ;
#26785=CARTESIAN_POINT ( 'NONE',  ( -11.74264578624800670, 36.14014761921585972, -2.400000000000000355 ) ) ;
#26905=LINE ( 'NONE', #138032, #75540 ) ;
#26907=CARTESIAN_POINT ( 'NONE',  ( 28.82186960331511827, 9.364793116373395065, 143.3500000054623911 ) ) ;
#26971=ORIENTED_EDGE ( 'NONE', *, *, #93425, .F. ) ;
#27020=ORIENTED_EDGE ( 'NONE', *, *, #119343, .T. ) ;
#27024=DIRECTION ( 'NONE',  ( 1.000000000000000000, 0.000000000000000000, 0.000000000000000000 ) ) ;
#27110=CARTESIAN_POINT ( 'NONE',  ( 3.444780402933648400, 37.36484951828411738, -8.000000000000003553 ) ) ;
#27183=DIRECTION ( 'NONE',  ( 1.000000000000000000, -0.000000000000000000, 6.982962677686266711E-15 ) ) ;
#27194=EDGE_CURVE ( 'NONE', #17663, #130010, #45803, .T. ) ;
#27214=DIRECTION ( 'NONE',  ( -1.000000000000000000, -0.000000000000000000, -3.709348145883536076E-20 ) ) ;
#27248=AXIS2_PLACEMENT_3D ( 'NONE', #90715, #185727, #152398 ) ;
#27271=CARTESIAN_POINT ( 'NONE',  ( -37.99626262588765968, 12.34573411038917179, -2.102157773949823394 ) ) ;
#27273=VECTOR ( 'NONE', #87400, 1000.000000000000000 ) ;
#27310=CIRCLE ( 'NONE', #30597, 2.649999999999999467 ) ;
#27343=CARTESIAN_POINT ( 'NONE',  ( 18.54787882382429487, -32.01089502393746500, -8.000000000000000000 ) ) ;
#27383=CARTESIAN_POINT ( 'NONE',  ( -22.81625015709509441, -31.40387420917324590, -2.824999997268812901 ) ) ;
#27393=AXIS2_PLACEMENT_3D ( 'NONE', #34112, #145255, #133092 ) ;
#27403=CARTESIAN_POINT ( 'NONE',  ( -11.40812507854754720, -35.11059874428192273, -2.724999997268813257 ) ) ;
#27437=SURFACE_SIDE_STYLE ('',( #88078 ) ) ;
#27544=DIRECTION ( 'NONE',  ( 1.000000000000000000, 0.000000000000000000, 3.709348145883536076E-20 ) ) ;
#27553=COLOUR_RGB ( '', 0.66274510, 0.83137255, 0.94901961) ;
#27582=CARTESIAN_POINT ( 'NONE',  ( -23.48529157249600985, 32.32473071737754111, -10.04999999453762705 ) ) ;
#27598=EDGE_LOOP ( 'NONE', ( #27020, #125207, #145675, #94863 ) ) ;
#27635=CARTESIAN_POINT ( 'NONE',  ( 36.86305638906669202, 5.498848518248650841, 44.61989603102466617 ) ) ;
#27667=CARTESIAN_POINT ( 'NONE',  ( 40.00000000000001421, 2.428612866367529932E-14, 0.000000000000000000 ) ) ;
#27673=CARTESIAN_POINT ( 'NONE',  ( -8.571926809382601320, -26.38167802310801591, 145.2750000027311899 ) ) ;
#27678=CARTESIAN_POINT ( 'NONE',  ( -8.571926809382608425, 26.38167802310805854, 144.4750000027312069 ) ) ;
#27787=CARTESIAN_POINT ( 'NONE',  ( -6.020228577223754586E-15, 39.95556452105416412, -4.500000000000000888 ) ) ;
#27839=CARTESIAN_POINT ( 'NONE',  ( 35.02332884957463932, 5.945191563609818708, 40.42135061281683761 ) ) ;
#27873=DIRECTION ( 'NONE',  ( 0.000000000000000000, 0.000000000000000000, -1.000000000000000000 ) ) ;
#27895=ORIENTED_EDGE ( 'NONE', *, *, #15250, .T. ) ;
#28042=CARTESIAN_POINT ( 'NONE',  ( 37.52651979737520094, -1.772832052285338689, 39.78107084225509027 ) ) ;
#28109=( BOUNDED_CURVE ( )  B_SPLINE_CURVE ( 2, ( #42276, #72609, #40262, #74591, #55427, #120090, #103934, #25118, #28116, #12927, #73612 ),
 .UNSPECIFIED., .F., .F. ) 
 B_SPLINE_CURVE_WITH_KNOTS ( ( 3, 2, 2, 2, 2, 3 ),
 ( 0.7000000000000006217, 0.7200000000000006395, 0.7400000000000006573, 0.7600000000000006750, 0.7800000000000006928, 0.8000000000000007105 ),
 .UNSPECIFIED. ) 
 CURVE ( )  GEOMETRIC_REPRESENTATION_ITEM ( )  RATIONAL_B_SPLINE_CURVE ( ( 0.9999999999999983347, 0.9510565162951551965, 1.000000000000000000, 0.9510565162951535312, 1.000000000000000000, 0.9510565162951535312, 1.000000000000000000, 0.9510565162951535312, 1.000000000000000000, 0.9510565162951518658, 1.000000000000001554 ) ) 
 REPRESENTATION_ITEM ( '' )  );
#28116=CARTESIAN_POINT ( 'NONE',  ( -23.31738231874055245, -16.94106989632524574, 140.4500000054623854 ) ) ;
#28142=CARTESIAN_POINT ( 'NONE',  ( -8.571926809382601320, -26.38167802310801591, 141.7750000027311899 ) ) ;
#28166=CARTESIAN_POINT ( 'NONE',  ( -35.02332884957466064, 5.945191563609817820, 40.42135061281684472 ) ) ;
#28176=DIRECTION ( 'NONE',  ( 0.000000000000000000, 0.000000000000000000, -1.000000000000000000 ) ) ;
#28222=CIRCLE ( 'NONE', #112169, 30.82560697742735556 ) ;
#28252=ORIENTED_EDGE ( 'NONE', *, *, #58814, .T. ) ;
#28260=ORIENTED_EDGE ( 'NONE', *, *, #60978, .T. ) ;
#28360=DIRECTION ( 'NONE',  ( 1.000000000000000000, 0.000000000000000000, 0.000000000000000000 ) ) ;
#28384=CARTESIAN_POINT ( 'NONE',  ( 29.86685920354754487, 21.69954338932564752, -9.924999997268812990 ) ) ;
#28390=CARTESIAN_POINT ( 'NONE',  ( 30.73962218707677962, -22.33364281372841376, -1.202157773949823039 ) ) ;
#28461=DIRECTION ( 'NONE',  ( 1.000000000000000000, 0.000000000000000000, 0.000000000000000000 ) ) ;
#28493=CYLINDRICAL_SURFACE ( 'NONE', #17098, 5.500000000001017852 ) ;
#28570=CARTESIAN_POINT ( 'NONE',  ( -29.86685920354755197, -21.69954338932560134, -2.924999997268813878 ) ) ;
#28582=ORIENTED_EDGE ( 'NONE', *, *, #49370, .F. ) ;
#28660=CARTESIAN_POINT ( 'NONE',  ( -22.44159573604009950, -16.30477369853688430, 147.0750000027312012 ) ) ;
#28665=CARTESIAN_POINT ( 'NONE',  ( 27.73933785331498214, 9.013057229001095294, 141.9750000027311501 ) ) ;
#28772=CARTESIAN_POINT ( 'NONE',  ( 38.00000000000000711, -12.34694845685040754, -1.099999999999999645 ) ) ;
#28811=EDGE_CURVE ( 'NONE', #189747, #83417, #46820, .T. ) ;
#28824=CARTESIAN_POINT ( 'NONE',  ( 34.40742850069380410, 7.501893140248843572, 45.46088305597103130 ) ) ;
#28948=CARTESIAN_POINT ( 'NONE',  ( 30.73962218707677607, 22.33364281372847060, -0.8021577739498229054 ) ) ;
#29005=EDGE_LOOP ( 'NONE', ( #150930, #57009 ) ) ;
#29062=ADVANCED_FACE ( 'NONE', ( #126894 ), #63248, .T. ) ;
#29090=CARTESIAN_POINT ( 'NONE',  ( -37.47059448506522727, -2.437326220201143201, 40.06626038917661248 ) ) ;
#29103=PRODUCT ( 'Front Concentrator Nozzle', 'Front Concentrator Nozzle', '', ( #84596 ) ) ;
#29122=CARTESIAN_POINT ( 'NONE',  ( -8.571926809382601320, -26.38167802310801591, 145.7750000027311899 ) ) ;
#29146=CARTESIAN_POINT ( 'NONE',  ( -28.82186960331499037, 2.428612866367529932E-14, 146.2500000054623683 ) ) ;
#29166=CARTESIAN_POINT ( 'NONE',  ( -30.00000000000000000, -5.186379194389042044E-15, 42.35000000000000853 ) ) ;
#29235=CARTESIAN_POINT ( 'NONE',  ( -17.14385361876520264, -23.59649016807271238, 141.6750000027311387 ) ) ;
#29250=CARTESIAN_POINT ( 'NONE',  ( -32.00000000000000000, -1.163414459189985801E-14, 95.00000000000000000 ) ) ;
#29362=CARTESIAN_POINT ( 'NONE',  ( -22.81625015709509441, -31.40387420917324590, -2.324999997268813789 ) ) ;
#29363=CARTESIAN_POINT ( 'NONE',  ( -34.46456012332993168, 1.775814316247263713, 89.78225565739067804 ) ) ;
#29368=CARTESIAN_POINT ( 'NONE',  ( 33.83483822987808765, 1.427510505796701690, 100.3145928531378672 ) ) ;
#29380=CARTESIAN_POINT ( 'NONE',  ( -36.91746825000000598, 11.99521256947798520, -5.224999997268812812 ) ) ;
#29546=CARTESIAN_POINT ( 'NONE',  ( -22.81625015709509441, -31.40387420917324590, -8.824999997268811569 ) ) ;
#29596=CARTESIAN_POINT ( 'NONE',  ( 30.00000000000000711, -5.510910596163089556E-15, 37.50000000000000000 ) ) ;
#29625=CARTESIAN_POINT ( 'NONE',  ( -36.77100073307799022, 4.779104515855422619, 47.74589100149062659 ) ) ;
#29631=CARTESIAN_POINT ( 'NONE',  ( 22.44159573604009594, -16.30477369853687364, 145.6750000027311671 ) ) ;
#29636=CARTESIAN_POINT ( 'NONE',  ( 27.73933785331498214, 9.013057229001095294, 145.9750000027311785 ) ) ;
#29667=CARTESIAN_POINT ( 'NONE',  ( -32.00000000000000000, -1.163414459189985801E-14, 89.49999999999897682 ) ) ;
#29669=EDGE_LOOP ( 'NONE', ( #85230, #152997, #142160, #142681 ) ) ;
#29673=ORIENTED_EDGE ( 'NONE', *, *, #139182, .T. ) ;
#29683=EDGE_CURVE ( 'NONE', #154069, #83417, #19474, .T. ) ;
#29746=CARTESIAN_POINT ( 'NONE',  ( 23.48529157249599919, 32.32473071737754111, -8.700000000000002842 ) ) ;
#29798=CARTESIAN_POINT ( 'NONE',  ( 35.31606782002515388, 4.574060259307362486, 39.03637847775443248 ) ) ;
#29866=CARTESIAN_POINT ( 'NONE',  ( 28.82186960331498327, 2.781578969918950771E-14, 147.2500000054623683 ) ) ;
#29989=CARTESIAN_POINT ( 'NONE',  ( 3.556970738554033499E-15, -38.81732327939057825, -2.124999997268813612 ) ) ;
#30101=CARTESIAN_POINT ( 'NONE',  ( 27.73933785331498925, -9.013057229001033122, 146.2750000027311899 ) ) ;
#30124=CARTESIAN_POINT ( 'NONE',  ( 23.31738231874054534, 16.94106989632529192, 145.4500000054623854 ) ) ;
#30213=CARTESIAN_POINT ( 'NONE',  ( 27.73933785331498569, 9.013057229001093518, 143.9750000027312069 ) ) ;
#30306=ORIENTED_EDGE ( 'NONE', *, *, #193551, .F. ) ;
#30340=CARTESIAN_POINT ( 'NONE',  ( -11.40812507854755609, 35.11059874428196537, -7.524999997268813523 ) ) ;
#30341=CARTESIAN_POINT ( 'NONE',  ( -34.11680238834244960, 4.370175642590067966, 91.64155955192003944 ) ) ;
#30343=CARTESIAN_POINT ( 'NONE',  ( 37.99626262588767389, -12.34573411038910251, -2.847842220587804007 ) ) ;
#30346=CARTESIAN_POINT ( 'NONE',  ( 33.85315667487626712, 0.3602237081833412069, 100.5000000000009948 ) ) ;
#30380=CARTESIAN_POINT ( 'NONE',  ( -31.72709406046301339, 2.040068635034919209E-14, 102.5000000000000142 ) ) ;
#30396=LINE ( 'NONE', #94042, #134214 ) ;
#30433=CARTESIAN_POINT ( 'NONE',  ( 28.82186960331498327, 2.781578969918950771E-14, 143.2500000054623683 ) ) ;
#30445=CARTESIAN_POINT ( 'NONE',  ( -32.33351994418283937, 3.967450966133711177, 88.63067128610950363 ) ) ;
#30528=CARTESIAN_POINT ( 'NONE',  ( -11.40812507854754720, -35.11059874428192273, -6.724999997268813701 ) ) ;
#30597=AXIS2_PLACEMENT_3D ( 'NONE', #53506, #132355, #55511 ) ;
#30621=CARTESIAN_POINT ( 'NONE',  ( -27.73933785331498925, -9.013057229001049109, 144.9750000027312069 ) ) ;
#30721=CARTESIAN_POINT ( 'NONE',  ( -8.906447517083053711, -27.41122689804191026, 144.6500000054623740 ) ) ;
#30791=CARTESIAN_POINT ( 'NONE',  ( 35.13534055906293929, 5.469967203781499698, 39.86293573631996878 ) ) ;
#30819=EDGE_CURVE ( 'NONE', #128112, #172412, #141459, .T. ) ;
#31052=DIRECTION ( 'NONE',  ( 0.000000000000000000, 0.000000000000000000, 1.000000000000000000 ) ) ;
#31068=CARTESIAN_POINT ( 'NONE',  ( -36.80065496640119704, -5.465942522010068139, 45.70922642070194541 ) ) ;
#31074=VECTOR ( 'NONE', #167212, 1000.000000000000000 ) ;
#31099=CARTESIAN_POINT ( 'NONE',  ( -22.44159573604009950, -16.30477369853688430, 145.5750000027311728 ) ) ;
#31123=CARTESIAN_POINT ( 'NONE',  ( -28.82186960331499392, -9.364793116373526516, 144.3500000054623627 ) ) ;
#31145=CARTESIAN_POINT ( 'NONE',  ( -37.99626262588769521, -12.34573411038907764, -7.647842220587804718 ) ) ;
#31159=EDGE_LOOP ( 'NONE', ( #100520, #49126, #110587, #197677 ) ) ;
#31210=CARTESIAN_POINT ( 'NONE',  ( -27.73933785331498925, 9.013057229001088189, 140.7750000027311899 ) ) ;
#31227=CARTESIAN_POINT ( 'NONE',  ( 37.99626262588765258, 2.893932880411085066E-14, -4.747842220587804363 ) ) ;
#31336=CARTESIAN_POINT ( 'NONE',  ( -29.86685920354755552, 21.69954338932564397, -0.8249999972688133454 ) ) ;
#31337=CARTESIAN_POINT ( 'NONE',  ( -34.16333257229422316, 4.138830072290156536, 91.36021987110632381 ) ) ;
#31339=CARTESIAN_POINT ( 'NONE',  ( -23.48298174826589602, -32.32155151706771790, -3.447842220587803652 ) ) ;
#31342=CARTESIAN_POINT ( 'NONE',  ( 33.70206089117255743, 4.379927107397421082, 98.34612363080974262 ) ) ;
#31354=CARTESIAN_POINT ( 'NONE',  ( 36.91746824999999177, 11.99521256947799230, -4.024999997268814411 ) ) ;
#31358=AXIS2_PLACEMENT_3D ( 'NONE', #125878, #27183, #63207 ) ;
#31381=SHAPE_REPRESENTATION ( 'Front Concentrator Nozzle', ( #82054 ), #62737 ) ;
#31396=ORIENTED_EDGE ( 'NONE', *, *, #43889, .T. ) ;
#31438=CARTESIAN_POINT ( 'NONE',  ( -32.64453336272028139, 0.4913919212617717247, 87.50000000000000000 ) ) ;
#31498=AXIS2_PLACEMENT_3D ( 'NONE', #158380, #145193, #187753 ) ;
#31524=CARTESIAN_POINT ( 'NONE',  ( 29.86685920354754487, 21.69954338932564752, -3.924999997268812990 ) ) ;
#31542=VERTEX_POINT ( 'NONE', #171926 ) ;
#31610=CARTESIAN_POINT ( 'NONE',  ( -36.87151287952131185, 2.273789158011777722, 50.01119746921813913 ) ) ;
#31616=CARTESIAN_POINT ( 'NONE',  ( -5.359611314223446995E-15, 29.16686587814335496, 144.3750000027311842 ) ) ;
#31630=EDGE_LOOP ( 'NONE', ( #177392, #24946 ) ) ;
#31712=CARTESIAN_POINT ( 'NONE',  ( -17.81289503416611097, -24.51734667627696496, 144.5500000054623513 ) ) ;
#31971=CARTESIAN_POINT ( 'NONE',  ( 22.81625015709509441, 31.40387420917330275, -1.324999997268813123 ) ) ;
#32016=CARTESIAN_POINT ( 'NONE',  ( 38.00000000000000711, -12.34694845685040754, -6.849999994537626868 ) ) ;
#32062=CARTESIAN_POINT ( 'NONE',  ( -36.99122028029232467, -5.215067209438918105, 43.21662174228439568 ) ) ;
#32092=CARTESIAN_POINT ( 'NONE',  ( 17.14385361876520264, -23.59649016807271238, 142.0750000027311444 ) ) ;
#32115=CARTESIAN_POINT ( 'NONE',  ( 17.81289503416611453, -24.51734667627695785, 140.6999999999999602 ) ) ;
#32116=CARTESIAN_POINT ( 'NONE',  ( 17.81289503416610742, 24.51734667627700404, 143.5500000054623513 ) ) ;
#32152=ORIENTED_EDGE ( 'NONE', *, *, #146342, .T. ) ;
#32179=CARTESIAN_POINT ( 'NONE',  ( -37.99626262588765968, 12.34573411038917179, -1.847842220587803341 ) ) ;
#32206=CARTESIAN_POINT ( 'NONE',  ( 27.73933785331498569, 9.013057229001093518, 145.9750000027311785 ) ) ;
#32262=ADVANCED_FACE ( 'NONE', ( #192072, #38394 ), #52550, .F. ) ;
#32333=CARTESIAN_POINT ( 'NONE',  ( -29.86685920354755552, 21.69954338932564397, -7.324999997268814234 ) ) ;
#32338=DIRECTION ( 'NONE',  ( 0.000000000000000000, 0.000000000000000000, 1.000000000000000000 ) ) ;
#32382=CARTESIAN_POINT ( 'NONE',  ( 34.67490716095262826, -3.335491994402099092, 51.73554620185606012 ) ) ;
#32387=DIRECTION ( 'NONE',  ( 1.000000000000000000, 0.000000000000000000, 0.000000000000000000 ) ) ;
#32434=CARTESIAN_POINT ( 'NONE',  ( -31.49214409296861916, 4.585214664522601069, 100.9553921309669562 ) ) ;
#32476=CARTESIAN_POINT ( 'NONE',  ( 37.99626262588765258, 2.893932880411085066E-14, -4.747842220587804363 ) ) ;
#32497=EDGE_CURVE ( 'NONE', #17723, #55000, #88682, .T. ) ;
#32521=CARTESIAN_POINT ( 'NONE',  ( 29.86685920354754487, 21.69954338932564752, -5.924999997268813878 ) ) ;
#32572=CARTESIAN_POINT ( 'NONE',  ( -28.82186960331494419, 9.364793116373629545, 146.1500000054623456 ) ) ;
#32574=LINE ( 'NONE', #83780, #150133 ) ;
#32604=CARTESIAN_POINT ( 'NONE',  ( -36.76795047837064345, 4.947931209100015160, 47.42876213711301858 ) ) ;
#32609=CARTESIAN_POINT ( 'NONE',  ( -27.73933785331498925, 2.428612866367529932E-14, 142.8750000027311842 ) ) ;
#32644=EDGE_LOOP ( 'NONE', ( #38049, #100008, #36115, #193625 ) ) ;
#32687=EDGE_CURVE ( 'NONE', #167889, #46374, #65274, .T. ) ;
#32708=DIRECTION ( 'NONE',  ( 0.000000000000000000, 0.000000000000000000, -1.000000000000000000 ) ) ;
#32723=CARTESIAN_POINT ( 'NONE',  ( -23.48529157249599919, -32.32473071737750558, -9.699999999999999289 ) ) ;
#32747=B_SPLINE_CURVE_WITH_KNOTS ( 'NONE', 3,
 ( #191459, #159116, #172313, #83274, #52937, #188490, #112621, #111633, #173318, #19627, #81269, #174313, #41793, #161125, #22621, #195485, #72120, #69114, #165139, #101439, #194477, #116623, #56960, #102456, #71124, #177319, #57958, #84268, #178312, #88273, #148970, #38790, #119629, #55949, #26630, #73138, #40787, #85271, #11467, #134808, #99445, #39775, #164144 ),
 .UNSPECIFIED., .F., .F.,
 ( 4, 2, 2, 2, 2, 2, 2, 2, 2, 2, 2, 2, 2, 1, 2, 2, 2, 2, 2, 2, 2, 4 ),
 ( 0.04122229388621103524, 0.04269295678691728546, 0.04416361968762353568, 0.04489895113797665732, 0.04563428258832977896, 0.04710494548903602918, 0.04857560838974227940, 0.04931093984009541492, 0.05004627129044855044, 0.05151693419115481454, 0.05298759709186107864, 0.05445825999256734273, 0.05519359144292046437, 0.05592892289327358601, 0.05666425434362670766, 0.05739958579397982930, 0.05887024869468609339, 0.06034091159539235749, 0.06181157449609861465, 0.06254690594645175017, 0.06328223739680488569, 0.06475290029751114285 ),
 .UNSPECIFIED. ) ;
#32774=ORIENTED_EDGE ( 'NONE', *, *, #4359, .T. ) ;
#32933=CARTESIAN_POINT ( 'NONE',  ( 34.16298174666832921, -4.140866818352566092, 91.36220571553955949 ) ) ;
#32968=CARTESIAN_POINT ( 'NONE',  ( 29.86685920354754487, 21.69954338932564752, -1.424999997268813212 ) ) ;
#33012=ORIENTED_EDGE ( 'NONE', *, *, #73347, .F. ) ;
#33057=CARTESIAN_POINT ( 'NONE',  ( -37.42090987696013116, -2.907880681671515255, 40.32815749938560401 ) ) ;
#33086=CARTESIAN_POINT ( 'NONE',  ( -28.82186960331499037, 2.428612866367529932E-14, 146.0000000000000000 ) ) ;
#33110=CARTESIAN_POINT ( 'NONE',  ( -35.31606782002515388, 4.574060259307354492, 39.03637847775443248 ) ) ;
#33122=VERTEX_POINT ( 'NONE', #10067 ) ;
#33197=EDGE_CURVE ( 'NONE', #26356, #60581, #7982, .T. ) ;
#33202=CARTESIAN_POINT ( 'NONE',  ( 27.73933785331498925, -9.013057229001034898, 145.7750000027311899 ) ) ;
#33276=CARTESIAN_POINT ( 'NONE',  ( 37.99626262588765258, 2.893932880411085066E-14, -7.002157773949822861 ) ) ;
#33323=CARTESIAN_POINT ( 'NONE',  ( -22.81625015709510507, 31.40387420917330275, -4.924999997268813878 ) ) ;
#33341=CARTESIAN_POINT ( 'NONE',  ( 34.12434206616184440, 14.08647367304311260, -8.000000000000001776 ) ) ;
#33375=CARTESIAN_POINT ( 'NONE',  ( 30.00000000000000711, -5.510910596163089556E-15, 45.00000000000000000 ) ) ;
#33404=AXIS2_PLACEMENT_3D ( 'NONE', #193592, #195601, #116735 ) ;
#33407=CARTESIAN_POINT ( 'NONE',  ( 23.31738231874054534, 16.94106989632529192, 141.1999999999999886 ) ) ;
#33509=CARTESIAN_POINT ( 'NONE',  ( -37.99626262588762415, -12.34573411038919311, -5.902157773949822328 ) ) ;
#33512=CARTESIAN_POINT ( 'NONE',  ( 22.81625015709509441, 31.40387420917330275, -3.824999997268813345 ) ) ;
#33574=CARTESIAN_POINT ( 'NONE',  ( 37.99626262588765258, 2.893932880411085066E-14, -7.002157773949822861 ) ) ;
#33592=ORIENTED_EDGE ( 'NONE', *, *, #152340, .F. ) ;
#33599=CARTESIAN_POINT ( 'NONE',  ( -27.73933785331498925, 2.428612866367529932E-14, 140.8750000027311842 ) ) ;
#33603=CARTESIAN_POINT ( 'NONE',  ( -8.571926809382608425, 26.38167802310805854, 140.4750000027312069 ) ) ;
#33633=ORIENTED_EDGE ( 'NONE', *, *, #142366, .F. ) ;
#33669=CARTESIAN_POINT ( 'NONE',  ( -8.571926809382608425, 26.38167802310805854, 146.9750000027311785 ) ) ;
#33715=CARTESIAN_POINT ( 'NONE',  ( -17.81289503416611808, 24.51734667627700404, 147.6999999999999886 ) ) ;
#33717=DIRECTION ( 'NONE',  ( -1.000000000000000000, 0.000000000000000000, -3.709348145883536076E-20 ) ) ;
#33725=AXIS2_PLACEMENT_3D ( 'NONE', #53782, #193304, #175130 ) ;
#33834=CARTESIAN_POINT ( 'NONE',  ( -11.40812507854755609, 35.11059874428196537, -5.024999997268813523 ) ) ;
#33851=ORIENTED_EDGE ( 'NONE', *, *, #198419, .F. ) ;
#33906=DIRECTION ( 'NONE',  ( 0.000000000000000000, 0.000000000000000000, -1.000000000000000000 ) ) ;
#33914=DIRECTION ( 'NONE',  ( 1.000000000000000000, 0.000000000000000000, 0.000000000000000000 ) ) ;
#33957=CARTESIAN_POINT ( 'NONE',  ( 11.40812507854754365, 35.11059874428196537, -5.224999997268813701 ) ) ;
#34002=ORIENTED_EDGE ( 'NONE', *, *, #16626, .F. ) ;
#34048=CARTESIAN_POINT ( 'NONE',  ( -11.74149087413295511, 36.13659316521247433, -6.147842220587803830 ) ) ;
#34078=CARTESIAN_POINT ( 'NONE',  ( 22.44159573604009239, 16.30477369853692693, 140.5750000027311728 ) ) ;
#34101=VECTOR ( 'NONE', #166044, 1000.000000000000114 ) ;
#34103=CARTESIAN_POINT ( 'NONE',  ( -17.81289503416611808, 24.51734667627700404, 141.9500000054623285 ) ) ;
#34109=DIRECTION ( 'NONE',  ( -1.000000000000000000, -0.000000000000000000, -0.000000000000000000 ) ) ;
#34112=CARTESIAN_POINT ( 'NONE',  ( 31.99364916731006048, 4.791014396527177230E-13, 45.00000000000022027 ) ) ;
#34164=CARTESIAN_POINT ( 'NONE',  ( -30.73962218707678318, 22.33364281372846705, -1.947842220587803874 ) ) ;
#34192=CARTESIAN_POINT ( 'NONE',  ( -22.44159573604010305, 16.30477369853692338, 142.6750000027311671 ) ) ;
#34272=CYLINDRICAL_SURFACE ( 'NONE', #120879, 5.500000000001017852 ) ;
#34315=CARTESIAN_POINT ( 'NONE',  ( 3.556970738554033499E-15, -38.81732327939057825, -6.124999997268812280 ) ) ;
#34370=CARTESIAN_POINT ( 'NONE',  ( 35.02204707441116227, -5.958053119633049732, 40.41886734368968348 ) ) ;
#34507=CARTESIAN_POINT ( 'NONE',  ( 22.81625015709509441, 31.40387420917330275, -9.824999997268811569 ) ) ;
#34556=CARTESIAN_POINT ( 'NONE',  ( 12.78135187869861511, -34.69226357686214612, -8.000000000000003553 ) ) ;
#34592=CARTESIAN_POINT ( 'NONE',  ( -8.571926809382608425, 26.38167802310805854, 142.4750000027312069 ) ) ;
#34625=EDGE_LOOP ( 'NONE', ( #118427, #64920, #137199, #118377 ) ) ;
#34628=VERTEX_POINT ( 'NONE', #169215 ) ;
#34663=CARTESIAN_POINT ( 'NONE',  ( -17.14385361876520264, -23.59649016807271238, 145.6750000027311671 ) ) ;
#34793=CARTESIAN_POINT ( 'NONE',  ( -27.73933785331498925, 2.428612866367529932E-14, 148.8750000027311842 ) ) ;
#34823=CARTESIAN_POINT ( 'NONE',  ( -22.81625015709510507, 31.40387420917330275, -0.9249999972688132122 ) ) ;
#34899=DIRECTION ( 'NONE',  ( -7.855351589328939542E-15, 0.000000000000000000, 1.000000000000000000 ) ) ;
#34922=( BOUNDED_CURVE ( )  B_SPLINE_CURVE ( 2, ( #103575, #149083, #74233, #10571, #88382, #59040, #57074, #168210, #13541, #48846, #139837 ),
 .UNSPECIFIED., .F., .T. ) 
 B_SPLINE_CURVE_WITH_KNOTS ( ( 3, 2, 2, 2, 2, 3 ),
 ( 0.3000000000000002665, 0.3200000000000002842, 0.3400000000000003020, 0.3600000000000003197, 0.3800000000000003375, 0.4000000000000003553 ),
 .UNSPECIFIED. ) 
 CURVE ( )  GEOMETRIC_REPRESENTATION_ITEM ( )  RATIONAL_B_SPLINE_CURVE ( ( 0.9999999999999993339, 0.9510565162951541973, 1.000000000000000000, 0.9510565162951535312, 1.000000000000000000, 0.9510565162951535312, 1.000000000000000000, 0.9510565162951535312, 1.000000000000000000, 0.9510565162951527540, 1.000000000000000888 ) ) 
 REPRESENTATION_ITEM ( '' )  );
#34927=AXIS2_PLACEMENT_3D ( 'NONE', #22358, #98161, #35524 ) ;
#34946=CARTESIAN_POINT ( 'NONE',  ( -30.74264578624800492, 22.33583958711400186, -0.1999999999999999001 ) ) ;
#35034=CARTESIAN_POINT ( 'NONE',  ( 31.25074303019345479, -7.456059982492100779, 95.94898436327792979 ) ) ;
#35063=CARTESIAN_POINT ( 'NONE',  ( 23.31738231874054890, -16.94106989632523508, 146.7999999999999829 ) ) ;
#35086=CARTESIAN_POINT ( 'NONE',  ( -17.81289503416611808, 24.51734667627700404, 139.9500000054623285 ) ) ;
#35122=ORIENTED_EDGE ( 'NONE', *, *, #41647, .F. ) ;
#35157=ADVANCED_BREP_SHAPE_REPRESENTATION ( '', ( #142731, #82054 ), #62737 ) ;
#35180=CARTESIAN_POINT ( 'NONE',  ( 8.571926809382597767, 26.38167802310806209, 140.2750000027311899 ) ) ;
#35258=FACE_OUTER_BOUND ( 'NONE', #47494, .T. ) ;
#35302=CARTESIAN_POINT ( 'NONE',  ( 36.91746825000000598, -11.99521256947793546, -7.724999997268812812 ) ) ;
#35359=CARTESIAN_POINT ( 'NONE',  ( 34.40547513665162427, -6.508760260264946140, 48.73452191691476543 ) ) ;
#35432=AXIS2_PLACEMENT_3D ( 'NONE', #45867, #43891, #60038 ) ;
#35496=CYLINDRICAL_SURFACE ( 'NONE', #179082, 28.82186960331498682 ) ;
#35524=DIRECTION ( 'NONE',  ( 1.000000000000000000, 0.000000000000000000, 0.000000000000000000 ) ) ;
#35583=CARTESIAN_POINT ( 'NONE',  ( 22.44159573604009594, -16.30477369853687364, 141.6750000027311671 ) ) ;
#35607=AXIS2_PLACEMENT_3D ( 'NONE', #60057, #182431, #32708 ) ;
#35653=CARTESIAN_POINT ( 'NONE',  ( 27.73933785331498569, 2.768321779492822058E-14, 146.3750000027311842 ) ) ;
#35731=CARTESIAN_POINT ( 'NONE',  ( 23.48529157249599919, 32.32473071737754111, -2.449999994537626069 ) ) ;
#35741=( BOUNDED_CURVE ( )  B_SPLINE_CURVE ( 2, ( #76211, #109533, #186403, #137890, #141853, #47880, #30721, #31712, #356, #92368, #95352 ),
 .UNSPECIFIED., .F., .T. ) 
 B_SPLINE_CURVE_WITH_KNOTS ( ( 3, 2, 2, 2, 2, 3 ),
 ( 0.3000000000000002665, 0.3200000000000002842, 0.3400000000000003020, 0.3600000000000003197, 0.3800000000000003375, 0.4000000000000003553 ),
 .UNSPECIFIED. ) 
 CURVE ( )  GEOMETRIC_REPRESENTATION_ITEM ( )  RATIONAL_B_SPLINE_CURVE ( ( 0.9999999999999993339, 0.9510565162951541973, 1.000000000000000000, 0.9510565162951535312, 1.000000000000000000, 0.9510565162951535312, 1.000000000000000000, 0.9510565162951535312, 1.000000000000000000, 0.9510565162951527540, 1.000000000000000888 ) ) 
 REPRESENTATION_ITEM ( '' )  );
#35744=ORIENTED_EDGE ( 'NONE', *, *, #76080, .F. ) ;
#35779=CARTESIAN_POINT ( 'NONE',  ( 37.01127658466556625, 5.144934411046667044, 43.04759647146322266 ) ) ;
#35781=CARTESIAN_POINT ( 'NONE',  ( -11.40812507854755609, 35.11059874428196537, -3.524999997268813523 ) ) ;
#35813=CARTESIAN_POINT ( 'NONE',  ( 22.81625015709509441, 31.40387420917330275, -5.324999997268813345 ) ) ;
#35932=CARTESIAN_POINT ( 'NONE',  ( -29.86685920354755197, -21.69954338932560134, -6.424999997268812990 ) ) ;
#36039=VERTEX_POINT ( 'NONE', #177210 ) ;
#36051=CARTESIAN_POINT ( 'NONE',  ( -8.906447517083053711, -27.41122689804191026, 146.4000000000000057 ) ) ;
#36073=CARTESIAN_POINT ( 'NONE',  ( -23.31738231874055600, 16.94106989632528837, 140.0500000054623513 ) ) ;
#36115=ORIENTED_EDGE ( 'NONE', *, *, #176051, .T. ) ;
#36176=DIRECTION ( 'NONE',  ( -0.06104853953485701173, -7.476289853398329258E-18, -0.9981347984218670311 ) ) ;
#36178=CARTESIAN_POINT ( 'NONE',  ( 28.82186960331498327, 2.781578969918950771E-14, 149.0000000000000000 ) ) ;
#36181=CARTESIAN_POINT ( 'NONE',  ( 36.81601778013476434, -3.637449627666672569, 49.14141020753752542 ) ) ;
#36223=ADVANCED_FACE ( 'NONE', ( #101330 ), #164037, .F. ) ;
#36281=CARTESIAN_POINT ( 'NONE',  ( 36.91746825000000598, -11.99521256947793546, -3.724999997268812812 ) ) ;
#36282=CARTESIAN_POINT ( 'NONE',  ( -33.70615967800006985, 5.466638699193796747, 95.70352821367444562 ) ) ;
#36338=CARTESIAN_POINT ( 'NONE',  ( 34.64437015671236963, -3.766696895669991552, 51.50405731776599083 ) ) ;
#36361=CARTESIAN_POINT ( 'NONE',  ( -11.74149087413295511, 36.13659316521247433, -4.402157773949823216 ) ) ;
#36566=CARTESIAN_POINT ( 'NONE',  ( -17.14385361876520264, -23.59649016807271593, 147.6750000027311671 ) ) ;
#36637=CARTESIAN_POINT ( 'NONE',  ( 27.73933785331498569, 2.768321779492822058E-14, 148.3750000027311842 ) ) ;
#36714=CARTESIAN_POINT ( 'NONE',  ( -30.74264578624800492, 22.33583958711400186, -1.949999994537626735 ) ) ;
#36736=ORIENTED_EDGE ( 'NONE', *, *, #81855, .T. ) ;
#36766=CARTESIAN_POINT ( 'NONE',  ( 22.81625015709510151, -31.40387420917324590, -6.424999997268812102 ) ) ;
#36793=EDGE_CURVE ( 'NONE', #180473, #175318, #20372, .T. ) ;
#36799=CARTESIAN_POINT ( 'NONE',  ( -36.91746825000000598, 11.99521256947798520, -4.724999997268811924 ) ) ;
#36843=AXIS2_PLACEMENT_3D ( 'NONE', #26739, #148076, #41904 ) ;
#36884=CARTESIAN_POINT ( 'NONE',  ( -32.00000000000000000, -5.510910596163089556E-15, 39.49999999999996447 ) ) ;
#36924=CARTESIAN_POINT ( 'NONE',  ( -22.81625015709509441, -31.40387420917324590, -8.324999997268815122 ) ) ;
#37040=DIRECTION ( 'NONE',  ( 0.8660254037844392627, 0.000000000000000000, 0.4999999999999988898 ) ) ;
#37050=CARTESIAN_POINT ( 'NONE',  ( -5.359611314223446995E-15, 29.16686587814335496, 140.8750000027311842 ) ) ;
#37072=CARTESIAN_POINT ( 'NONE',  ( 8.906447517083057264, -27.41122689804191026, 140.8500000054623911 ) ) ;
#37079=CARTESIAN_POINT ( 'NONE',  ( 35.99626262588764547, 2.869439944428138037E-14, 2.000000000000000000 ) ) ;
#37139=AXIS2_PLACEMENT_3D ( 'NONE', #40384, #163743, #34899 ) ;
#37154=AXIS2_PLACEMENT_3D ( 'NONE', #73026, #86176, #23514 ) ;
#37171=AXIS2_PLACEMENT_3D ( 'NONE', #50464, #191948, #82760 ) ;
#37182=DIRECTION ( 'NONE',  ( -1.000000000000000000, -0.000000000000000000, -0.000000000000000000 ) ) ;
#37288=CARTESIAN_POINT ( 'NONE',  ( 11.40812507854754365, 35.11059874428196537, -7.224999997268813701 ) ) ;
#37344=CARTESIAN_POINT ( 'NONE',  ( -27.73933785331498925, 2.428612866367529932E-14, 139.3750000027311842 ) ) ;
#37423=FACE_OUTER_BOUND ( 'NONE', #483, .T. ) ;
#37503=EDGE_LOOP ( 'NONE', ( #80250, #39779, #2613, #55497 ) ) ;
#37533=DIRECTION ( 'NONE',  ( 0.000000000000000000, 0.000000000000000000, -1.000000000000000000 ) ) ;
#37575=CARTESIAN_POINT ( 'NONE',  ( 27.73933785331498214, 9.013057229001095294, 144.4750000027311501 ) ) ;
#37579=CARTESIAN_POINT ( 'NONE',  ( -37.99626262588766679, 2.428612866367529932E-14, -0.002157773949821304490 ) ) ;
#37608=ADVANCED_FACE ( 'NONE', ( #175744 ), #146388, .F. ) ;
#37649=CARTESIAN_POINT ( 'NONE',  ( 22.44159573604009239, 16.30477369853692693, 146.5750000027312012 ) ) ;
#37728=CARTESIAN_POINT ( 'NONE',  ( -30.74264578624800492, -22.33583958711396278, -3.549999994537626602 ) ) ;
#37741=ORIENTED_EDGE ( 'NONE', *, *, #177539, .F. ) ;
#37764=CARTESIAN_POINT ( 'NONE',  ( 31.37858599332833620, 5.662547894918608549, 99.94225302722350079 ) ) ;
#37779=CARTESIAN_POINT ( 'NONE',  ( 36.91746824999999887, 11.99521256947799053, -4.024999997268814411 ) ) ;
#37808=CARTESIAN_POINT ( 'NONE',  ( -38.00373040315628970, 1.963201398428686990E-14, -0.1220970790697140096 ) ) ;
#37813=CARTESIAN_POINT ( 'NONE',  ( 29.86685920354754487, 21.69954338932564752, -3.424999997268813434 ) ) ;
#37936=CARTESIAN_POINT ( 'NONE',  ( -29.86685920354755197, -21.69954338932560134, -10.42499999726881299 ) ) ;
#37951=EDGE_CURVE ( 'NONE', #58436, #150593, #179764, .T. ) ;
#38003=VERTEX_POINT ( 'NONE', #186630 ) ;
#38049=ORIENTED_EDGE ( 'NONE', *, *, #142366, .T. ) ;
#38060=CARTESIAN_POINT ( 'NONE',  ( 17.81289503416611453, -24.51734667627695785, 144.6999999999999886 ) ) ;
#38083=CARTESIAN_POINT ( 'NONE',  ( -27.73933785331498925, 2.428612866367529932E-14, 144.8750000027311842 ) ) ;
#38178=CARTESIAN_POINT ( 'NONE',  ( -27.73933785331498925, 2.428612866367529932E-14, 138.8750000027311842 ) ) ;
#38195=LINE ( 'NONE', #6838, #141830 ) ;
#38295=CARTESIAN_POINT ( 'NONE',  ( 22.81625015709509441, 31.40387420917330275, -9.324999997268813345 ) ) ;
#38394=FACE_BOUND ( 'NONE', #130095, .T. ) ;
#38501=CARTESIAN_POINT ( 'NONE',  ( 35.03251413515944535, -11.89243146578850130, -8.000000000000001776 ) ) ;
#38548=CARTESIAN_POINT ( 'NONE',  ( -33.84943726220063098, -0.7253354391803957801, 100.4638154892406021 ) ) ;
#38586=CARTESIAN_POINT ( 'NONE',  ( -27.73933785331498925, 9.013057229001089965, 141.2750000027311614 ) ) ;
#38617=ADVANCED_FACE ( 'NONE', ( #52062, #98549 ), #69229, .F. ) ;
#38661=CARTESIAN_POINT ( 'NONE',  ( -8.571926809382601320, -26.38167802310801591, 139.7750000027311899 ) ) ;
#38737=CARTESIAN_POINT ( 'NONE',  ( 38.00000000000000711, -12.34694845685040754, -4.849999994537625092 ) ) ;
#38747=FACE_BOUND ( 'NONE', #124199, .T. ) ;
#38774=CARTESIAN_POINT ( 'NONE',  ( 31.23840969660177436, 7.314650797970924323, 96.67552899226035379 ) ) ;
#38790=CARTESIAN_POINT ( 'NONE',  ( -34.48175918554795771, -5.660046887242175195, 49.94512835368022508 ) ) ;
#38813=FACE_OUTER_BOUND ( 'NONE', #134527, .T. ) ;
#38938=CARTESIAN_POINT ( 'NONE',  ( -36.91746825000000598, 2.428612866367529932E-14, -8.624999997268814056 ) ) ;
#39120=EDGE_CURVE ( 'NONE', #31542, #82818, #43493, .T. ) ;
#39121=ORIENTED_EDGE ( 'NONE', *, *, #68419, .T. ) ;
#39187=CARTESIAN_POINT ( 'NONE',  ( 36.85371136276476278, -2.758154363750434879, 49.76185830465986015 ) ) ;
#39260=CARTESIAN_POINT ( 'NONE',  ( -13.79161361927567597, 35.19715793953689342, -8.000000000000000000 ) ) ;
#39290=CARTESIAN_POINT ( 'NONE',  ( -22.44159573604009950, -16.30477369853688430, 147.5750000027312012 ) ) ;
#39318=EDGE_CURVE ( 'NONE', #17723, #168659, #164256, .T. ) ;
#39334=DIRECTION ( 'NONE',  ( 0.000000000000000000, 0.000000000000000000, -1.000000000000000000 ) ) ;
#39351=B_SPLINE_CURVE_WITH_KNOTS ( 'NONE', 3,
 ( #12659, #197664, #105639, #123762, #138945, #170288, #61110, #1420, #13631, #44970, #59130, #60125, #93431, #74326, #120797, #151171, #119826, #181511, #43977, #75298, #42990, #167328, #28824, #78258, #122783, #136969, #104655, #184473, #121792, #198658, #183486, #77276, #27839, #91434, #30791, #106628, #29798, #107607, #168302, #169285, #92439, #154125, #185461, #425, #62099, #46951, #89480, #67078 ),
 .UNSPECIFIED., .F., .F.,
 ( 4, 2, 2, 2, 2, 2, 2, 2, 2, 2, 2, 2, 2, 2, 2, 2, 2, 2, 2, 2, 2, 2, 2, 4 ),
 ( 0.01768515071410577122, 0.01915622216236236713, 0.01989175788649066162, 0.02062729361061895611, 0.02209836505887554162, 0.02283390078300383264, 0.02356943650713212365, 0.02504050795538871610, 0.02651157940364531201, 0.02724711512777359956, 0.02798265085190188711, 0.02945372230015844486, 0.03092479374841500261, 0.03239586519667155690, 0.03313140092079984445, 0.03386693664492812506, 0.03460247236905640567, 0.03533800809318470015, 0.03680907954144128219, 0.03754461526556956974, 0.03828015098969785729, 0.03975122243795443933, 0.04048675816208271994, 0.04122229388621100749 ),
 .UNSPECIFIED. ) ;
#39501=ORIENTED_EDGE ( 'NONE', *, *, #176156, .F. ) ;
#39535=CARTESIAN_POINT ( 'NONE',  ( -34.42160027699925706, -2.272024392515961555, 89.98798656105711302 ) ) ;
#39536=CARTESIAN_POINT ( 'NONE',  ( -36.91746825000000598, 2.428612866367529932E-14, -0.8749999972688132788 ) ) ;
#39551=ORIENTED_EDGE ( 'NONE', *, *, #23933, .T. ) ;
#39571=CARTESIAN_POINT ( 'NONE',  ( -31.79921067246706201, -6.362367971534558464, 91.02144216243111430 ) ) ;
#39575=CARTESIAN_POINT ( 'NONE',  ( 8.571926809382597767, 26.38167802310806209, 144.7750000027311899 ) ) ;
#39649=CARTESIAN_POINT ( 'NONE',  ( -8.571926809382601320, -26.38167802310801591, 141.7750000027311899 ) ) ;
#39721=CARTESIAN_POINT ( 'NONE',  ( 11.74264578624800315, -36.14014761921581709, -11.14999999453762669 ) ) ;
#39759=CARTESIAN_POINT ( 'NONE',  ( 31.49214409296861206, 4.585214664522583305, 100.9553921309669704 ) ) ;
#39772=CARTESIAN_POINT ( 'NONE',  ( 36.93866063236283281, 5.356020730800094221, 43.73704834337281966 ) ) ;
#39775=CARTESIAN_POINT ( 'NONE',  ( -34.78522506798721992, -0.4968532545621949237, 52.49999999999998579 ) ) ;
#39779=ORIENTED_EDGE ( 'NONE', *, *, #124331, .T. ) ;
#39790=ADVANCED_FACE ( 'NONE', ( #115628 ), #82108, .T. ) ;
#39818=ORIENTED_EDGE ( 'NONE', *, *, #39120, .F. ) ;
#39820=CYLINDRICAL_SURFACE ( 'NONE', #25126, 5.500000000001017852 ) ;
#39887=DIRECTION ( 'NONE',  ( -3.709348145883536076E-20, 0.000000000000000000, 1.000000000000000000 ) ) ;
#39930=CARTESIAN_POINT ( 'NONE',  ( 30.74264578624800137, -22.33583958711395212, -1.200000000000000178 ) ) ;
#40008=DIRECTION ( 'NONE',  ( -0.000000000000000000, -0.000000000000000000, 1.000000000000000000 ) ) ;
#40047=CARTESIAN_POINT ( 'NONE',  ( -28.82186960331499037, 2.428612866367529932E-14, 142.0000000000000000 ) ) ;
#40149=AXIS2_PLACEMENT_3D ( 'NONE', #159113, #117623, #100445 ) ;
#40241=CARTESIAN_POINT ( 'NONE',  ( 23.31738231874054534, 16.94106989632529192, 145.1999999999999886 ) ) ;
#40259=CARTESIAN_POINT ( 'NONE',  ( 34.12434206616184440, 14.08647367304311260, -8.000000000000001776 ) ) ;
#40262=CARTESIAN_POINT ( 'NONE',  ( 23.31738231874054890, -16.94106989632523508, 141.0500000054623513 ) ) ;
#40331=EDGE_CURVE ( 'NONE', #83841, #177652, #130777, .T. ) ;
#40384=CARTESIAN_POINT ( 'NONE',  ( 31.99364916730971231, 1.011436372600181938E-12, 95.00000000000021316 ) ) ;
#40426=CARTESIAN_POINT ( 'NONE',  ( 23.48298174826589246, 32.32155151706776053, -2.702157773949822595 ) ) ;
#40457=VECTOR ( 'NONE', #87244, 1000.000000000000000 ) ;
#40510=ORIENTED_EDGE ( 'NONE', *, *, #121415, .F. ) ;
#40549=CARTESIAN_POINT ( 'NONE',  ( -37.07204608585244188, -7.847727336691864508, -7.999999999999996447 ) ) ;
#40561=CARTESIAN_POINT ( 'NONE',  ( -22.81625015709509441, -31.40387420917324590, -2.824999997268812901 ) ) ;
#40586=CARTESIAN_POINT ( 'NONE',  ( -27.73933785331498925, 9.013057229001089965, 145.2750000027311899 ) ) ;
#40606=CIRCLE ( 'NONE', #150454, 0.2000000000000057288 ) ;
#40659=CARTESIAN_POINT ( 'NONE',  ( -17.14385361876520264, -23.59649016807271238, 139.6750000027311955 ) ) ;
#40733=CARTESIAN_POINT ( 'NONE',  ( -11.74264578624799782, -36.14014761921581709, -11.34999999453762776 ) ) ;
#40770=CARTESIAN_POINT ( 'NONE',  ( 31.56642711641980625, 3.769985069463992478, 101.5021612967808409 ) ) ;
#40777=CARTESIAN_POINT ( 'NONE',  ( 31.68593437162162019, -6.718755962661552950, 91.65819149638747376 ) ) ;
#40784=CARTESIAN_POINT ( 'NONE',  ( 36.87151287952131185, 2.273789158011782163, 50.01119746921813913 ) ) ;
#40787=CARTESIAN_POINT ( 'NONE',  ( -34.71415419550760362, -2.652640888949080455, 52.01956328305328014 ) ) ;
#40802=EDGE_LOOP ( 'NONE', ( #123635, #84527 ) ) ;
#40815=CARTESIAN_POINT ( 'NONE',  ( 36.91746824999999177, 11.99521256947799230, -7.524999997268813523 ) ) ;
#40894=PLANE ( 'NONE',  #36843 ) ;
#40941=CARTESIAN_POINT ( 'NONE',  ( 11.74264578624800315, -36.14014761921581709, -5.400000000000000355 ) ) ;
#40971=EDGE_CURVE ( 'NONE', #49688, #200018, #175533, .T. ) ;
#41065=CARTESIAN_POINT ( 'NONE',  ( -17.81289503416611808, 24.51734667627700404, 143.7000000000000171 ) ) ;
#41197=CARTESIAN_POINT ( 'NONE',  ( 37.19790397533368775, -4.369830079088518282, 41.64077531718624670 ) ) ;
#41268=CARTESIAN_POINT ( 'NONE',  ( -18.63871995876255383, 32.95139847355620333, -7.999999999999996447 ) ) ;
#41300=CARTESIAN_POINT ( 'NONE',  ( 28.82186960331498327, 2.781578969918950771E-14, 145.2500000054623683 ) ) ;
#41323=CARTESIAN_POINT ( 'NONE',  ( -34.48171762721880640, 5.660481407866293502, 49.94458042978408940 ) ) ;
#41548=CARTESIAN_POINT ( 'NONE',  ( -11.40812507854754720, -35.11059874428192273, -2.724999997268813257 ) ) ;
#41567=CARTESIAN_POINT ( 'NONE',  ( 36.91746824999999887, -11.99521256947793546, -2.224999997268813701 ) ) ;
#41589=CARTESIAN_POINT ( 'NONE',  ( -31.34418352700887311, -5.970234417100033220, 99.56646813413776442 ) ) ;
#41593=CARTESIAN_POINT ( 'NONE',  ( 27.73933785331498569, 2.768321779492822058E-14, 146.3750000027311842 ) ) ;
#41605=ORIENTED_EDGE ( 'NONE', *, *, #115308, .T. ) ;
#41626=CARTESIAN_POINT ( 'NONE',  ( 8.906447517083050158, 27.41122689804195645, 139.6500000054623740 ) ) ;
#41639=CARTESIAN_POINT ( 'NONE',  ( 17.81289503416611453, -24.51734667627695785, 142.9500000054624138 ) ) ;
#41647=EDGE_CURVE ( 'NONE', #99233, #122084, #181060, .T. ) ;
#41664=EDGE_LOOP ( 'NONE', ( #143970, #36736, #164631, #100931, #160815 ) ) ;
#41740=CARTESIAN_POINT ( 'NONE',  ( -11.40812507854754720, -35.11059874428192273, -2.724999997268813257 ) ) ;
#41780=ORIENTED_EDGE ( 'NONE', *, *, #16626, .T. ) ;
#41793=CARTESIAN_POINT ( 'NONE',  ( -35.02204707441116938, -5.958053119633060390, 40.41886734368969059 ) ) ;
#41822=CARTESIAN_POINT ( 'NONE',  ( -37.51279278323693234, 1.941191203875217264, 39.85083793614485614 ) ) ;
#41833=CARTESIAN_POINT ( 'NONE',  ( -5.359611314223446995E-15, 29.16686587814335496, 144.3750000027311842 ) ) ;
#41837=ORIENTED_EDGE ( 'NONE', *, *, #61842, .F. ) ;
#41904=DIRECTION ( 'NONE',  ( 1.000000000000000000, 0.000000000000000000, -0.000000000000000000 ) ) ;
#41908=CARTESIAN_POINT ( 'NONE',  ( -31.28760401664904833, 6.510460035718205418, 98.73157056914054408 ) ) ;
#41934=CARTESIAN_POINT ( 'NONE',  ( -31.99364916731038022, -1.163414459189985801E-14, 95.00000000000000000 ) ) ;
#41950=CARTESIAN_POINT ( 'NONE',  ( -23.48529157249600985, 32.32473071737754111, -4.299999999999999822 ) ) ;
#41953=CARTESIAN_POINT ( 'NONE',  ( -30.00000000000000000, -1.163414459189985801E-14, 97.65000000000000568 ) ) ;
#41956=DIRECTION ( 'NONE',  ( 0.000000000000000000, -1.224646799151876092E-16, 1.000000000000000000 ) ) ;
#42236=CARTESIAN_POINT ( 'NONE',  ( -40.00000000000002842, 1.938754146708588393E-14, 0.000000000000000000 ) ) ;
#42273=CARTESIAN_POINT ( 'NONE',  ( 27.87032660475913204, 24.53198321425060158, -8.000000000000003553 ) ) ;
#42276=CARTESIAN_POINT ( 'NONE',  ( 28.82186960331498327, 2.781578969918950771E-14, 141.2500000054623683 ) ) ;
#42307=CARTESIAN_POINT ( 'NONE',  ( -40.00200000000003087, -1.163414459189985801E-14, 95.00000000000000000 ) ) ;
#42414=ORIENTED_EDGE ( 'NONE', *, *, #156518, .T. ) ;
#42542=CARTESIAN_POINT ( 'NONE',  ( 3.556970738554033499E-15, -38.81732327939057825, -4.624999997268814056 ) ) ;
#42549=CARTESIAN_POINT ( 'NONE',  ( -15.54838543842805443, -33.98976552189215283, -7.999999999999996447 ) ) ;
#42559=LINE ( 'NONE', #104222, #169681 ) ;
#42582=CARTESIAN_POINT ( 'NONE',  ( -31.76083434626056956, -6.487688756757402864, 91.22915654580295097 ) ) ;
#42663=DIRECTION ( 'NONE',  ( 0.000000000000000000, -1.224646799146988112E-16, 1.000000000000000000 ) ) ;
#42699=CARTESIAN_POINT ( 'NONE',  ( 30.00000000000000000, -5.510910596163089556E-15, 45.00000000000000000 ) ) ;
#42735=CARTESIAN_POINT ( 'NONE',  ( 37.99999999999999289, 2.893978650043524126E-14, -8.749999994537628112 ) ) ;
#42787=CARTESIAN_POINT ( 'NONE',  ( 36.79349492566039714, 4.147684444183153296, 48.62988885745598111 ) ) ;
#42819=CARTESIAN_POINT ( 'NONE',  ( -36.81781682666242972, 5.501098665926424935, 45.34601664933740039 ) ) ;
#42825=CARTESIAN_POINT ( 'NONE',  ( 17.14385361876520264, 23.59649016807275856, 148.1750000027311955 ) ) ;
#42830=CARTESIAN_POINT ( 'NONE',  ( 8.571926809382603096, -26.38167802310801235, 143.4750000027312069 ) ) ;
#42835=CARTESIAN_POINT ( 'NONE',  ( -28.82186960331499037, 2.428612866367529932E-14, 139.1250000027311842 ) ) ;
#42874=DIRECTION ( 'NONE',  ( 1.000000000000000000, 0.000000000000000000, 0.000000000000000000 ) ) ;
#42939=CARTESIAN_POINT ( 'NONE',  ( -30.74264578624800492, -22.33583958711396278, -1.800000000000000044 ) ) ;
#42990=CARTESIAN_POINT ( 'NONE',  ( 34.37178856895486234, 7.314363934749350094, 46.67665261413966959 ) ) ;
#43109=CARTESIAN_POINT ( 'NONE',  ( 37.99626262588764547, 12.34573411038917357, -0.9021577739498228832 ) ) ;
#43259=CARTESIAN_POINT ( 'NONE',  ( -3.573655867282028392E-15, 2.428612866367529932E-14, -8.000000000000000000 ) ) ;
#43285=CARTESIAN_POINT ( 'NONE',  ( -5.359611314223446995E-15, 29.16686587814335496, 142.8750000027311842 ) ) ;
#43293=DIRECTION ( 'NONE',  ( 1.000000000000000000, 0.000000000000000000, 0.000000000000000000 ) ) ;
#43310=CARTESIAN_POINT ( 'NONE',  ( -34.77165353390495284, 6.824181688848569571, 41.87898302971510844 ) ) ;
#43390=EDGE_CURVE ( 'NONE', #57160, #166090, #145569, .T. ) ;
#43410=AXIS2_PLACEMENT_3D ( 'NONE', #67943, #161955, #177147 ) ;
#43493=B_SPLINE_CURVE_WITH_KNOTS ( 'NONE', 3,
 ( #152783, #71237, #45615, #26743, #118747, #107267, #14274, #76935, #149082, #32434, #194589, #75943, #25751, #153780, #41908, #180436, #132900, #155767, #138604, #10570, #86, #185117, #168938, #56059, #61756, #123424, #169947, #109263, #60769, #139592, #92091, #62753, #46607, #117738, #1078, #30445, #91095, #103574, #165249, #137618, #122441, #108268, #31438, #154776 ),
 .UNSPECIFIED., .F., .F.,
 ( 4, 2, 2, 2, 2, 2, 2, 2, 2, 2, 2, 2, 2, 2, 2, 2, 2, 2, 2, 2, 2, 4 ),
 ( 0.01750047681075390590, 0.01897230708297386464, 0.01970822221908384228, 0.02044413735519382339, 0.02191596762741378213, 0.02338779789963374087, 0.02485962817185370308, 0.02559554330796365990, 0.02633145844407362365, 0.02706737358018358394, 0.02780328871629354423, 0.02927511898851346828, 0.03074694926073338885, 0.03221877953295330943, 0.03295469466906329054, 0.03369060980517327164, 0.03516244007739323385, 0.03663427034961320300, 0.03737018548572319798, 0.03810610062183318603, 0.03957793089405317599, 0.04104976116627316596 ),
 .UNSPECIFIED. ) ;
#43523=VERTEX_POINT ( 'NONE', #6193 ) ;
#43531=CARTESIAN_POINT ( 'NONE',  ( -36.91746825000001309, -11.99521256947794789, -11.02499999726881263 ) ) ;
#43537=CARTESIAN_POINT ( 'NONE',  ( -37.38060010999600280, -6.349431928853577212, -7.999999999999996447 ) ) ;
#43549=CARTESIAN_POINT ( 'NONE',  ( 22.81625015709509441, 31.40387420917330275, -3.824999997268813345 ) ) ;
#43557=ORIENTED_EDGE ( 'NONE', *, *, #142600, .F. ) ;
#43571=CARTESIAN_POINT ( 'NONE',  ( -31.45337032948814482, -4.959272002022346193, 100.6317495573355245 ) ) ;
#43605=CARTESIAN_POINT ( 'NONE',  ( -3.573655867282028392E-15, 2.428612866367529932E-14, 2.000000000000000000 ) ) ;
#43648=EDGE_CURVE ( 'NONE', #130010, #116580, #190230, .T. ) ;
#43721=CARTESIAN_POINT ( 'NONE',  ( 38.00000000000000711, -12.34694845685040754, -8.849999994537625980 ) ) ;
#43766=CARTESIAN_POINT ( 'NONE',  ( 31.68374724557848765, -1.945525369148856987, 102.2474955886453643 ) ) ;
#43811=CARTESIAN_POINT ( 'NONE',  ( -8.571926809382608425, 26.38167802310805854, 146.4750000027311785 ) ) ;
#43816=CARTESIAN_POINT ( 'NONE',  ( -27.73933785331498925, 9.013057229001089965, 144.7750000027311614 ) ) ;
#43889=EDGE_CURVE ( 'NONE', #9032, #58436, #93947, .T. ) ;
#43891=DIRECTION ( 'NONE',  ( -1.000000000000000000, -0.000000000000000000, -3.709348145883536076E-20 ) ) ;
#43925=CARTESIAN_POINT ( 'NONE',  ( 23.48529157249600630, -32.32473071737749137, -5.300000000000000711 ) ) ;
#43933=AXIS2_PLACEMENT_3D ( 'NONE', #72143, #165162, #74147 ) ;
#43977=CARTESIAN_POINT ( 'NONE',  ( 34.36946425582527098, 7.112708652184213776, 47.39170078794326457 ) ) ;
#44050=CARTESIAN_POINT ( 'NONE',  ( 28.82186960331498327, 2.781578969918950771E-14, 143.2500000054623683 ) ) ;
#44185=CARTESIAN_POINT ( 'NONE',  ( 37.32596994906252519, -3.631267627803086206, 40.85341334860915907 ) ) ;
#44209=ORIENTED_EDGE ( 'NONE', *, *, #36793, .T. ) ;
#44219=AXIS2_PLACEMENT_3D ( 'NONE', #103040, #27214, #56539 ) ;
#44252=CARTESIAN_POINT ( 'NONE',  ( -37.57652299961961262, -0.7251171387572962201, 39.53617709569547856 ) ) ;
#44270=ORIENTED_EDGE ( 'NONE', *, *, #81855, .F. ) ;
#44282=CARTESIAN_POINT ( 'NONE',  ( 27.73933785331498569, 2.768321779492822058E-14, 146.3750000027311842 ) ) ;
#44306=CARTESIAN_POINT ( 'NONE',  ( -35.70266437024451989, 0.2453497911276154020, 37.50000000000000711 ) ) ;
#44397=CARTESIAN_POINT ( 'NONE',  ( -22.44159573604010305, 16.30477369853692338, 141.1750000027311671 ) ) ;
#44445=EDGE_LOOP ( 'NONE', ( #108669, #151253, #116948, #54910 ) ) ;
#44483=FACE_OUTER_BOUND ( 'NONE', #166911, .T. ) ;
#44523=CARTESIAN_POINT ( 'NONE',  ( 36.91746824999999887, 11.99521256947799053, -1.524999997268813745 ) ) ;
#44524=CARTESIAN_POINT ( 'NONE',  ( -34.52594549653172606, 0.3596637467104419339, 89.49999999999899103 ) ) ;
#44530=CARTESIAN_POINT ( 'NONE',  ( 33.72265478998905053, 5.501106843017430137, 95.34580731367215378 ) ) ;
#44564=CARTESIAN_POINT ( 'NONE',  ( -31.68374724557850541, -1.945525369148830563, 102.2474955886453785 ) ) ;
#44634=FACE_OUTER_BOUND ( 'NONE', #54338, .T. ) ;
#44639=CARTESIAN_POINT ( 'NONE',  ( -32.00000000000000711, -5.510910596163089556E-15, 45.00000000000000000 ) ) ;
#44676=DIRECTION ( 'NONE',  ( 1.000000000000000000, 0.000000000000000000, 3.709348145883536076E-20 ) ) ;
#44711=CARTESIAN_POINT ( 'NONE',  ( 36.91746824999999887, 11.99521256947799053, -4.024999997268814411 ) ) ;
#44725=VERTEX_POINT ( 'NONE', #98840 ) ;
#44752=CARTESIAN_POINT ( 'NONE',  ( -27.73933785331498925, 2.428612866367529932E-14, 149.1250000027311842 ) ) ;
#44755=CARTESIAN_POINT ( 'NONE',  ( 31.71843943275782962, -0.9850135343614644379, 102.4512077271823642 ) ) ;
#44759=ADVANCED_FACE ( 'NONE', ( #190875, #83676 ), #67520, .F. ) ;
#44781=ADVANCED_FACE ( 'NONE', ( #175705 ), #112043, .F. ) ;
#44795=CARTESIAN_POINT ( 'NONE',  ( -28.82186960331499037, 2.428612866367529932E-14, 146.2500000054623683 ) ) ;
#44801=CARTESIAN_POINT ( 'NONE',  ( 8.571926809382603096, -26.38167802310801235, 147.4750000027311785 ) ) ;
#44806=CARTESIAN_POINT ( 'NONE',  ( -27.73933785331498925, 2.428612866367529932E-14, 146.8750000027311842 ) ) ;
#44815=VERTEX_POINT ( 'NONE', #161533 ) ;
#44917=CARTESIAN_POINT ( 'NONE',  ( 11.74264578624799427, 36.14014761921585972, -8.599999999999999645 ) ) ;
#44970=CARTESIAN_POINT ( 'NONE',  ( 34.59574315510280940, 4.379613810579301436, 51.09339236891210589 ) ) ;
#44984=ORIENTED_EDGE ( 'NONE', *, *, #18810, .F. ) ;
#45012=EDGE_CURVE ( 'NONE', #82818, #44725, #3852, .T. ) ;
#45039=CARTESIAN_POINT ( 'NONE',  ( 28.82186960331500813, 9.364793116373537174, 147.3500000054623627 ) ) ;
#45161=CARTESIAN_POINT ( 'NONE',  ( 29.86685920354754842, -21.69954338932559068, -1.824999997268813345 ) ) ;
#45275=CARTESIAN_POINT ( 'NONE',  ( -22.44159573604010305, 16.30477369853692338, 147.1750000027311671 ) ) ;
#45299=CARTESIAN_POINT ( 'NONE',  ( -35.63758492646881137, 1.954004632199960012, 37.74231687961064807 ) ) ;
#45321=FACE_OUTER_BOUND ( 'NONE', #92008, .T. ) ;
#45322=CARTESIAN_POINT ( 'NONE',  ( -37.99626262588766679, 2.428612866367529932E-14, -7.747842220587803475 ) ) ;
#45334=ORIENTED_EDGE ( 'NONE', *, *, #142600, .T. ) ;
#45386=CARTESIAN_POINT ( 'NONE',  ( -27.73933785331498925, 2.428612866367529932E-14, 148.8750000027311842 ) ) ;
#45400=LINE ( 'NONE', #17049, #147821 ) ;
#45439=AXIS2_PLACEMENT_3D ( 'NONE', #160773, #22263, #83912 ) ;
#45468=CARTESIAN_POINT ( 'NONE',  ( 14.18669005401828187, -34.08280046153741694, -8.000000000000001776 ) ) ;
#45490=FACE_OUTER_BOUND ( 'NONE', #86062, .T. ) ;
#45509=CARTESIAN_POINT ( 'NONE',  ( -36.91746825000001309, -11.99521256947794789, -9.024999997268812635 ) ) ;
#45510=CARTESIAN_POINT ( 'NONE',  ( -34.25194412823100976, 3.632597792548372340, 90.85486465461549699 ) ) ;
#45515=CARTESIAN_POINT ( 'NONE',  ( 33.80093248007431583, 2.440252113607736195, 99.94207534358628209 ) ) ;
#45556=CARTESIAN_POINT ( 'NONE',  ( -27.73933785331498925, -9.013057229001049109, 139.4750000027311785 ) ) ;
#45563=VERTEX_POINT ( 'NONE', #193885 ) ;
#45615=CARTESIAN_POINT ( 'NONE',  ( -31.71835025711374101, 0.9887710624358323486, 102.4506977131440237 ) ) ;
#45622=CYLINDRICAL_SURFACE ( 'NONE', #133281, 28.82186960331498682 ) ;
#45699=CARTESIAN_POINT ( 'NONE',  ( 22.81625015709510151, -31.40387420917324590, -4.424999997268812990 ) ) ;
#45790=CARTESIAN_POINT ( 'NONE',  ( 8.571926809382597767, 26.38167802310806209, 146.2750000027311899 ) ) ;
#45803=( BOUNDED_CURVE ( )  B_SPLINE_CURVE ( 2, ( #63742, #75920, #46584, #61735, #170919, #125416, #111230, #172922, #33407, #48584, #123403 ),
 .UNSPECIFIED., .F., .T. ) 
 B_SPLINE_CURVE_WITH_KNOTS ( ( 3, 2, 2, 2, 2, 3 ),
 ( 0.8000000000000007105, 0.8200000000000006173, 0.8400000000000006350, 0.8600000000000007638, 0.8800000000000007816, 0.9000000000000007994 ),
 .UNSPECIFIED. ) 
 CURVE ( )  GEOMETRIC_REPRESENTATION_ITEM ( )  RATIONAL_B_SPLINE_CURVE ( ( 0.9999999999999983347, 0.9510565162951551965, 1.000000000000000000, 0.9510565162951535312, 1.000000000000000000, 0.9510565162951535312, 1.000000000000000000, 0.9510565162951535312, 1.000000000000000000, 0.9510565162951516438, 1.000000000000001998 ) ) 
 REPRESENTATION_ITEM ( '' )  );
#45864=CARTESIAN_POINT ( 'NONE',  ( 17.14385361876520264, 23.59649016807275856, 148.6750000027311387 ) ) ;
#45867=CARTESIAN_POINT ( 'NONE',  ( -30.00000000000000000, -1.163414459189985801E-14, 95.00000000000000000 ) ) ;
#45902=CARTESIAN_POINT ( 'NONE',  ( -11.74264578624799782, -36.14014761921581709, -9.600000000000001421 ) ) ;
#45952=DIRECTION ( 'NONE',  ( 0.000000000000000000, 0.000000000000000000, -1.000000000000000000 ) ) ;
#46215=CARTESIAN_POINT ( 'NONE',  ( 37.58407650405589351, 2.428612866815129610E-14, 39.49999999999996447 ) ) ;
#46230=CARTESIAN_POINT ( 'NONE',  ( -36.87149605698876087, -2.274342727564272693, 50.01098105774816105 ) ) ;
#46250=AXIS2_PLACEMENT_3D ( 'NONE', #173436, #53053, #96561 ) ;
#46261=CARTESIAN_POINT ( 'NONE',  ( -8.571926809382608425, 26.38167802310805854, 146.9750000027311785 ) ) ;
#46284=CARTESIAN_POINT ( 'NONE',  ( -35.41256452865198412, 3.967314244253445032, 38.63057146076392456 ) ) ;
#46305=DIRECTION ( 'NONE',  ( 1.000000000000000000, 0.000000000000000000, 0.000000000000000000 ) ) ;
#46372=CARTESIAN_POINT ( 'NONE',  ( -17.14385361876520975, 23.59649016807275856, 146.5750000027311728 ) ) ;
#46374=VERTEX_POINT ( 'NONE', #155078 ) ;
#46392=DIRECTION ( 'NONE',  ( 0.06104853953485701173, 0.000000000000000000, -0.9981347984218670311 ) ) ;
#46421=ORIENTED_EDGE ( 'NONE', *, *, #43648, .F. ) ;
#46471=DIRECTION ( 'NONE',  ( 1.000000000000000000, 0.000000000000000000, 0.000000000000000000 ) ) ;
#46500=CARTESIAN_POINT ( 'NONE',  ( -22.81625015709509441, -31.40387420917324590, -10.82499999726881157 ) ) ;
#46520=CARTESIAN_POINT ( 'NONE',  ( -22.81625015709509441, -31.40387420917324590, -6.824999997268814234 ) ) ;
#46528=EDGE_LOOP ( 'NONE', ( #19196, #118842, #67309, #158152 ) ) ;
#46549=CARTESIAN_POINT ( 'NONE',  ( 22.44159573604009594, -16.30477369853687364, 140.1750000027311955 ) ) ;
#46584=CARTESIAN_POINT ( 'NONE',  ( -23.31738231874055600, 16.94106989632528837, 141.7999999999999829 ) ) ;
#46607=CARTESIAN_POINT ( 'NONE',  ( -31.99745974829804140, 5.643669518723349654, 90.03617080843918075 ) ) ;
#46694=CARTESIAN_POINT ( 'NONE',  ( -22.81625015709510507, 31.40387420917330275, -9.424999997268812990 ) ) ;
#46781=DIRECTION ( 'NONE',  ( 0.000000000000000000, 0.000000000000000000, -1.000000000000000000 ) ) ;
#46786=CARTESIAN_POINT ( 'NONE',  ( -5.359611314223446995E-15, 29.16686587814335496, 148.3750000027311842 ) ) ;
#46820=CIRCLE ( 'NONE', #37139, 2.649999999999999467 ) ;
#46870=TOROIDAL_SURFACE ( 'NONE', #156560, 2.700000000000000622, 0.2000000000000000111 ) ;
#46951=CARTESIAN_POINT ( 'NONE',  ( 35.69940131823276630, 0.4911691522782191677, 37.51200899188186355 ) ) ;
#47144=CARTESIAN_POINT ( 'NONE',  ( 29.86685920354754487, 21.69954338932564752, -3.424999997268813434 ) ) ;
#47195=CIRCLE ( 'NONE', #98831, 2.649999999999999467 ) ;
#47233=DIRECTION ( 'NONE',  ( -0.8660254037844410391, -0.000000000000000000, -0.4999999999999958367 ) ) ;
#47243=CARTESIAN_POINT ( 'NONE',  ( -3.573655867282028392E-15, 2.428612866367529932E-14, 139.9999999999999716 ) ) ;
#47265=CARTESIAN_POINT ( 'NONE',  ( 27.73933785331498569, 2.768321779492822058E-14, 142.3750000027311842 ) ) ;
#47289=CARTESIAN_POINT ( 'NONE',  ( 8.906447517083057264, -27.41122689804191026, 140.5999999999999943 ) ) ;
#47290=CARTESIAN_POINT ( 'NONE',  ( 8.906447517083050158, 27.41122689804195645, 143.6500000054623740 ) ) ;
#47351=ADVANCED_FACE ( 'NONE', ( #57994 ), #15089, .F. ) ;
#47381=CARTESIAN_POINT ( 'NONE',  ( 27.73933785331498925, -9.013057229001034898, 141.7750000027311899 ) ) ;
#47391=VECTOR ( 'NONE', #132819, 1000.000000000000114 ) ;
#47400=CARTESIAN_POINT ( 'NONE',  ( 30.73962218707677607, 22.33364281372847060, -6.802157773949823572 ) ) ;
#47486=AXIS2_PLACEMENT_3D ( 'NONE', #174394, #96527, #64227 ) ;
#47494=EDGE_LOOP ( 'NONE', ( #149638, #5003, #60952, #27895 ) ) ;
#47506=CARTESIAN_POINT ( 'NONE',  ( 29.86685920354754487, 21.69954338932564752, -7.924999997268814766 ) ) ;
#47511=CARTESIAN_POINT ( 'NONE',  ( 34.46456012332993879, 1.775814316247266156, 89.78225565739066383 ) ) ;
#47698=CARTESIAN_POINT ( 'NONE',  ( -5.950531402560715689E-15, 38.81732327939063509, -7.624999997268814056 ) ) ;
#47760=CARTESIAN_POINT ( 'NONE',  ( -11.74149087413294623, -36.13659316521243881, -7.602157773949822506 ) ) ;
#47780=CARTESIAN_POINT ( 'NONE',  ( 32.00000000000000000, -5.510910596163089556E-15, 45.00000000000000000 ) ) ;
#47786=CARTESIAN_POINT ( 'NONE',  ( 22.44159573604009239, 16.30477369853692693, 142.0750000027311728 ) ) ;
#47794=EDGE_CURVE ( 'NONE', #170159, #53763, #151749, .T. ) ;
#47880=CARTESIAN_POINT ( 'NONE',  ( 1.993301997531345686E-15, -30.30510711980685556, 144.7500000054623399 ) ) ;
#47899=DIRECTION ( 'NONE',  ( -1.000000000000000000, 0.000000000000000000, 0.000000000000000000 ) ) ;
#48134=VERTEX_POINT ( 'NONE', #141537 ) ;
#48139=CARTESIAN_POINT ( 'NONE',  ( -11.40812507854755609, 35.11059874428196537, -5.024999997268813523 ) ) ;
#48212=FACE_OUTER_BOUND ( 'NONE', #773, .T. ) ;
#48261=CARTESIAN_POINT ( 'NONE',  ( 8.906447517083057264, -27.41122689804191026, 148.5999999999999943 ) ) ;
#48285=CARTESIAN_POINT ( 'NONE',  ( 28.82186960331498327, 9.364793116373570925, 143.3500000054623342 ) ) ;
#48306=CIRCLE ( 'NONE', #193659, 0.1999999999999987899 ) ;
#48377=CARTESIAN_POINT ( 'NONE',  ( 8.571926809382603096, -26.38167802310801235, 143.4750000027312069 ) ) ;
#48393=CARTESIAN_POINT ( 'NONE',  ( -23.31738231874055600, 16.94106989632528837, 142.0500000054623513 ) ) ;
#48503=CARTESIAN_POINT ( 'NONE',  ( -11.40812507854754720, -35.11059874428192273, -6.224999997268812812 ) ) ;
#48520=CARTESIAN_POINT ( 'NONE',  ( -11.40812507854754720, -35.11059874428192273, -4.724999997268812812 ) ) ;
#48528=ORIENTED_EDGE ( 'NONE', *, *, #30819, .T. ) ;
#48554=CARTESIAN_POINT ( 'NONE',  ( 35.24470855014509141, -4.955302550156627461, 39.34877664276073261 ) ) ;
#48559=CYLINDRICAL_SURFACE ( 'NONE', #198726, 28.82186960331498682 ) ;
#48582=CARTESIAN_POINT ( 'NONE',  ( 32.00000000000000000, -5.510910596163089556E-15, 45.00000000000000000 ) ) ;
#48584=CARTESIAN_POINT ( 'NONE',  ( 28.82186960331521419, 9.364793116373263615, 141.0999999999999943 ) ) ;
#48616=CIRCLE ( 'NONE', #77615, 2.649999999999999467 ) ;
#48689=CARTESIAN_POINT ( 'NONE',  ( 22.81625015709509441, 31.40387420917330275, -7.824999997268813345 ) ) ;
#48747=DIRECTION ( 'NONE',  ( -1.000000000000000000, 0.000000000000000000, 0.000000000000000000 ) ) ;
#48771=DIRECTION ( 'NONE',  ( 0.06104853953485701173, 0.000000000000000000, -0.9981347984218670311 ) ) ;
#48776=CARTESIAN_POINT ( 'NONE',  ( 27.73933785331498214, 9.013057229001095294, 139.9750000027311501 ) ) ;
#48782=CARTESIAN_POINT ( 'NONE',  ( 17.14385361876520264, -23.59649016807271238, 139.5750000027311444 ) ) ;
#48846=CARTESIAN_POINT ( 'NONE',  ( -28.82186960331508985, -9.364793116373393289, 146.0999999999999659 ) ) ;
#48848=CARTESIAN_POINT ( 'NONE',  ( 8.571926809382603096, -26.38167802310801235, 145.9750000027311785 ) ) ;
#49010=CARTESIAN_POINT ( 'NONE',  ( 29.86685920354754487, 21.69954338932564752, -1.424999997268813212 ) ) ;
#49094=DIRECTION ( 'NONE',  ( 0.000000000000000000, 0.000000000000000000, 1.000000000000000000 ) ) ;
#49097=CARTESIAN_POINT ( 'NONE',  ( 34.29482437030766562, -3.353353130260861459, 90.62592007927790405 ) ) ;
#49126=ORIENTED_EDGE ( 'NONE', *, *, #121041, .F. ) ;
#49131=CARTESIAN_POINT ( 'NONE',  ( 29.86685920354754842, -21.69954338932559068, -3.824999997268813345 ) ) ;
#49203=CYLINDRICAL_SURFACE ( 'NONE', #198404, 2.649999999999999467 ) ;
#49219=CARTESIAN_POINT ( 'NONE',  ( -30.73962218707678318, 22.33364281372846705, -5.947842220587803652 ) ) ;
#49248=CARTESIAN_POINT ( 'NONE',  ( 22.44159573604009594, -16.30477369853687364, 140.1750000027311955 ) ) ;
#49271=CARTESIAN_POINT ( 'NONE',  ( -5.359611314223446995E-15, 29.16686587814335496, 148.3750000027311842 ) ) ;
#49302=EDGE_CURVE ( 'NONE', #77271, #97477, #27310, .T. ) ;
#49359=CARTESIAN_POINT ( 'NONE',  ( 17.14385361876520264, -23.59649016807270883, 141.5750000027311728 ) ) ;
#49369=ADVANCED_FACE ( 'NONE', ( #22178 ), #163701, .F. ) ;
#49370=EDGE_CURVE ( 'NONE', #50285, #14250, #21176, .T. ) ;
#49377=CARTESIAN_POINT ( 'NONE',  ( 8.906447517083050158, 27.41122689804195645, 141.6500000054623740 ) ) ;
#49451=ORIENTED_EDGE ( 'NONE', *, *, #171492, .T. ) ;
#49483=CARTESIAN_POINT ( 'NONE',  ( 22.81625015709510151, -31.40387420917324590, -5.924999997268812990 ) ) ;
#49484=CARTESIAN_POINT ( 'NONE',  ( -33.85315667487628133, 0.3602237081833374321, 100.5000000000010516 ) ) ;
#49508=ORIENTED_EDGE ( 'NONE', *, *, #14461, .T. ) ;
#49542=CARTESIAN_POINT ( 'NONE',  ( -3.573655867282028392E-15, 2.428612866367529932E-14, 2.000000000000000000 ) ) ;
#49671=DIRECTION ( 'NONE',  ( -1.000000000000000000, 0.000000000000000000, 0.000000000000000000 ) ) ;
#49674=CARTESIAN_POINT ( 'NONE',  ( 22.81625015709510151, -31.40387420917324590, -10.42499999726881477 ) ) ;
#49688=VERTEX_POINT ( 'NONE', #13982 ) ;
#49762=( GEOMETRIC_REPRESENTATION_CONTEXT ( 3 ) GLOBAL_UNCERTAINTY_ASSIGNED_CONTEXT ( ( #146977 ) ) GLOBAL_UNIT_ASSIGNED_CONTEXT ( ( #89080, #10261, #149764 ) ) REPRESENTATION_CONTEXT ( 'NONE', 'WORKASPACE' ) );
#49764=CARTESIAN_POINT ( 'NONE',  ( 27.73933785331498925, -9.013057229001033122, 141.7750000027311899 ) ) ;
#49765=ADVANCED_FACE ( 'NONE', ( #11017 ), #49933, .T. ) ;
#49837=CARTESIAN_POINT ( 'NONE',  ( 1.784210473542230573E-15, -29.16686587814331588, 147.8750000027311273 ) ) ;
#49933=TOROIDAL_SURFACE ( 'NONE', #72475, 2.700000000000000622, 0.2000000000000000111 ) ;
#50000=CARTESIAN_POINT ( 'NONE',  ( 22.81625015709510151, -31.40387420917324590, -3.924999997268812102 ) ) ;
#50081=CARTESIAN_POINT ( 'NONE',  ( -40.00200000000003087, -5.510910596163089556E-15, 45.00000000000000000 ) ) ;
#50120=ORIENTED_EDGE ( 'NONE', *, *, #168447, .T. ) ;
#50125=CARTESIAN_POINT ( 'NONE',  ( -11.40812507854754720, -35.11059874428192273, -10.22499999726881548 ) ) ;
#50203=DIRECTION ( 'NONE',  ( 0.000000000000000000, 0.000000000000000000, -1.000000000000000000 ) ) ;
#50220=CARTESIAN_POINT ( 'NONE',  ( -6.019987952026119621E-15, 39.95163481335720235, -6.247842220587802586 ) ) ;
#50221=CARTESIAN_POINT ( 'NONE',  ( 32.50820986112747590, -2.649538386493603515, 87.97934651352352375 ) ) ;
#50250=CARTESIAN_POINT ( 'NONE',  ( 28.82186960331498327, 2.781578969918950771E-14, 147.0000000000000000 ) ) ;
#50271=CARTESIAN_POINT ( 'NONE',  ( 23.31738231874054890, -16.94106989632523508, 140.7999999999999829 ) ) ;
#50272=CARTESIAN_POINT ( 'NONE',  ( 8.906447517083057264, -27.41122689804191026, 142.8500000054623911 ) ) ;
#50285=VERTEX_POINT ( 'NONE', #55270 ) ;
#50293=CARTESIAN_POINT ( 'NONE',  ( -28.82186960331518932, -9.364793116373263615, 142.0999999999999943 ) ) ;
#50364=CARTESIAN_POINT ( 'NONE',  ( -22.44159573604010305, 16.30477369853692338, 146.6750000027311671 ) ) ;
#50381=CARTESIAN_POINT ( 'NONE',  ( 8.906447517083057264, -27.41122689804191026, 148.5999999999999943 ) ) ;
#50385=CARTESIAN_POINT ( 'NONE',  ( 36.80065496640121836, -5.465942522010069027, 45.70922642070194541 ) ) ;
#50421=CARTESIAN_POINT ( 'NONE',  ( 28.82186960331498327, 2.781578969918950771E-14, 149.0000000000000000 ) ) ;
#50464=CARTESIAN_POINT ( 'NONE',  ( -3.573655867282028392E-15, 2.428612866367529932E-14, 2.000000000000000000 ) ) ;
#50484=CARTESIAN_POINT ( 'NONE',  ( -29.86685920354755552, 21.69954338932564397, -4.824999997268814234 ) ) ;
#50509=EDGE_CURVE ( 'NONE', #187938, #60305, #139087, .T. ) ;
#50539=CARTESIAN_POINT ( 'NONE',  ( 34.54531151325587501, -4.968019249220454903, 50.63996542006481860 ) ) ;
#50691=ORIENTED_EDGE ( 'NONE', *, *, #33197, .F. ) ;
#50727=CARTESIAN_POINT ( 'NONE',  ( -33.70211957050084095, -4.378872343537607570, 98.34732289368837144 ) ) ;
#50728=CARTESIAN_POINT ( 'NONE',  ( 1.601920565550454256, -37.08308084913829816, -8.000000000000000000 ) ) ;
#50764=CARTESIAN_POINT ( 'NONE',  ( -27.73933785331498925, 9.013057229001089965, 149.2750000027311330 ) ) ;
#50771=DIRECTION ( 'NONE',  ( 1.000000000000000000, -0.000000000000000000, -0.000000000000000000 ) ) ;
#50775=VERTEX_POINT ( 'NONE', #29667 ) ;
#50799=ORIENTED_EDGE ( 'NONE', *, *, #121415, .T. ) ;
#50834=CARTESIAN_POINT ( 'NONE',  ( 27.73933785331498925, -9.013057229001034898, 142.2750000027311899 ) ) ;
#50910=CARTESIAN_POINT ( 'NONE',  ( 38.00000000000000000, 12.34694845685046616, -4.649999994537627579 ) ) ;
#50991=CARTESIAN_POINT ( 'NONE',  ( 36.91746824999999177, 2.880721459617395097E-14, -3.624999997268813168 ) ) ;
#51058=DIRECTION ( 'NONE',  ( 1.000000000000000000, 0.000000000000000000, 0.000000000000000000 ) ) ;
#51111=CARTESIAN_POINT ( 'NONE',  ( 36.91746824999999887, 11.99521256947799053, -7.524999997268814411 ) ) ;
#51201=CARTESIAN_POINT ( 'NONE',  ( 31.43434485161623826, -5.140865793513109239, 100.4663950908259125 ) ) ;
#51231=CARTESIAN_POINT ( 'NONE',  ( -8.906447517083060816, 27.41122689804195645, 147.5999999999999943 ) ) ;
#51253=CARTESIAN_POINT ( 'NONE',  ( 23.31738231874054534, 16.94106989632529192, 141.4500000054623854 ) ) ;
#51286=EDGE_CURVE ( 'NONE', #31542, #44815, #142561, .T. ) ;
#51317=CARTESIAN_POINT ( 'NONE',  ( 30.73962218707677252, 22.33364281372847060, -2.547842220587803297 ) ) ;
#51359=LINE ( 'NONE', #174712, #180173 ) ;
#51365=CARTESIAN_POINT ( 'NONE',  ( 36.86261346499075131, -5.499032313789902204, 44.62661474502113634 ) ) ;
#51421=CARTESIAN_POINT ( 'NONE',  ( -27.73933785331498925, 2.428612866367529932E-14, 139.1250000027311842 ) ) ;
#51465=CARTESIAN_POINT ( 'NONE',  ( 36.91746824999999887, 11.99521256947799053, -5.524999997268812635 ) ) ;
#51466=CARTESIAN_POINT ( 'NONE',  ( -33.79632059884287543, 5.461862605997785280, 94.26112944759005075 ) ) ;
#51521=CARTESIAN_POINT ( 'NONE',  ( 34.91229673954796908, -6.363315211036958630, 41.02293916657587403 ) ) ;
#51746=CARTESIAN_POINT ( 'NONE',  ( -8.571926809382601320, -26.38167802310801591, 147.7750000027311899 ) ) ;
#51790=EDGE_CURVE ( 'NONE', #171099, #33122, #59600, .T. ) ;
#51817=CARTESIAN_POINT ( 'NONE',  ( 27.73933785331498925, -9.013057229001034898, 146.2750000027311899 ) ) ;
#51870=ADVANCED_FACE ( 'NONE', ( #112228, #173918 ), #110234, .F. ) ;
#51896=CARTESIAN_POINT ( 'NONE',  ( -11.74264578624800670, 36.14014761921585972, -4.149999994537627579 ) ) ;
#51934=EDGE_LOOP ( 'NONE', ( #94812, #15197 ) ) ;
#51946=CARTESIAN_POINT ( 'NONE',  ( 29.86685920354754842, -21.69954338932559068, -6.324999997268814234 ) ) ;
#51979=CARTESIAN_POINT ( 'NONE',  ( 36.91746824999999177, 11.99521256947799230, -3.524999997268813079 ) ) ;
#52062=FACE_BOUND ( 'NONE', #14682, .T. ) ;
#52075=DIRECTION ( 'NONE',  ( 1.000000000000000000, -0.000000000000000000, -0.000000000000000000 ) ) ;
#52100=CARTESIAN_POINT ( 'NONE',  ( -22.81625015709509441, -31.40387420917324590, -10.32499999726881157 ) ) ;
#52189=CARTESIAN_POINT ( 'NONE',  ( 31.54463713289763049, -7.108708273820915302, 92.55936662351712130 ) ) ;
#52219=CARTESIAN_POINT ( 'NONE',  ( 8.571926809382603096, -26.38167802310801235, 139.9750000027311785 ) ) ;
#52241=CARTESIAN_POINT ( 'NONE',  ( -28.82186960331499037, 2.428612866367529932E-14, 142.2500000054623683 ) ) ;
#52285=( BOUNDED_CURVE ( )  B_SPLINE_CURVE ( 2, ( #171081, #32572, #18408, #107404, #122582, #93228, #92235, #15415, #140732, #110394, #139726 ),
 .UNSPECIFIED., .F., .F. ) 
 B_SPLINE_CURVE_WITH_KNOTS ( ( 3, 2, 2, 2, 2, 3 ),
 ( 0.2000000000000001776, 0.2200000000000001954, 0.2400000000000002132, 0.2600000000000002309, 0.2800000000000003042, 0.3000000000000002665 ),
 .UNSPECIFIED. ) 
 CURVE ( )  GEOMETRIC_REPRESENTATION_ITEM ( )  RATIONAL_B_SPLINE_CURVE ( ( 0.9999999999999995559, 0.9510565162951539753, 1.000000000000000000, 0.9510565162951535312, 1.000000000000000000, 0.9510565162951535312, 1.000000000000000000, 0.9510565162951535312, 1.000000000000000000, 0.9510565162951528650, 1.000000000000000666 ) ) 
 REPRESENTATION_ITEM ( '' )  );
#52331=ORIENTED_EDGE ( 'NONE', *, *, #54728, .T. ) ;
#52334=CARTESIAN_POINT ( 'NONE',  ( 27.73933785331498569, 9.013057229001093518, 139.9750000027311785 ) ) ;
#52351=CARTESIAN_POINT ( 'NONE',  ( -32.00000000000000000, -5.510910596163089556E-15, 45.00000000000000000 ) ) ;
#52353=CARTESIAN_POINT ( 'NONE',  ( 36.81794758165437997, -5.500929263287720694, 45.34431116311555598 ) ) ;
#52455=CARTESIAN_POINT ( 'NONE',  ( -36.91746825000000598, 2.428612866367529932E-14, -8.624999997268814056 ) ) ;
#52509=CARTESIAN_POINT ( 'NONE',  ( 35.52771690032645324, -3.099362195827463751, 38.16599597228978524 ) ) ;
#52550=PLANE ( 'NONE',  #150037 ) ;
#52612=FACE_OUTER_BOUND ( 'NONE', #128988, .T. ) ;
#52654=CARTESIAN_POINT ( 'NONE',  ( 11.40812507854754365, 35.11059874428196537, -9.724999997268813701 ) ) ;
#52667=EDGE_LOOP ( 'NONE', ( #52772, #81834 ) ) ;
#52706=CARTESIAN_POINT ( 'NONE',  ( -3.573655867282028392E-15, 2.428612866367529932E-14, 139.9999999999999716 ) ) ;
#52723=AXIS2_PLACEMENT_3D ( 'NONE', #77432, #1579, #93588 ) ;
#52737=CARTESIAN_POINT ( 'NONE',  ( -27.73933785331498925, 2.428612866367529932E-14, 145.3750000027311842 ) ) ;
#52741=CARTESIAN_POINT ( 'NONE',  ( -23.48298174826589602, -32.32155151706771790, -5.447842220587802764 ) ) ;
#52772=ORIENTED_EDGE ( 'NONE', *, *, #166279, .T. ) ;
#52806=ORIENTED_EDGE ( 'NONE', *, *, #139182, .F. ) ;
#52809=CARTESIAN_POINT ( 'NONE',  ( -22.44159573604010305, 16.30477369853692338, 143.1750000027311671 ) ) ;
#52885=CARTESIAN_POINT ( 'NONE',  ( 3.766062262543149401E-15, -39.95556452105413570, -7.249999994537627224 ) ) ;
#52935=CARTESIAN_POINT ( 'NONE',  ( -36.91746825000000598, 2.428612866367529932E-14, -3.124999997268813168 ) ) ;
#52937=CARTESIAN_POINT ( 'NONE',  ( -35.59965464630457888, -2.422542088861810772, 37.88523239209964544 ) ) ;
#52966=CARTESIAN_POINT ( 'NONE',  ( 11.40812507854754365, 35.11059874428196537, -1.224999997268813479 ) ) ;
#53035=EDGE_CURVE ( 'NONE', #115964, #89861, #197071, .T. ) ;
#53053=DIRECTION ( 'NONE',  ( 0.000000000000000000, 0.000000000000000000, 1.000000000000000000 ) ) ;
#53065=AXIS2_PLACEMENT_3D ( 'NONE', #63255, #14781, #49094 ) ;
#53091=CARTESIAN_POINT ( 'NONE',  ( 29.86685920354754487, 21.69954338932564752, -5.424999997268813878 ) ) ;
#53154=EDGE_LOOP ( 'NONE', ( #186535, #91073, #10251, #113865, #177040, #156490, #48528, #174458, #39121, #20418, #9675, #28252, #88230, #166700 ) ) ;
#53183=VECTOR ( 'NONE', #151367, 1000.000000000000000 ) ;
#53214=CARTESIAN_POINT ( 'NONE',  ( 28.82186960331498327, 2.781578969918950771E-14, 143.0000000000000000 ) ) ;
#53239=CARTESIAN_POINT ( 'NONE',  ( -8.906447517083053711, -27.41122689804191026, 138.6500000054623740 ) ) ;
#53281=ORIENTED_EDGE ( 'NONE', *, *, #187248, .T. ) ;
#53306=AXIS2_PLACEMENT_3D ( 'NONE', #50081, #33914, #65234 ) ;
#53351=CARTESIAN_POINT ( 'NONE',  ( 36.90807327575559071, -0.7244114042849700841, 50.46397389534120492 ) ) ;
#53428=LINE ( 'NONE', #174791, #60500 ) ;
#53439=EDGE_CURVE ( 'NONE', #49688, #193619, #159741, .T. ) ;
#53448=DIRECTION ( 'NONE',  ( 1.000000000000000000, 0.000000000000000000, 0.000000000000000000 ) ) ;
#53506=CARTESIAN_POINT ( 'NONE',  ( 30.00000000000000000, -5.510910596163089556E-15, 45.00000000000000000 ) ) ;
#53535=CARTESIAN_POINT ( 'NONE',  ( -37.99626262588769521, 12.34573411038911317, -4.102157773949822506 ) ) ;
#53656=CARTESIAN_POINT ( 'NONE',  ( -30.73962218707678318, -22.33364281372842441, -5.802157773949822683 ) ) ;
#53663=CARTESIAN_POINT ( 'NONE',  ( 36.67794138864803699, -4.841227315053108882, -7.999999999999994671 ) ) ;
#53712=CARTESIAN_POINT ( 'NONE',  ( -33.70754165857147200, -5.457863348371953194, 95.70317755519533875 ) ) ;
#53713=CARTESIAN_POINT ( 'NONE',  ( 6.906787368987876263, -36.38763403141891217, -7.999999999999998224 ) ) ;
#53723=CIRCLE ( 'NONE', #140742, 29.43349580481983807 ) ;
#53748=CARTESIAN_POINT ( 'NONE',  ( -31.31738933903720223, -7.498949511226637554, 94.72411213025000620 ) ) ;
#53752=CARTESIAN_POINT ( 'NONE',  ( -27.73933785331498925, -9.013057229001049109, 141.4750000027311785 ) ) ;
#53756=CARTESIAN_POINT ( 'NONE',  ( 30.73962218707677607, -22.33364281372841376, -4.947842220587803652 ) ) ;
#53763=VERTEX_POINT ( 'NONE', #34793 ) ;
#53782=CARTESIAN_POINT ( 'NONE',  ( 31.79999999999968807, 4.791014396527177230E-13, 45.00000000000022027 ) ) ;
#53826=CARTESIAN_POINT ( 'NONE',  ( 22.44159573604009594, -16.30477369853687364, 140.1750000027311955 ) ) ;
#53903=CARTESIAN_POINT ( 'NONE',  ( 37.99999999999999289, 2.893978650043524126E-14, -6.749999994537627224 ) ) ;
#53938=CARTESIAN_POINT ( 'NONE',  ( 31.30058771566192988, 6.382914491190405215, 98.94581565101640308 ) ) ;
#54053=( BOUNDED_CURVE ( )  B_SPLINE_CURVE ( 2, ( #159700, #82853, #50271, #32115, #47289, #127080, #126105, #92770, #188788, #199975, #110928 ),
 .UNSPECIFIED., .F., .F. ) 
 B_SPLINE_CURVE_WITH_KNOTS ( ( 3, 2, 2, 2, 2, 3 ),
 ( 0.9000000000000007994, 0.9200000000000007061, 0.9400000000000003908, 0.9600000000000002975, 0.9800000000000002043, 1.000000000000000000 ),
 .UNSPECIFIED. ) 
 CURVE ( )  GEOMETRIC_REPRESENTATION_ITEM ( )  RATIONAL_B_SPLINE_CURVE ( ( 0.9999999999999981126, 0.9510565162951554186, 1.000000000000000000, 0.9510565162951535312, 1.000000000000000000, 0.9510565162951535312, 1.000000000000000000, 0.9510565162951535312, 1.000000000000000000, 0.9510565162951535312, 1.000000000000000000 ) ) 
 REPRESENTATION_ITEM ( '' )  );
#54106=CARTESIAN_POINT ( 'NONE',  ( 29.86685920354754842, -21.69954338932559068, -5.824999997268813345 ) ) ;
#54169=VERTEX_POINT ( 'NONE', #4431 ) ;
#54227=CARTESIAN_POINT ( 'NONE',  ( -28.82186960331499037, 2.428612866367529932E-14, 148.2500000054623683 ) ) ;
#54281=DIRECTION ( 'NONE',  ( 0.000000000000000000, 0.000000000000000000, -1.000000000000000000 ) ) ;
#54338=EDGE_LOOP ( 'NONE', ( #96944, #190020, #13120, #178328 ) ) ;
#54358=CARTESIAN_POINT ( 'NONE',  ( 36.91128768240055535, -0.3593773198236868138, 50.50000000000002842 ) ) ;
#54415=CARTESIAN_POINT ( 'NONE',  ( -5.429308488886486681E-15, 30.30510711980690175, 145.4999999999999716 ) ) ;
#54417=( BOUNDED_CURVE ( )  B_SPLINE_CURVE ( 2, ( #151597, #178956, #148608, #40426, #10100, #179966, #199083, #11100, #58580, #27271, #120246 ),
 .UNSPECIFIED., .F., .T. ) 
 B_SPLINE_CURVE_WITH_KNOTS ( ( 3, 2, 2, 2, 2, 3 ),
 ( 0.7000000000000001776, 0.7200000000000001954, 0.7400000000000001021, 0.7600000000000001199, 0.7800000000000000266, 0.8000000000000000444 ),
 .UNSPECIFIED. ) 
 CURVE ( )  GEOMETRIC_REPRESENTATION_ITEM ( )  RATIONAL_B_SPLINE_CURVE ( ( 0.9999999999999994449, 0.9510565162951540863, 1.000000000000000000, 0.9510565162951535312, 1.000000000000000000, 0.9510565162951535312, 1.000000000000000000, 0.9510565162951535312, 1.000000000000000000, 0.9510565162951535312, 1.000000000000000000 ) ) 
 REPRESENTATION_ITEM ( '' )  );
#54432=CARTESIAN_POINT ( 'NONE',  ( -26.63278688795740834, 27.10001173645601114, -8.000000000000000000 ) ) ;
#54448=ORIENTED_EDGE ( 'NONE', *, *, #16286, .F. ) ;
#54451=DIRECTION ( 'NONE',  ( -1.000000000000000000, 0.000000000000000000, 0.000000000000000000 ) ) ;
#54461=CARTESIAN_POINT ( 'NONE',  ( -8.571926809382601320, -26.38167802310801591, 147.7750000027311899 ) ) ;
#54483=CARTESIAN_POINT ( 'NONE',  ( -34.46971384048858766, 7.497988128173094680, 44.47943501004273514 ) ) ;
#54625=ADVANCED_FACE ( 'NONE', ( #98432 ), #160128, .F. ) ;
#54707=CARTESIAN_POINT ( 'NONE',  ( -19.63849963310777369, -31.90967075912679718, -8.000000000000000000 ) ) ;
#54728=EDGE_CURVE ( 'NONE', #50285, #44725, #32747, .T. ) ;
#54741=CARTESIAN_POINT ( 'NONE',  ( -32.15403441185031141, -4.954129643790889048, 89.34785441345069046 ) ) ;
#54745=CARTESIAN_POINT ( 'NONE',  ( -17.14385361876520264, -23.59649016807271593, 145.6750000027311671 ) ) ;
#54751=CARTESIAN_POINT ( 'NONE',  ( 23.48298174826590667, -32.32155151706770368, -5.047842220587804185 ) ) ;
#54770=EDGE_CURVE ( 'NONE', #177652, #26356, #175937, .T. ) ;
#54864=LINE ( 'NONE', #117536, #8657 ) ;
#54897=CARTESIAN_POINT ( 'NONE',  ( -11.74264578624800670, 36.14014761921585972, -10.14999999453762669 ) ) ;
#54910=ORIENTED_EDGE ( 'NONE', *, *, #73347, .T. ) ;
#54935=CARTESIAN_POINT ( 'NONE',  ( 31.71835025711371259, 0.9887710624358057032, 102.4506977131440522 ) ) ;
#54948=CARTESIAN_POINT ( 'NONE',  ( 37.11214605083871021, 4.768680519348648339, 42.23634591622184331 ) ) ;
#54981=CARTESIAN_POINT ( 'NONE',  ( -37.32565804592077541, 3.633088190964871345, 40.85532123380856007 ) ) ;
#55000=VERTEX_POINT ( 'NONE', #146962 ) ;
#55097=ORIENTED_EDGE ( 'NONE', *, *, #149178, .F. ) ;
#55102=CARTESIAN_POINT ( 'NONE',  ( 37.99999999999999289, 2.893978650043524126E-14, -7.000000000000000000 ) ) ;
#55147=ORIENTED_EDGE ( 'NONE', *, *, #92301, .T. ) ;
#55221=CARTESIAN_POINT ( 'NONE',  ( -28.82186960331499392, -9.364793116373526516, 140.0999999999999943 ) ) ;
#55270=CARTESIAN_POINT ( 'NONE',  ( -35.70266437024450568, -5.510913496957479854E-15, 37.50000000000000000 ) ) ;
#55352=CARTESIAN_POINT ( 'NONE',  ( 37.48574882824303245, -2.272739345372913000, 39.98829423970371977 ) ) ;
#55409=CARTESIAN_POINT ( 'NONE',  ( -28.82186960331499037, 2.428612866367529932E-14, 146.0000000000000000 ) ) ;
#55424=CARTESIAN_POINT ( 'NONE',  ( 33.56183721214949145, 15.50984559938615526, -7.999999999999996447 ) ) ;
#55427=CARTESIAN_POINT ( 'NONE',  ( 8.906447517083057264, -27.41122689804191026, 140.8500000054623911 ) ) ;
#55455=CARTESIAN_POINT ( 'NONE',  ( 36.91746824999999887, 11.99521256947799053, -9.524999997268812635 ) ) ;
#55479=CARTESIAN_POINT ( 'NONE',  ( -35.13534055906293929, 5.469967203781493481, 39.86293573631996168 ) ) ;
#55497=ORIENTED_EDGE ( 'NONE', *, *, #123690, .T. ) ;
#55511=DIRECTION ( 'NONE',  ( 0.000000000000000000, 0.000000000000000000, -1.000000000000000000 ) ) ;
#55516=DIRECTION ( 'NONE',  ( 1.000000000000000000, 0.000000000000000000, 3.709348145883536076E-20 ) ) ;
#55558=DIRECTION ( 'NONE',  ( 0.000000000000000000, 0.000000000000000000, -1.000000000000000000 ) ) ;
#55709=CARTESIAN_POINT ( 'NONE',  ( -37.96308138437226631, -1.796937805546485301, -7.999999999999996447 ) ) ;
#55721=CARTESIAN_POINT ( 'NONE',  ( 36.91746824999999177, 2.880721459617395097E-14, -2.124999997268813168 ) ) ;
#55742=CARTESIAN_POINT ( 'NONE',  ( -31.23717829866982854, -7.254840157072011131, 96.91794063280337923 ) ) ;
#55746=CARTESIAN_POINT ( 'NONE',  ( -5.359611314223446995E-15, 29.16686587814335496, 142.8750000027311842 ) ) ;
#55774=EDGE_CURVE ( 'NONE', #80486, #9032, #32574, .T. ) ;
#55821=CARTESIAN_POINT ( 'NONE',  ( -22.44159573604009950, -16.30477369853688430, 141.5750000027311728 ) ) ;
#55824=CARTESIAN_POINT ( 'NONE',  ( -3.573655867282028392E-15, 2.428612866367529932E-14, 2.000000000000000000 ) ) ;
#55895=CARTESIAN_POINT ( 'NONE',  ( 23.48529157249599919, 32.32473071737754111, -10.44999999453762385 ) ) ;
#55897=AXIS2_PLACEMENT_3D ( 'NONE', #103724, #177581, #87546 ) ;
#55905=ORIENTED_EDGE ( 'NONE', *, *, #108503, .F. ) ;
#55931=CARTESIAN_POINT ( 'NONE',  ( 31.34393194264161053, 5.972569355670986901, 99.56318414118018723 ) ) ;
#55946=CARTESIAN_POINT ( 'NONE',  ( 36.85386064174074505, 2.754345082724624749, 49.76404540304363167 ) ) ;
#55949=CARTESIAN_POINT ( 'NONE',  ( -34.57969012852956325, -4.582005219005604424, 50.95785156492173940 ) ) ;
#55978=CARTESIAN_POINT ( 'NONE',  ( -36.89064505505186986, 5.462148823192606528, 44.26314855211814603 ) ) ;
#56059=CARTESIAN_POINT ( 'NONE',  ( -31.33330333603525375, 7.497710212630239290, 94.47580324309011246 ) ) ;
#56069=AXIS2_PLACEMENT_3D ( 'NONE', #150836, #100315, #193344 ) ;
#56101=CARTESIAN_POINT ( 'NONE',  ( -23.48529157249600985, 32.32473071737754111, -2.299999999999999822 ) ) ;
#56198=ORIENTED_EDGE ( 'NONE', *, *, #176051, .F. ) ;
#56222=CARTESIAN_POINT ( 'NONE',  ( 28.82186960331498327, 9.364793116373570925, 143.0999999999999659 ) ) ;
#56324=EDGE_CURVE ( 'NONE', #129957, #21601, #3219, .T. ) ;
#56433=CARTESIAN_POINT ( 'NONE',  ( -8.906447517083053711, -27.41122689804191026, 144.4000000000000057 ) ) ;
#56461=CARTESIAN_POINT ( 'NONE',  ( -29.86685920354755197, -21.69954338932560134, -10.42499999726881299 ) ) ;
#56484=CARTESIAN_POINT ( 'NONE',  ( -34.51210051733097828, 7.446700168151136445, 43.98226744806001420 ) ) ;
#56539=DIRECTION ( 'NONE',  ( 0.000000000000000000, 0.000000000000000000, 1.000000000000000000 ) ) ;
#56569=CARTESIAN_POINT ( 'NONE',  ( -23.48298174826589602, -32.32155151706772500, -3.702157773949823039 ) ) ;
#56587=DIRECTION ( 'NONE',  ( -1.000000000000000000, 0.000000000000000000, 0.000000000000000000 ) ) ;
#56681=VERTEX_POINT ( 'NONE', #26142 ) ;
#56713=CARTESIAN_POINT ( 'NONE',  ( 3.556970738554033499E-15, -38.81732327939057825, -2.624999997268812724 ) ) ;
#56720=CARTESIAN_POINT ( 'NONE',  ( -33.98208146068709112, -4.940236926081948532, 92.55634382532309701 ) ) ;
#56722=CARTESIAN_POINT ( 'NONE',  ( -9.776814272916249493, -36.00870872231931230, -7.999999999999998224 ) ) ;
#56733=DIRECTION ( 'NONE',  ( 0.000000000000000000, 0.000000000000000000, -1.000000000000000000 ) ) ;
#56735=CARTESIAN_POINT ( 'NONE',  ( 36.91746824999999177, 11.99521256947799230, -2.024999997268813523 ) ) ;
#56760=CARTESIAN_POINT ( 'NONE',  ( 27.73933785331498569, 2.768321779492822058E-14, 142.3750000027311842 ) ) ;
#56780=AXIS2_PLACEMENT_3D ( 'NONE', #136920, #180482, #106576 ) ;
#56793=CARTESIAN_POINT ( 'NONE',  ( -15.45904554457977653, 25.28215873741137898, 139.9235714043273617 ) ) ;
#56796=CARTESIAN_POINT ( 'NONE',  ( -31.99364916731038022, -5.510910596163089556E-15, 47.64999999999999147 ) ) ;
#56829=ORIENTED_EDGE ( 'NONE', *, *, #100974, .T. ) ;
#56830=CYLINDRICAL_SURFACE ( 'NONE', #56069, 28.82186960331498682 ) ;
#56832=CARTESIAN_POINT ( 'NONE',  ( -5.359611314223446995E-15, 29.16686587814335851, 140.8750000027311842 ) ) ;
#56874=CARTESIAN_POINT ( 'NONE',  ( 23.31738231874054534, 16.94106989632529192, 147.1999999999999886 ) ) ;
#56906=CARTESIAN_POINT ( 'NONE',  ( 29.86685920354754487, 21.69954338932564752, -1.924999997268813212 ) ) ;
#56945=CARTESIAN_POINT ( 'NONE',  ( 32.00000000000000000, -1.163414459189985801E-14, 95.00000000000000000 ) ) ;
#56957=CARTESIAN_POINT ( 'NONE',  ( 36.84755799831103928, 2.910846538911452619, 49.67009533327786386 ) ) ;
#56960=CARTESIAN_POINT ( 'NONE',  ( -34.38690502837285123, -7.455999864800775256, 45.95008414374198225 ) ) ;
#56999=CARTESIAN_POINT ( 'NONE',  ( 27.73933785331498925, -9.013057229001033122, 143.7750000027311614 ) ) ;
#57009=ORIENTED_EDGE ( 'NONE', *, *, #152340, .T. ) ;
#57074=CARTESIAN_POINT ( 'NONE',  ( -8.906447517083053711, -27.41122689804191026, 146.4000000000000057 ) ) ;
#57116=CARTESIAN_POINT ( 'NONE',  ( 11.74264578624800315, -36.14014761921581709, -7.400000000000000355 ) ) ;
#57160=VERTEX_POINT ( 'NONE', #117128 ) ;
#57191=APPLICATION_CONTEXT ( 'automotive_design' ) ;
#57236=CARTESIAN_POINT ( 'NONE',  ( 23.31738231874054534, 16.94106989632529192, 145.1999999999999886 ) ) ;
#57298=VERTEX_POINT ( 'NONE', #195999 ) ;
#57353=CARTESIAN_POINT ( 'NONE',  ( -33.85315667487628133, 2.014031266883448522E-14, 100.5000000000010232 ) ) ;
#57440=CARTESIAN_POINT ( 'NONE',  ( -17.96519593369847101, 33.31065106363013228, -7.999999999999994671 ) ) ;
#57443=CARTESIAN_POINT ( 'NONE',  ( -3.573655867282028392E-15, 2.428612866367529932E-14, 150.0000000000000000 ) ) ;
#57470=CARTESIAN_POINT ( 'NONE',  ( 17.14385361876520264, 23.59649016807275856, 148.6750000027311387 ) ) ;
#57632=( BOUNDED_CURVE ( )  B_SPLINE_CURVE ( 2, ( #181629, #43109, #28948, #117957, #86608, #9785, #116943, #87605, #135134, #120923, #165465 ),
 .UNSPECIFIED., .F., .T. ) 
 B_SPLINE_CURVE_WITH_KNOTS ( ( 3, 2, 2, 2, 2, 3 ),
 ( 0.9000000000000000222, 0.9200000000000000400, 0.9399999999999999467, 0.9599999999999999645, 0.9799999999999999822, 1.000000000000000000 ),
 .UNSPECIFIED. ) 
 CURVE ( )  GEOMETRIC_REPRESENTATION_ITEM ( )  RATIONAL_B_SPLINE_CURVE ( ( 1.000000000000000000, 0.9510565162951535312, 1.000000000000000000, 0.9510565162951535312, 1.000000000000000000, 0.9510565162951535312, 1.000000000000000000, 0.9510565162951535312, 1.000000000000000000, 0.9510565162951535312, 1.000000000000000000 ) ) 
 REPRESENTATION_ITEM ( '' )  );
#57714=CARTESIAN_POINT ( 'NONE',  ( -29.86685920354755552, 21.69954338932564397, -3.324999997268813345 ) ) ;
#57720=CARTESIAN_POINT ( 'NONE',  ( -34.29482437030765851, -3.353353130260861015, 90.62592007927790405 ) ) ;
#57721=CARTESIAN_POINT ( 'NONE',  ( -37.83797858686578053, -3.323448926770519840, -8.000000000000000000 ) ) ;
#57733=CARTESIAN_POINT ( 'NONE',  ( -5.950531402560715689E-15, 38.81732327939063509, -3.624999997268813168 ) ) ;
#57759=CARTESIAN_POINT ( 'NONE',  ( 22.44159573604009239, 16.30477369853692693, 140.5750000027311728 ) ) ;
#57790=DIRECTION ( 'NONE',  ( 1.000000000000000000, 0.000000000000000000, 0.000000000000000000 ) ) ;
#57826=ORIENTED_EDGE ( 'NONE', *, *, #146342, .F. ) ;
#57843=VECTOR ( 'NONE', #37533, 1000.000000000000000 ) ;
#57868=LINE ( 'NONE', #119540, #34101 ) ;
#57903=CARTESIAN_POINT ( 'NONE',  ( -30.74264578624800492, 22.33583958711400186, -9.949999994537627401 ) ) ;
#57958=CARTESIAN_POINT ( 'NONE',  ( -34.37447276284162001, -6.948158515131154012, 47.85536288891452728 ) ) ;
#57987=CARTESIAN_POINT ( 'NONE',  ( -36.95577132204472548, 5.312067825339672034, 43.56319566887930250 ) ) ;
#57994=FACE_OUTER_BOUND ( 'NONE', #133947, .T. ) ;
#57999=CARTESIAN_POINT ( 'NONE',  ( -17.14385361876520619, 23.59649016807275856, 142.5750000027312012 ) ) ;
#58107=CARTESIAN_POINT ( 'NONE',  ( -30.74264578624800492, -22.33583958711396278, -3.799999999999999822 ) ) ;
#58113=DIRECTION ( 'NONE',  ( -8.551662891793917213E-31, 1.000000000000000000, 1.224646799147353207E-16 ) ) ;
#58154=ORIENTED_EDGE ( 'NONE', *, *, #59414, .F. ) ;
#58240=ORIENTED_EDGE ( 'NONE', *, *, #55774, .F. ) ;
#58333=ORIENTED_EDGE ( 'NONE', *, *, #197168, .F. ) ;
#58420=CARTESIAN_POINT ( 'NONE',  ( -9.446479005521629446, 36.53641634556310436, -7.999999999999998224 ) ) ;
#58423=DIRECTION ( 'NONE',  ( 0.000000000000000000, 0.000000000000000000, -1.000000000000000000 ) ) ;
#58436=VERTEX_POINT ( 'NONE', #114894 ) ;
#58448=CARTESIAN_POINT ( 'NONE',  ( 17.14385361876520264, 23.59649016807275856, 142.6750000027311103 ) ) ;
#58450=DIRECTION ( 'NONE',  ( 0.000000000000000000, 0.000000000000000000, -1.000000000000000000 ) ) ;
#58551=CARTESIAN_POINT ( 'NONE',  ( -30.73962218707678318, -22.33364281372842441, -3.802157773949823127 ) ) ;
#58580=CARTESIAN_POINT ( 'NONE',  ( -30.73962218707678673, 22.33364281372846705, -2.202157773949823039 ) ) ;
#58662=CARTESIAN_POINT ( 'NONE',  ( -40.00200000000003087, -5.510910596163089556E-15, 45.00000000000000000 ) ) ;
#58686=CARTESIAN_POINT ( 'NONE',  ( 22.81625015709509441, 31.40387420917330275, -5.824999997268813345 ) ) ;
#58691=CARTESIAN_POINT ( 'NONE',  ( -31.69676786489883469, -20.43759221091016798, -7.999999999999998224 ) ) ;
#58703=CARTESIAN_POINT ( 'NONE',  ( -22.81625015709510507, 31.40387420917330275, -3.424999997268813434 ) ) ;
#58711=ORIENTED_EDGE ( 'NONE', *, *, #39318, .F. ) ;
#58712=EDGE_CURVE ( 'NONE', #155489, #128112, #186951, .T. ) ;
#58725=CARTESIAN_POINT ( 'NONE',  ( -31.71843943275784383, -0.9850135343614436767, 102.4512077271823784 ) ) ;
#58730=CARTESIAN_POINT ( 'NONE',  ( -8.571926809382601320, -26.38167802310801591, 139.7750000027311899 ) ) ;
#58812=DIRECTION ( 'NONE',  ( 0.000000000000000000, 0.000000000000000000, 1.000000000000000000 ) ) ;
#58814=EDGE_CURVE ( 'NONE', #90959, #142504, #91231, .T. ) ;
#58877=CARTESIAN_POINT ( 'NONE',  ( -38.00000000000000711, 2.428612866367529932E-14, -9.749999994537626336 ) ) ;
#58967=CARTESIAN_POINT ( 'NONE',  ( -8.571926809382608425, 26.38167802310805854, 148.4750000027311785 ) ) ;
#58972=CARTESIAN_POINT ( 'NONE',  ( -17.14385361876520264, -23.59649016807271593, 143.1750000027311671 ) ) ;
#58977=LINE ( 'NONE', #195531, #92914 ) ;
#59040=CARTESIAN_POINT ( 'NONE',  ( 1.993301997531345686E-15, -30.30510711980685556, 146.5000000000000284 ) ) ;
#59079=CARTESIAN_POINT ( 'NONE',  ( 3.766062262543149401E-15, -39.95556452105413570, -1.499999999999999778 ) ) ;
#59130=CARTESIAN_POINT ( 'NONE',  ( 34.57898328185100212, 4.579095689294076621, 50.94499274836910985 ) ) ;
#59198=CARTESIAN_POINT ( 'NONE',  ( 8.906447517083050158, 27.41122689804195645, 143.6500000054623740 ) ) ;
#59235=CIRCLE ( 'NONE', #33404, 2.649999999999992806 ) ;
#59237=VERTEX_POINT ( 'NONE', #17679 ) ;
#59312=ORIENTED_EDGE ( 'NONE', *, *, #169979, .F. ) ;
#59400=CARTESIAN_POINT ( 'NONE',  ( 1.160557336561849118, 37.56284411304923054, -8.000000000000003553 ) ) ;
#59414=EDGE_CURVE ( 'NONE', #117112, #43523, #179280, .T. ) ;
#59432=CARTESIAN_POINT ( 'NONE',  ( -27.73933785331498925, 2.428612866367529932E-14, 141.3750000027311842 ) ) ;
#59456=CARTESIAN_POINT ( 'NONE',  ( -28.82186960331499037, 2.428612866367529932E-14, 148.2500000054623683 ) ) ;
#59517=DIRECTION ( 'NONE',  ( 1.000000000000000000, 0.000000000000000000, 0.000000000000000000 ) ) ;
#59530=CARTESIAN_POINT ( 'NONE',  ( -37.99626262588766679, 2.428612866367529932E-14, -4.002157773949823749 ) ) ;
#59563=CIRCLE ( 'NONE', #188760, 29.43349580481983807 ) ;
#59600=CIRCLE ( 'NONE', #88624, 5.500000000000032863 ) ;
#59642=EDGE_LOOP ( 'NONE', ( #93786, #8255, #195780, #107132 ) ) ;
#59675=CARTESIAN_POINT ( 'NONE',  ( -11.40812507854755609, 35.11059874428196537, -1.024999997268813301 ) ) ;
#59681=CARTESIAN_POINT ( 'NONE',  ( 33.90110335395769425, 5.206480924673163813, 93.21819085016215922 ) ) ;
#59745=AXIS2_PLACEMENT_3D ( 'NONE', #176310, #80289, #6429 ) ;
#59769=CARTESIAN_POINT ( 'NONE',  ( -17.81289503416611097, -24.51734667627696496, 142.5500000054623513 ) ) ;
#59844=EDGE_CURVE ( 'NONE', #64642, #163891, #71153, .T. ) ;
#59868=CARTESIAN_POINT ( 'NONE',  ( 22.81625015709510151, -31.40387420917324590, -6.424999997268812102 ) ) ;
#59918=CARTESIAN_POINT ( 'NONE',  ( 36.89613260305527120, 1.429147721188409825, 50.32345767270687986 ) ) ;
#59945=EDGE_CURVE ( 'NONE', #136632, #150593, #88483, .T. ) ;
#59951=CARTESIAN_POINT ( 'NONE',  ( -36.84755799831103928, 2.910846538911445069, 49.67009533327788517 ) ) ;
#59957=CARTESIAN_POINT ( 'NONE',  ( 27.73933785331498214, 9.013057229001095294, 143.9750000027312069 ) ) ;
#59963=CARTESIAN_POINT ( 'NONE',  ( -27.73933785331498925, 9.013057229001089965, 146.7750000027312183 ) ) ;
#60035=CARTESIAN_POINT ( 'NONE',  ( -8.571926809382608425, 26.38167802310805854, 148.9750000027311785 ) ) ;
#60038=DIRECTION ( 'NONE',  ( 0.000000000000000000, 0.000000000000000000, 1.000000000000000000 ) ) ;
#60057=CARTESIAN_POINT ( 'NONE',  ( -40.00200000000003087, -1.163414459189985801E-14, 95.00000000000000000 ) ) ;
#60125=CARTESIAN_POINT ( 'NONE',  ( 34.54575687042838439, 4.960469055748728984, 50.63070180855212499 ) ) ;
#60174=AXIS2_PLACEMENT_3D ( 'NONE', #76743, #199104, #61566 ) ;
#60180=VERTEX_POINT ( 'NONE', #170116 ) ;
#60305=VERTEX_POINT ( 'NONE', #44795 ) ;
#60310=CARTESIAN_POINT ( 'NONE',  ( -11.40812507854754720, -35.11059874428192273, -4.224999997268813701 ) ) ;
#60326=AXIS2_PLACEMENT_3D ( 'NONE', #79533, #141203, #184730 ) ;
#60352=EDGE_CURVE ( 'NONE', #33122, #171099, #24744, .T. ) ;
#60424=CARTESIAN_POINT ( 'NONE',  ( -8.571926809382608425, 26.38167802310805854, 144.9750000027312069 ) ) ;
#60447=CARTESIAN_POINT ( 'NONE',  ( 1.993301997531345292E-15, -30.30510711980685912, 146.7500000054623683 ) ) ;
#60474=DIRECTION ( 'NONE',  ( 0.000000000000000000, 0.000000000000000000, -1.000000000000000000 ) ) ;
#60500=VECTOR ( 'NONE', #127271, 1000.000000000000000 ) ;
#60581=VERTEX_POINT ( 'NONE', #76110 ) ;
#60619=DIRECTION ( 'NONE',  ( 0.000000000000000000, 0.000000000000000000, 1.000000000000000000 ) ) ;
#60628=ORIENTED_EDGE ( 'NONE', *, *, #178712, .F. ) ;
#60663=CARTESIAN_POINT ( 'NONE',  ( 29.86685920354754842, -21.69954338932559068, -8.324999997268813345 ) ) ;
#60669=CARTESIAN_POINT ( 'NONE',  ( 33.68458106784984096, 5.328653173427194467, 96.40873914273848300 ) ) ;
#60707=CARTESIAN_POINT ( 'NONE',  ( 17.14385361876520264, 23.59649016807275856, 140.6750000027311387 ) ) ;
#60769=CARTESIAN_POINT ( 'NONE',  ( -31.68669428337296523, 6.716517432552113753, 91.65365426639641555 ) ) ;
#60852=CARTESIAN_POINT ( 'NONE',  ( -36.91746825000001309, -11.99521256947794789, -9.024999997268812635 ) ) ;
#60863=EDGE_LOOP ( 'NONE', ( #58240, #18043, #101781, #150464, #91050, #34002, #161140, #78137, #100690, #187021, #140295, #88288 ) ) ;
#60925=VERTEX_POINT ( 'NONE', #125602 ) ;
#60944=CARTESIAN_POINT ( 'NONE',  ( -22.44159573604010305, 16.30477369853692338, 144.6750000027311671 ) ) ;
#60949=CARTESIAN_POINT ( 'NONE',  ( -8.571926809382601320, -26.38167802310801591, 145.2750000027311899 ) ) ;
#60952=ORIENTED_EDGE ( 'NONE', *, *, #106236, .T. ) ;
#60978=EDGE_CURVE ( 'NONE', #96409, #89861, #143745, .T. ) ;
#60986=VERTEX_POINT ( 'NONE', #175092 ) ;
#61059=CARTESIAN_POINT ( 'NONE',  ( 38.00000000000000711, -12.34694845685040754, -9.100000000000001421 ) ) ;
#61110=CARTESIAN_POINT ( 'NONE',  ( 34.71410084532069362, 2.653616468751211155, 52.01918243487461524 ) ) ;
#61157=ORIENTED_EDGE ( 'NONE', *, *, #169870, .F. ) ;
#61161=FACE_OUTER_BOUND ( 'NONE', #196633, .T. ) ;
#61303=CARTESIAN_POINT ( 'NONE',  ( -29.86685920354755552, 21.69954338932564397, -4.824999997268814234 ) ) ;
#61387=CARTESIAN_POINT ( 'NONE',  ( -37.58407650405590061, -0.3597885541503507145, 39.49999999999997158 ) ) ;
#61418=CARTESIAN_POINT ( 'NONE',  ( 17.14385361876520264, -23.59649016807271238, 144.0750000027311444 ) ) ;
#61441=CARTESIAN_POINT ( 'NONE',  ( -35.70266437024450568, -5.510913496957479854E-15, 37.50000000000000000 ) ) ;
#61460=PLANE ( 'NONE',  #64089 ) ;
#61507=CARTESIAN_POINT ( 'NONE',  ( -37.99626262588766679, 2.428612866367529932E-14, -1.747842220587805251 ) ) ;
#61531=CARTESIAN_POINT ( 'NONE',  ( -27.73933785331498925, -9.013057229001049109, 142.9750000027312069 ) ) ;
#61548=CARTESIAN_POINT ( 'NONE',  ( -37.99626262588769521, 12.34573411038911317, -6.102157773949821618 ) ) ;
#61566=DIRECTION ( 'NONE',  ( 1.000000000000000000, 0.000000000000000000, 0.000000000000000000 ) ) ;
#61576=ORIENTED_EDGE ( 'NONE', *, *, #72314, .T. ) ;
#61627=CYLINDRICAL_SURFACE ( 'NONE', #12202, 28.82186960331498682 ) ;
#61653=CARTESIAN_POINT ( 'NONE',  ( -5.950531402560715689E-15, 38.81732327939063509, -9.624999997268815832 ) ) ;
#61656=CARTESIAN_POINT ( 'NONE',  ( 11.74149087413295156, -36.13659316521243881, -3.147842220587803386 ) ) ;
#61671=CARTESIAN_POINT ( 'NONE',  ( 32.44846625821359254, 18.14626611352247210, -7.961615373864755263 ) ) ;
#61681=DIRECTION ( 'NONE',  ( 0.000000000000000000, 0.000000000000000000, -1.000000000000000000 ) ) ;
#61735=CARTESIAN_POINT ( 'NONE',  ( -17.81289503416611808, 24.51734667627700404, 141.6999999999999602 ) ) ;
#61745=CARTESIAN_POINT ( 'NONE',  ( 28.82186960331486958, -9.364793116373689941, 143.1500000054623740 ) ) ;
#61756=CARTESIAN_POINT ( 'NONE',  ( -31.37700036491433053, 7.446261808816053041, 93.97872476790939800 ) ) ;
#61840=CARTESIAN_POINT ( 'NONE',  ( -29.86685920354755552, 21.69954338932564397, -5.324999997268814234 ) ) ;
#61842=EDGE_CURVE ( 'NONE', #82818, #31542, #64110, .T. ) ;
#61885=LINE ( 'NONE', #44752, #74009 ) ;
#61931=CARTESIAN_POINT ( 'NONE',  ( 27.73933785331498925, -9.013057229001033122, 147.7750000027311899 ) ) ;
#61946=ORIENTED_EDGE ( 'NONE', *, *, #171253, .F. ) ;
#62047=CARTESIAN_POINT ( 'NONE',  ( -38.00000000000001421, -12.34694845685042708, -7.900000000000001243 ) ) ;
#62082=( BOUNDED_CURVE ( )  B_SPLINE_CURVE ( 2, ( #167977, #1088, #155779, #152795, #78930 ),
 .UNSPECIFIED., .F., .T. ) 
 B_SPLINE_CURVE_WITH_KNOTS ( ( 3, 2, 3 ),
 ( 0.8000000000000007105, 0.8200000000000000622, 0.8250928956683720727 ),
 .UNSPECIFIED. ) 
 CURVE ( )  GEOMETRIC_REPRESENTATION_ITEM ( )  RATIONAL_B_SPLINE_CURVE ( ( 0.9999999999999983347, 0.9510565162951551965, 1.000000000000000000, 0.9875367971922273114, 0.9814209735438295112 ) ) 
 REPRESENTATION_ITEM ( '' )  );
#62099=CARTESIAN_POINT ( 'NONE',  ( 35.68624576866247367, 0.9837712456776031011, 37.56068211393102274 ) ) ;
#62286=CARTESIAN_POINT ( 'NONE',  ( -22.81625015709509441, -31.40387420917324590, -4.324999997268812457 ) ) ;
#62290=B_SPLINE_CURVE_WITH_KNOTS ( 'NONE', 3,
 ( #132196, #54358, #53351, #82675, #116030, #128192, #177719, #39187, #162527, #114009, #36181, #66529, #159523, #173733, #24030, #190877, #85684, #67522, #189890, #50385, #52353, #51365, #175707, #158539, #113026, #97835, #21020, #41197, #166544, #44185, #86685, #179727, #71523, #133190, #55352, #28042, #195896, #11878, #102859, #181705 ),
 .UNSPECIFIED., .F., .F.,
 ( 4, 2, 2, 2, 2, 2, 2, 2, 2, 2, 2, 2, 2, 2, 2, 2, 2, 2, 2, 4 ),
 ( 0.02146664961600480703, 0.02254346109514431332, 0.02362027257428381960, 0.02415867831385357795, 0.02469708405342333629, 0.02577389553256286339, 0.02685070701170239049, 0.02738911275127214884, 0.02792751849084190024, 0.02900432996998139265, 0.03008114144912088506, 0.03115795292826037746, 0.03223476440739986987, 0.03331157588653935880, 0.03438838736567885468, 0.03546519884481834362, 0.03600360458438808114, 0.03654201032395781867, 0.03761882180309729373, 0.03869563328223677573 ),
 .UNSPECIFIED. ) ;
#62328=EDGE_LOOP ( 'NONE', ( #92976, #89479, #28260, #33012, #118927, #39501, #199514, #130455, #59312, #52331, #84253, #24649 ) ) ;
#62376=CARTESIAN_POINT ( 'NONE',  ( -37.24135263299452703, -4.142047767899336819, 41.36355589474229788 ) ) ;
#62379=CARTESIAN_POINT ( 'NONE',  ( -28.82186960331514669, -9.364793116373306248, 144.0999999999999659 ) ) ;
#62407=CARTESIAN_POINT ( 'NONE',  ( -27.73933785331498925, 9.013057229001089965, 147.2750000027311614 ) ) ;
#62431=CARTESIAN_POINT ( 'NONE',  ( -8.906447517083060816, 27.41122689804195645, 143.8500000054623911 ) ) ;
#62457=AXIS2_PLACEMENT_3D ( 'NONE', #135298, #184765, #92737 ) ;
#62523=CARTESIAN_POINT ( 'NONE',  ( 17.14385361876520264, 23.59649016807275856, 144.1750000027311671 ) ) ;
#62543=CARTESIAN_POINT ( 'NONE',  ( -23.48298174826590667, 32.32155151706776053, -6.302157773949822683 ) ) ;
#62649=CARTESIAN_POINT ( 'NONE',  ( 36.91746824999999177, 2.880721459617395097E-14, -1.624999997268813390 ) ) ;
#62665=CARTESIAN_POINT ( 'NONE',  ( -11.40812507854755609, 35.11059874428196537, -7.524999997268813523 ) ) ;
#62737=( GEOMETRIC_REPRESENTATION_CONTEXT ( 3 ) GLOBAL_UNCERTAINTY_ASSIGNED_CONTEXT ( ( #130795 ) ) GLOBAL_UNIT_ASSIGNED_CONTEXT ( ( #151754, #106229, #163949 ) ) REPRESENTATION_CONTEXT ( 'NONE', 'WORKASPACE' ) );
#62753=CARTESIAN_POINT ( 'NONE',  ( -31.91717023173582746, 5.953136853522615013, 90.41250038490913710 ) ) ;
#62838=CARTESIAN_POINT ( 'NONE',  ( -36.91746825000001309, 11.99521256947798342, -5.224999997268811924 ) ) ;
#62930=CARTESIAN_POINT ( 'NONE',  ( -17.14385361876520619, 23.59649016807275856, 140.5750000027311728 ) ) ;
#62943=EDGE_LOOP ( 'NONE', ( #188880, #13305, #88527, #30306 ) ) ;
#62987=AXIS2_PLACEMENT_3D ( 'NONE', #162562, #7876, #97869 ) ;
#63028=CARTESIAN_POINT ( 'NONE',  ( 34.52594549653173317, 2.428612888752089207E-14, 89.49999999999897682 ) ) ;
#63101=AXIS2_PLACEMENT_3D ( 'NONE', #177276, #147929, #71081 ) ;
#63207=DIRECTION ( 'NONE',  ( -7.709882115452472644E-15, 0.000000000000000000, 1.000000000000000000 ) ) ;
#63242=CIRCLE ( 'NONE', #195651, 7.500000000000000000 ) ;
#63248=CYLINDRICAL_SURFACE ( 'NONE', #53306, 7.500000000000000000 ) ;
#63255=CARTESIAN_POINT ( 'NONE',  ( 30.00000000000000000, -1.163414459189985801E-14, 95.00000000000000000 ) ) ;
#63258=CARTESIAN_POINT ( 'NONE',  ( 33.83559363775140838, -1.430799499857053680, 100.3228003899268401 ) ) ;
#63292=CARTESIAN_POINT ( 'NONE',  ( -36.91746825000001309, 11.99521256947798342, -4.724999997268811924 ) ) ;
#63385=CARTESIAN_POINT ( 'NONE',  ( -37.52651979737520094, -1.772832052285354010, 39.78107084225509738 ) ) ;
#63417=CARTESIAN_POINT ( 'NONE',  ( -17.81289503416611808, 24.51734667627700404, 149.6999999999999602 ) ) ;
#63441=CARTESIAN_POINT ( 'NONE',  ( -17.81289503416611097, -24.51734667627696496, 144.5500000054623513 ) ) ;
#63499=VECTOR ( 'NONE', #107306, 1000.000000000000000 ) ;
#63505=ADVANCED_FACE ( 'NONE', ( #161678 ), #177865, .T. ) ;
#63535=CARTESIAN_POINT ( 'NONE',  ( -8.571926809382608425, 26.38167802310805854, 146.4750000027311785 ) ) ;
#63538=ORIENTED_EDGE ( 'NONE', *, *, #67479, .T. ) ;
#63616=CARTESIAN_POINT ( 'NONE',  ( 31.99364916731006048, 4.791014396527177230E-13, 45.00000000000022027 ) ) ;
#63641=CONICAL_SURFACE ( 'NONE', #47486, 40.00000000000002132, 0.06108652381980166773 ) ;
#63662=CARTESIAN_POINT ( 'NONE',  ( 36.91746824999999887, 11.99521256947799053, -8.024999997268814411 ) ) ;
#63667=CARTESIAN_POINT ( 'NONE',  ( 34.48736576873178450, 1.429538131128955669, 89.67663809442005629 ) ) ;
#63678=CARTESIAN_POINT ( 'NONE',  ( -29.86685920354755197, -21.69954338932560134, -6.924999997268813878 ) ) ;
#63712=CARTESIAN_POINT ( 'NONE',  ( 34.37447276284161291, -6.948158515131153123, 47.85536288891451306 ) ) ;
#63742=CARTESIAN_POINT ( 'NONE',  ( -28.82186960331499037, 2.428612866367529932E-14, 142.0000000000000000 ) ) ;
#63840=EDGE_CURVE ( 'NONE', #186418, #134298, #76530, .T. ) ;
#63847=LINE ( 'NONE', #18351, #103195 ) ;
#63851=CARTESIAN_POINT ( 'NONE',  ( -36.91746825000001309, -11.99521256947794789, -7.024999997268812635 ) ) ;
#63868=EDGE_LOOP ( 'NONE', ( #161094, #81760 ) ) ;
#63916=AXIS2_PLACEMENT_3D ( 'NONE', #177881, #8002, #134370 ) ;
#63939=CARTESIAN_POINT ( 'NONE',  ( -22.44159573604010305, 16.30477369853692338, 140.6750000027311671 ) ) ;
#63944=CARTESIAN_POINT ( 'NONE',  ( -27.73933785331498925, 2.428612866367529932E-14, 138.8750000027311842 ) ) ;
#64012=CARTESIAN_POINT ( 'NONE',  ( -17.14385361876520264, -23.59649016807271238, 143.6750000027311671 ) ) ;
#64057=CARTESIAN_POINT ( 'NONE',  ( -23.31738231874055600, 16.94106989632528837, 147.7999999999999829 ) ) ;
#64089=AXIS2_PLACEMENT_3D ( 'NONE', #198005, #137317, #1781 ) ;
#64110=B_SPLINE_CURVE_WITH_KNOTS ( 'NONE', 3,
 ( #84064, #148763, #72930, #119424, #116413, #70919, #179114, #23414, #85062, #146744, #164935, #69917, #54741, #181108, #178103, #39571, #42582, #192266, #162918, #104245, #71911, #22414, #117416, #88068, #53748, #163940, #24427, #115422, #55742, #133583, #102252, #118428, #180121, #41589, #26428, #139531, #43571, #153717, #168875, #74900, #93028, #154716, #184067, #44564, #152719, #58725, #197263, #30380 ),
 .UNSPECIFIED., .F., .F.,
 ( 4, 2, 2, 2, 2, 2, 2, 2, 2, 2, 2, 2, 2, 2, 2, 2, 2, 2, 2, 2, 2, 2, 2, 4 ),
 ( 0.04104976116627316596, 0.04252145193039927329, 0.04325729731246233389, 0.04399314269452538756, 0.04472898807658844123, 0.04546483345865150183, 0.04693652422277762998, 0.04840821498690375813, 0.04914406036896680485, 0.04987990575102985852, 0.05135159651515595197, 0.05208744189721900564, 0.05282328727928205236, 0.05429497804340815276, 0.05503082342547122030, 0.05576666880753428784, 0.05723835957166042293, 0.05871005033578655802, 0.05944589571784963944, 0.06018174109991272780, 0.06165343186403891840, 0.06238927724610200676, 0.06312512262816510900, 0.06459681339229128572 ),
 .UNSPECIFIED. ) ;
#64227=DIRECTION ( 'NONE',  ( 1.000000000000000000, 0.000000000000000000, 0.000000000000000000 ) ) ;
#64262=CARTESIAN_POINT ( 'NONE',  ( 34.40553910806574578, -2.436532241128160692, 90.06585364601157551 ) ) ;
#64413=CARTESIAN_POINT ( 'NONE',  ( -5.429308488886486681E-15, 30.30510711980690175, 145.4999999999999432 ) ) ;
#64436=CARTESIAN_POINT ( 'NONE',  ( -17.14385361876520619, 23.59649016807275856, 148.5750000027311444 ) ) ;
#64449=ORIENTED_EDGE ( 'NONE', *, *, #178834, .T. ) ;
#64529=CARTESIAN_POINT ( 'NONE',  ( 22.44159573604009594, -16.30477369853687364, 141.6750000027311671 ) ) ;
#64642=VERTEX_POINT ( 'NONE', #159182 ) ;
#64654=CARTESIAN_POINT ( 'NONE',  ( -36.91746825000001309, 11.99521256947798342, -6.724999997268813701 ) ) ;
#64655=CARTESIAN_POINT ( 'NONE',  ( -33.84581411518095706, 5.355620490906736642, 93.73536670833321693 ) ) ;
#64707=CARTESIAN_POINT ( 'NONE',  ( 34.61318912441599593, -7.252276964307556639, 43.02678305251431823 ) ) ;
#64731=CARTESIAN_POINT ( 'NONE',  ( -3.573655867282028392E-15, 2.428612866367529932E-14, 0.000000000000000000 ) ) ;
#64765=FACE_BOUND ( 'NONE', #40802, .T. ) ;
#64920=ORIENTED_EDGE ( 'NONE', *, *, #179710, .T. ) ;
#64926=CARTESIAN_POINT ( 'NONE',  ( 27.73933785331498214, 9.013057229001095294, 148.4750000027311785 ) ) ;
#64931=CARTESIAN_POINT ( 'NONE',  ( 27.73933785331498214, 9.013057229001095294, 139.9750000027311501 ) ) ;
#64977=EDGE_CURVE ( 'NONE', #65515, #147006, #105547, .T. ) ;
#64998=CARTESIAN_POINT ( 'NONE',  ( 17.14385361876520264, 23.59649016807275856, 142.6750000027311103 ) ) ;
#65120=CARTESIAN_POINT ( 'NONE',  ( -3.573655867282028392E-15, 2.428612866367529932E-14, 2.000000000000000000 ) ) ;
#65158=CARTESIAN_POINT ( 'NONE',  ( -5.950531402560715689E-15, 38.81732327939063509, -3.124999997268813168 ) ) ;
#65203=CARTESIAN_POINT ( 'NONE',  ( -3.573655867282028392E-15, 2.428612866367529932E-14, 2.000000000000000000 ) ) ;
#65234=DIRECTION ( 'NONE',  ( 0.000000000000000000, 0.000000000000000000, -1.000000000000000000 ) ) ;
#65274=( BOUNDED_CURVE ( )  B_SPLINE_CURVE ( 2, ( #59530, #134415, #58551, #56569, #136387, #89885, #120217, #181907, #149570, #26243, #197084 ),
 .UNSPECIFIED., .F., .F. ) 
 B_SPLINE_CURVE_WITH_KNOTS ( ( 3, 2, 2, 2, 2, 3 ),
 ( 0.6000000000000000888, 0.6200000000000001066, 0.6400000000000001243, 0.6600000000000001421, 0.6800000000000001599, 0.7000000000000001776 ),
 .UNSPECIFIED. ) 
 CURVE ( )  GEOMETRIC_REPRESENTATION_ITEM ( )  RATIONAL_B_SPLINE_CURVE ( ( 0.9999999999999997780, 0.9510565162951537532, 1.000000000000000000, 0.9510565162951535312, 1.000000000000000000, 0.9510565162951535312, 1.000000000000000000, 0.9510565162951535312, 1.000000000000000000, 0.9510565162951529761, 1.000000000000000444 ) ) 
 REPRESENTATION_ITEM ( '' )  );
#65279=CARTESIAN_POINT ( 'NONE',  ( 11.40812507854755253, -35.11059874428192273, -10.02499999726881441 ) ) ;
#65369=CARTESIAN_POINT ( 'NONE',  ( 32.64453336272026718, -1.163414472736631538E-14, 87.50000000000000000 ) ) ;
#65398=CARTESIAN_POINT ( 'NONE',  ( 17.81289503416610742, 24.51734667627700404, 147.2999999999999545 ) ) ;
#65420=CARTESIAN_POINT ( 'NONE',  ( 8.906447517083050158, 27.41122689804195645, 139.6500000054623740 ) ) ;
#65474=ORIENTED_EDGE ( 'NONE', *, *, #53439, .F. ) ;
#65512=CARTESIAN_POINT ( 'NONE',  ( 22.44159573604009239, 16.30477369853692693, 144.0750000027311728 ) ) ;
#65515=VERTEX_POINT ( 'NONE', #7498 ) ;
#65533=DIRECTION ( 'NONE',  ( -0.000000000000000000, -0.000000000000000000, -1.000000000000000000 ) ) ;
#65569=CARTESIAN_POINT ( 'NONE',  ( -28.82186960331499037, 2.428612866367529932E-14, 150.0000000000000000 ) ) ;
#65636=CARTESIAN_POINT ( 'NONE',  ( 3.556970738554033499E-15, -38.81732327939057825, -4.124999997268814056 ) ) ;
#65689=CARTESIAN_POINT ( 'NONE',  ( 35.31558682697088614, -4.577067960279664227, 39.03840433125808573 ) ) ;
#65731=EDGE_CURVE ( 'NONE', #83417, #131569, #196076, .T. ) ;
#65748=LINE ( 'NONE', #124441, #91402 ) ;
#65800=EDGE_CURVE ( 'NONE', #68554, #200018, #130350, .T. ) ;
#65875=CARTESIAN_POINT ( 'NONE',  ( -33.75684350552029400, -3.359699206722016385, 99.36933870599236229 ) ) ;
#65876=CARTESIAN_POINT ( 'NONE',  ( 6.154245480356221876, -36.53401430921382342, -8.000000000000003553 ) ) ;
#65914=CARTESIAN_POINT ( 'NONE',  ( -22.44159573604009950, -16.30477369853688430, 143.0750000027311728 ) ) ;
#65918=CARTESIAN_POINT ( 'NONE',  ( 8.571926809382603096, -26.38167802310801235, 139.4750000027311785 ) ) ;
#65951=ORIENTED_EDGE ( 'NONE', *, *, #92301, .F. ) ;
#65987=CARTESIAN_POINT ( 'NONE',  ( 27.73933785331498569, 2.768321779492822058E-14, 142.3750000027311842 ) ) ;
#66023=CIRCLE ( 'NONE', #101537, 2.699999999999993960 ) ;
#66036=PLANE ( 'NONE',  #126968 ) ;
#66066=CARTESIAN_POINT ( 'NONE',  ( 3.766062262543149401E-15, -39.95556452105413570, -3.249999994537627224 ) ) ;
#66098=ADVANCED_FACE ( 'NONE', ( #21201 ), #150742, .F. ) ;
#66116=CARTESIAN_POINT ( 'NONE',  ( 37.47229216401454011, 2.437641287457624095, 40.05669362136319478 ) ) ;
#66135=ADVANCED_FACE ( 'NONE', ( #143533 ), #5021, .T. ) ;
#66150=CARTESIAN_POINT ( 'NONE',  ( -11.40812507854755609, 35.11059874428196537, -7.024999997268813523 ) ) ;
#66184=( GEOMETRIC_REPRESENTATION_CONTEXT ( 3 ) GLOBAL_UNCERTAINTY_ASSIGNED_CONTEXT ( ( #98449 ) ) GLOBAL_UNIT_ASSIGNED_CONTEXT ( ( #130067, #114927, #100746 ) ) REPRESENTATION_CONTEXT ( 'NONE', 'WORKASPACE' ) );
#66188=CARTESIAN_POINT ( 'NONE',  ( -30.00000000000000000, -1.163414459189985801E-14, 95.00000000000000000 ) ) ;
#66241=CARTESIAN_POINT ( 'NONE',  ( 34.52594549653174028, -0.3594300054053903293, 89.49999999999896261 ) ) ;
#66275=CARTESIAN_POINT ( 'NONE',  ( -36.91746825000001309, -11.99521256947794789, -8.524999997268812635 ) ) ;
#66335=ORIENTED_EDGE ( 'NONE', *, *, #17662, .F. ) ;
#66395=CARTESIAN_POINT ( 'NONE',  ( 17.14385361876520264, 23.59649016807275856, 140.6750000027311387 ) ) ;
#66417=CARTESIAN_POINT ( 'NONE',  ( 22.44159573604009594, -16.30477369853687364, 147.6750000027311671 ) ) ;
#66443=CARTESIAN_POINT ( 'NONE',  ( -28.82186960331504721, -9.364793116373462567, 146.3500000054623911 ) ) ;
#66474=EDGE_CURVE ( 'NONE', #154069, #71503, #112034, .T. ) ;
#66527=DIRECTION ( 'NONE',  ( -0.06104853953485701173, -7.476289853398329258E-18, -0.9981347984218670311 ) ) ;
#66529=CARTESIAN_POINT ( 'NONE',  ( 36.79334119018157878, -4.151185298968582238, 48.62628996558957084 ) ) ;
#66628=CARTESIAN_POINT ( 'NONE',  ( -29.86685920354755552, 21.69954338932564397, -2.824999997268813345 ) ) ;
#66717=DIRECTION ( 'NONE',  ( 1.000000000000000000, 0.000000000000000000, 0.000000000000000000 ) ) ;
#66911=CARTESIAN_POINT ( 'NONE',  ( 17.14385361876520264, -23.59649016807271238, 148.0750000027311728 ) ) ;
#66983=VECTOR ( 'NONE', #126675, 1000.000000000000000 ) ;
#66987=CARTESIAN_POINT ( 'NONE',  ( 1.784210473542230573E-15, -29.16686587814331588, 143.8750000027311842 ) ) ;
#67034=CARTESIAN_POINT ( 'NONE',  ( 32.64453336272026718, -1.163414472736631538E-14, 87.50000000000000000 ) ) ;
#67065=CARTESIAN_POINT ( 'NONE',  ( 11.74264578624800315, -36.14014761921581709, -7.149999994537626691 ) ) ;
#67074=CARTESIAN_POINT ( 'NONE',  ( 32.00000000000000000, -1.163414459189985801E-14, 95.00000000000000000 ) ) ;
#67078=CARTESIAN_POINT ( 'NONE',  ( 35.70266437024449147, 2.428612576286966776E-14, 37.50000000000000000 ) ) ;
#67083=VECTOR ( 'NONE', #50771, 1000.000000000000000 ) ;
#67116=CARTESIAN_POINT ( 'NONE',  ( 36.91746824999999887, 11.99521256947799053, -6.024999997268811747 ) ) ;
#67148=CARTESIAN_POINT ( 'NONE',  ( 36.91746824999999177, 11.99521256947799230, -1.524999997268813523 ) ) ;
#67233=CARTESIAN_POINT ( 'NONE',  ( 33.73406392173259150, -5.500497537618388222, 95.16330145977877919 ) ) ;
#67266=CARTESIAN_POINT ( 'NONE',  ( 11.40812507854754365, 35.11059874428196537, -9.224999997268813701 ) ) ;
#67309=ORIENTED_EDGE ( 'NONE', *, *, #30819, .F. ) ;
#67356=CARTESIAN_POINT ( 'NONE',  ( 31.91599925174810792, -5.957486376704251185, 90.41819350476903594 ) ) ;
#67387=CARTESIAN_POINT ( 'NONE',  ( 17.81289503416611453, -24.51734667627695785, 148.6999999999999602 ) ) ;
#67410=CARTESIAN_POINT ( 'NONE',  ( 28.82186960331498327, 2.781578969918950771E-14, 139.2500000054623683 ) ) ;
#67479=EDGE_CURVE ( 'NONE', #38003, #60305, #53428, .T. ) ;
#67503=CARTESIAN_POINT ( 'NONE',  ( -5.359611314223446995E-15, 29.16686587814335851, 140.3750000027311842 ) ) ;
#67518=CARTESIAN_POINT ( 'NONE',  ( -28.82186960331499037, 2.428612866367529932E-14, 148.0000000000000000 ) ) ;
#67520=PLANE ( 'NONE',  #169145 ) ;
#67522=CARTESIAN_POINT ( 'NONE',  ( 36.77116682341763010, -5.223593267096956261, 46.75914592492880217 ) ) ;
#67549=EDGE_LOOP ( 'NONE', ( #84079, #163146, #154002 ) ) ;
#67623=CARTESIAN_POINT ( 'NONE',  ( 36.91746824999999887, 11.99521256947799053, -7.524999997268814411 ) ) ;
#67624=CARTESIAN_POINT ( 'NONE',  ( -33.74157273865942130, 3.640299887980672722, 99.13851753912355491 ) ) ;
#67682=CARTESIAN_POINT ( 'NONE',  ( 35.41276914313061752, -3.966036006072659603, 38.62970943314351757 ) ) ;
#67683=EDGE_LOOP ( 'NONE', ( #162996, #169034, #56829, #75921 ) ) ;
#67701=CARTESIAN_POINT ( 'NONE',  ( -3.573655867282028392E-15, 2.428612866367529932E-14, -0.1220970790697140096 ) ) ;
#67868=CARTESIAN_POINT ( 'NONE',  ( 37.99626262588765258, 2.893932880411085066E-14, 2.000000000000000000 ) ) ;
#67874=FACE_OUTER_BOUND ( 'NONE', #159501, .T. ) ;
#67911=CARTESIAN_POINT ( 'NONE',  ( 27.73933785331498925, -9.013057229001033122, 146.2750000027311899 ) ) ;
#67943=CARTESIAN_POINT ( 'NONE',  ( 30.00000000000000711, -1.163414459189985801E-14, 95.00000000000000000 ) ) ;
#67981=CARTESIAN_POINT ( 'NONE',  ( -22.44159573604009950, -16.30477369853688430, 143.5750000027311728 ) ) ;
#68058=CARTESIAN_POINT ( 'NONE',  ( -23.48529157249599919, -32.32473071737750558, -5.449999994537626513 ) ) ;
#68068=DIRECTION ( 'NONE',  ( 0.000000000000000000, 0.000000000000000000, -1.000000000000000000 ) ) ;
#68071=VERTEX_POINT ( 'NONE', #193964 ) ;
#68080=EDGE_CURVE ( 'NONE', #136632, #113568, #101935, .T. ) ;
#68093=EDGE_CURVE ( 'NONE', #113568, #60986, #118697, .T. ) ;
#68094=CARTESIAN_POINT ( 'NONE',  ( 32.64453336272026718, -1.163414472736631538E-14, 87.50000000000000000 ) ) ;
#68109=CARTESIAN_POINT ( 'NONE',  ( 11.40812507854755253, -35.11059874428192273, -2.524999997268813523 ) ) ;
#68140=CARTESIAN_POINT ( 'NONE',  ( 36.91746824999999177, 11.99521256947799230, -5.524999997268812635 ) ) ;
#68243=B_SPLINE_CURVE_WITH_KNOTS ( 'NONE', 3,
 ( #54432, #165611, #87752, #100916, #86759, #41268, #57440, #12924, #194953, #39260, #147446, #58420, #193961, #162601, #88756, #70603, #59400, #27110, #120087, #164615, #89751, #134280, #74588, #136256, #117095, #150449, #102930, #26109, #197932, #119113, #24105, #103931, #177790, #85759, #195968, #42273, #8934, #132270, #179799, #178790, #55424, #40259 ),
 .UNSPECIFIED., .F., .F.,
 ( 4, 2, 2, 2, 2, 2, 2, 2, 2, 2, 2, 2, 2, 2, 2, 2, 2, 2, 2, 2, 4 ),
 ( 0.0002562179899358165238, 0.004844394232870628293, 0.009432570475805439683, 0.01172665859727284841, 0.01402074671874025888, 0.01860892296167508675, 0.02319709920460991115, 0.02778527544754473902, 0.03237345169047955995, 0.03466753981194697909, 0.03696162793341439129, 0.04154980417634921569, 0.04384389229781662095, 0.04613798041928402621, 0.05072615666221883673, 0.05302024478368623506, 0.05531433290515364032, 0.05990250914808845084, 0.06449068539102326136, 0.06907886163395808576, 0.07366703787689289629 ),
 .UNSPECIFIED. ) ;
#68261=CARTESIAN_POINT ( 'NONE',  ( -11.40812507854755609, 35.11059874428196537, -9.024999997268814411 ) ) ;
#68381=CARTESIAN_POINT ( 'NONE',  ( -28.82186960331499037, 2.428612866367529932E-14, 144.0000000000000000 ) ) ;
#68404=CARTESIAN_POINT ( 'NONE',  ( 17.81289503416610742, 24.51734667627700404, 139.5500000054623229 ) ) ;
#68419=EDGE_CURVE ( 'NONE', #116580, #111465, #28109, .T. ) ;
#68498=CARTESIAN_POINT ( 'NONE',  ( 27.73933785331498569, 2.768321779492822058E-14, 139.8750000027311842 ) ) ;
#68513=CARTESIAN_POINT ( 'NONE',  ( 17.81289503416611453, -24.51734667627695785, 148.6999999999999602 ) ) ;
#68554=VERTEX_POINT ( 'NONE', #133265 ) ;
#68618=CARTESIAN_POINT ( 'NONE',  ( 17.14385361876520264, -23.59649016807271238, 148.0750000027311728 ) ) ;
#68656=EDGE_CURVE ( 'NONE', #64642, #80486, #28222, .T. ) ;
#68738=CARTESIAN_POINT ( 'NONE',  ( -3.573655867282028392E-15, 2.428612866367529932E-14, -8.000000000000000000 ) ) ;
#68776=EDGE_CURVE ( 'NONE', #114881, #24708, #8850, .T. ) ;
#68819=CARTESIAN_POINT ( 'NONE',  ( -23.48298174826589602, -32.32155151706772500, -5.702157773949823039 ) ) ;
#68826=CARTESIAN_POINT ( 'NONE',  ( 36.85948423281453046, 2.394443620734153289, -8.000000000000001776 ) ) ;
#68836=ORIENTED_EDGE ( 'NONE', *, *, #104283, .T. ) ;
#68874=CARTESIAN_POINT ( 'NONE',  ( -33.80700117934221538, -2.275881256356159010, 100.0103016164005112 ) ) ;
#68886=VERTEX_POINT ( 'NONE', #10936 ) ;
#68913=CARTESIAN_POINT ( 'NONE',  ( 8.571926809382603096, -26.38167802310801235, 141.9750000027312069 ) ) ;
#68918=CARTESIAN_POINT ( 'NONE',  ( 37.99626262588765258, 2.893932880411085066E-14, -4.747842220587804363 ) ) ;
#68986=CARTESIAN_POINT ( 'NONE',  ( 27.73933785331498569, 9.013057229001093518, 140.4750000027312069 ) ) ;
#69017=EDGE_CURVE ( 'NONE', #59237, #57160, #69403, .T. ) ;
#69062=CARTESIAN_POINT ( 'NONE',  ( -30.74264578624800492, -22.33583958711396278, -5.549999994537627046 ) ) ;
#69096=CARTESIAN_POINT ( 'NONE',  ( 32.15509708611484996, 4.949069787320328651, 89.34338315600291480 ) ) ;
#69110=DIRECTION ( 'NONE',  ( 1.000000000000000000, 0.000000000000000000, 3.709348145883536076E-20 ) ) ;
#69114=CARTESIAN_POINT ( 'NONE',  ( -34.67225235875025646, -7.109416101192573834, 42.56171885070867944 ) ) ;
#69143=CARTESIAN_POINT ( 'NONE',  ( -36.91746825000000598, 11.99521256947798520, -2.724999997268813701 ) ) ;
#69212=VECTOR ( 'NONE', #141444, 1000.000000000000000 ) ;
#69229=PLANE ( 'NONE',  #69794 ) ;
#69267=CARTESIAN_POINT ( 'NONE',  ( -22.81625015709509441, -31.40387420917324590, -6.324999997268815122 ) ) ;
#69356=CARTESIAN_POINT ( 'NONE',  ( 23.48298174826589246, 32.32155151706776053, -6.447842220587803652 ) ) ;
#69386=CARTESIAN_POINT ( 'NONE',  ( 17.81289503416611453, -24.51734667627695785, 142.6999999999999886 ) ) ;
#69397=EDGE_CURVE ( 'NONE', #157920, #136724, #186529, .T. ) ;
#69403=( BOUNDED_CURVE ( )  B_SPLINE_CURVE ( 2, ( #177793, #85762, #117098, #178793, #9940, #194956, #56433, #118113, #156393, #62379, #182771 ),
 .UNSPECIFIED., .F., .T. ) 
 B_SPLINE_CURVE_WITH_KNOTS ( ( 3, 2, 2, 2, 2, 3 ),
 ( 0.5000000000000004441, 0.5200000000000004619, 0.5400000000000004796, 0.5600000000000006084, 0.5800000000000005151, 0.6000000000000005329 ),
 .UNSPECIFIED. ) 
 CURVE ( )  GEOMETRIC_REPRESENTATION_ITEM ( )  RATIONAL_B_SPLINE_CURVE ( ( 0.9999999999999988898, 0.9510565162951546414, 1.000000000000000000, 0.9510565162951535312, 1.000000000000000000, 0.9510565162951535312, 1.000000000000000000, 0.9510565162951535312, 1.000000000000000000, 0.9510565162951521989, 1.000000000000001332 ) ) 
 REPRESENTATION_ITEM ( '' )  );
#69462=VECTOR ( 'NONE', #84230, 1000.000000000000114 ) ;
#69525=DIRECTION ( 'NONE',  ( 1.000000000000000000, -0.000000000000000000, -0.000000000000000000 ) ) ;
#69603=CIRCLE ( 'NONE', #198797, 2.649999999999992806 ) ;
#69607=CYLINDRICAL_SURFACE ( 'NONE', #37171, 37.99626262588765968 ) ;
#69628=CARTESIAN_POINT ( 'NONE',  ( 8.571926809382603096, -26.38167802310801235, 147.9750000027311785 ) ) ;
#69759=EDGE_CURVE ( 'NONE', #122026, #45563, #70190, .T. ) ;
#69794=AXIS2_PLACEMENT_3D ( 'NONE', #127896, #147080, #39887 ) ;
#69823=CARTESIAN_POINT ( 'NONE',  ( 30.73962218707677962, -22.33364281372841376, -5.202157773949823927 ) ) ;
#69880=CARTESIAN_POINT ( 'NONE',  ( -30.73962218707678318, -22.33364281372842441, -1.802157773949823127 ) ) ;
#69897=VECTOR ( 'NONE', #48771, 1000.000000000000114 ) ;
#69917=CARTESIAN_POINT ( 'NONE',  ( -32.22964258392465098, -4.577260022299249442, 89.03854312871814614 ) ) ;
#69921=CARTESIAN_POINT ( 'NONE',  ( -8.571926809382608425, 26.38167802310805854, 146.9750000027311785 ) ) ;
#69959=ORIENTED_EDGE ( 'NONE', *, *, #7934, .T. ) ;
#69996=CARTESIAN_POINT ( 'NONE',  ( 8.571926809382597767, 26.38167802310806209, 148.2750000027311899 ) ) ;
#70072=CARTESIAN_POINT ( 'NONE',  ( 23.48529157249599919, 32.32473071737754111, -6.449999994537626513 ) ) ;
#70120=CARTESIAN_POINT ( 'NONE',  ( 37.43947335741457039, 2.756686112915584630, 40.22705064412460985 ) ) ;
#70190=CIRCLE ( 'NONE', #31498, 0.2000000000000057288 ) ;
#70278=CARTESIAN_POINT ( 'NONE',  ( 38.00000000000000711, -12.34694845685040754, -3.100000000000000533 ) ) ;
#70384=ORIENTED_EDGE ( 'NONE', *, *, #22791, .T. ) ;
#70388=CARTESIAN_POINT ( 'NONE',  ( -3.573655867282028392E-15, 2.428612866367529932E-14, 150.0000000000000000 ) ) ;
#70396=CARTESIAN_POINT ( 'NONE',  ( -5.429308488886486681E-15, 30.30510711980690175, 141.5000000000000000 ) ) ;
#70449=CIRCLE ( 'NONE', #8977, 5.500000000001017852 ) ;
#70510=CARTESIAN_POINT ( 'NONE',  ( 22.44159573604009239, 16.30477369853692693, 140.0750000027311728 ) ) ;
#70603=CARTESIAN_POINT ( 'NONE',  ( -0.3641133308643078048, 37.60169961596129440, -7.999999999999994671 ) ) ;
#70606=DIRECTION ( 'NONE',  ( 1.000000000000000000, 0.000000000000000000, 0.000000000000000000 ) ) ;
#70616=EDGE_CURVE ( 'NONE', #184655, #171099, #1348, .T. ) ;
#70635=CARTESIAN_POINT ( 'NONE',  ( 36.91746824999999177, 2.880721459617395097E-14, -9.624999997268814056 ) ) ;
#70658=CARTESIAN_POINT ( 'NONE',  ( -34.54575687042841281, 4.960469055748716549, 50.63070180855214630 ) ) ;
#70870=VERTEX_POINT ( 'NONE', #63028 ) ;
#70884=CARTESIAN_POINT ( 'NONE',  ( -34.51794252349512249, -0.7246179257117795203, 89.53606970770105988 ) ) ;
#70886=CARTESIAN_POINT ( 'NONE',  ( -34.94848686537405769, -14.38147731881034375, -7.999999999999994671 ) ) ;
#70919=CARTESIAN_POINT ( 'NONE',  ( -32.53128430053963172, -2.419343514923748550, 87.89668391837240335 ) ) ;
#70923=CARTESIAN_POINT ( 'NONE',  ( 27.73933785331498214, 9.013057229001095294, 146.4750000027311501 ) ) ;
#70998=CARTESIAN_POINT ( 'NONE',  ( 17.14385361876520264, -23.59649016807270883, 147.5750000027311728 ) ) ;
#71047=EDGE_CURVE ( 'NONE', #126834, #155489, #35741, .T. ) ;
#71071=CARTESIAN_POINT ( 'NONE',  ( 11.74264578624800315, -36.14014761921581709, -9.149999994537626691 ) ) ;
#71081=DIRECTION ( 'NONE',  ( 0.000000000000000000, 0.000000000000000000, -1.000000000000000000 ) ) ;
#71107=CARTESIAN_POINT ( 'NONE',  ( 31.37700036491431632, 7.446261808816053041, 93.97872476790939800 ) ) ;
#71114=CARTESIAN_POINT ( 'NONE',  ( 31.76083434626055535, -6.487688756757409969, 91.22915654580297939 ) ) ;
#71121=CARTESIAN_POINT ( 'NONE',  ( 36.95577132204471837, 5.312067825339672922, 43.56319566887929540 ) ) ;
#71124=CARTESIAN_POINT ( 'NONE',  ( -34.36934878537049798, -7.254149193659903183, 46.92043707032850364 ) ) ;
#71153=LINE ( 'NONE', #27667, #47391 ) ;
#71237=CARTESIAN_POINT ( 'NONE',  ( -31.72709406046302760, 0.4964181571218586053, 102.5000000000000284 ) ) ;
#71263=DIRECTION ( 'NONE',  ( -6.982962677686266711E-15, 0.000000000000000000, 1.000000000000000000 ) ) ;
#71278=CARTESIAN_POINT ( 'NONE',  ( 3.766062262543149401E-15, -39.95556452105413570, -3.499999999999999556 ) ) ;
#71340=EDGE_LOOP ( 'NONE', ( #74505, #92312, #182159, #176265 ) ) ;
#71396=CARTESIAN_POINT ( 'NONE',  ( 28.82186960331498327, 2.781578969918950771E-14, 145.0000000000000000 ) ) ;
#71411=ORIENTED_EDGE ( 'NONE', *, *, #95173, .T. ) ;
#71503=VERTEX_POINT ( 'NONE', #16140 ) ;
#71506=DIRECTION ( 'NONE',  ( 0.000000000000000000, 0.000000000000000000, 1.000000000000000000 ) ) ;
#71523=CARTESIAN_POINT ( 'NONE',  ( 37.43820758241026425, -2.754439498815792753, 40.23603015349058154 ) ) ;
#71627=CARTESIAN_POINT ( 'NONE',  ( 3.556970738554033499E-15, -38.81732327939057825, -10.12499999726881228 ) ) ;
#71633=FACE_OUTER_BOUND ( 'NONE', #44445, .T. ) ;
#71650=CARTESIAN_POINT ( 'NONE',  ( -34.38590767368159362, 6.751198732549906545, 48.30327006964593295 ) ) ;
#71683=ADVANCED_FACE ( 'NONE', ( #17134 ), #61627, .T. ) ;
#71788=( BOUNDED_SURFACE ( )  B_SPLINE_SURFACE ( 1, 2, ( 
 ( #184660, #153316, #170481, #107796, #169480, #17802, #187660, #31971, #32968, #14817, #183676, #95615, #45161, #106817, #168491, #29989, #94622, #93627, #15808, #76478, #16801, #172470, #79459, #141128, #2618, #125962, #124972, #199836, #47144, #171479, #92628, #616, #49131, #78451, #77469, #110789, #60310, #62286, #1616, #123954, #138155, #63292, #61303, #185652, #48139, #108802, #33957, #18797, #53091, #85427, #96598, #7581, #54106, #115780, #129912, #158287, #143103, #69267, #35932, #20762, #174463, #4582, #126938, #6582, #130933, #159266, #146097, #175453, #99597, #51111, #23777, #84420, #177469, #128924, #173473, #3600, #19776, #36924, #81417, #66275, #38938, #144106, #5586, #98586, #68261, #100595, #67266, #97578, #145099, #82417, #192624, #190625, #162277, #114769, #65279, #188646, #50125, #52100, #37936, #111785, #191612 ),
 ( #160280, #112770, #34946, #21771, #127934, #189636, #176463, #113757, #83422, #161277, #22772, #28772, #39930, #151118, #197614, #59079, #73290, #132943, #42939, #167273, #194631, #88427, #164299, #56101, #26785, #181461, #118790, #195643, #147118, #9613, #134960, #70278, #8605, #165292, #196638, #71278, #89429, #120746, #58107, #102613, #180479, #119777, #87438, #41950, #133952, #27787, #117782, #86436, #131946, #179476, #150121, #103616, #25792, #43925, #40941, #149123, #104603, #12610, #178463, #10614, #101599, #163287, #193630, #11622, #24788, #166291, #182445, #74274, #135944, #105587, #55102, #116772, #148122, #72275, #57116, #154074, #187420, #78208, #153070, #62047, #140881, #124725, #156055, #152095, #185409, #172224, #44917, #29746, #94375, #122731, #107555, #61059, #91381, #13579, #93380, #17552, #45902, #32723, #123712, #186423, #137910 ) ),
 .UNSPECIFIED., .F., .F., .T. ) 
 B_SPLINE_SURFACE_WITH_KNOTS ( ( 2, 2 ),
 ( 3, 2, 2, 2, 2, 2, 2, 2, 2, 2, 2, 2, 2, 2, 2, 2, 2, 2, 2, 2, 2, 2, 2, 2, 2, 2, 2, 2, 2, 2, 2, 2, 2, 2, 2, 2, 2, 2, 2, 2, 2, 2, 2, 2, 2, 2, 2, 2, 2, 2, 3 ),
 ( 0.000000000000000000, 1.000000000000000000 ),
 ( 0.000000000000000000, 0.02000000000000000042, 0.04000000000000000083, 0.05999999999999999778, 0.08000000000000000167, 0.1000000000000000056, 0.1199999999999999956, 0.1400000000000000133, 0.1600000000000000033, 0.1799999999999999933, 0.2000000000000000111, 0.2200000000000000011, 0.2399999999999999911, 0.2600000000000000089, 0.2800000000000000266, 0.2999999999999999889, 0.3200000000000000067, 0.3400000000000000244, 0.3599999999999999867, 0.3800000000000000044, 0.4000000000000000222, 0.4199999999999999845, 0.4400000000000000022, 0.4600000000000000200, 0.4799999999999999822, 0.5000000000000000000, 0.5200000000000000178, 0.5400000000000000355, 0.5600000000000000533, 0.5799999999999999600, 0.5999999999999999778, 0.6199999999999999956, 0.6400000000000000133, 0.6600000000000000311, 0.6800000000000000488, 0.6999999999999999556, 0.7199999999999999734, 0.7399999999999999911, 0.7600000000000000089, 0.7800000000000000266, 0.8000000000000000444, 0.8199999999999999512, 0.8399999999999999689, 0.8599999999999999867, 0.8800000000000000044, 0.9000000000000000222, 0.9200000000000000400, 0.9399999999999999467, 0.9599999999999999645, 0.9799999999999999822, 1.000000000000000000 ),
 .UNSPECIFIED. ) 
 GEOMETRIC_REPRESENTATION_ITEM ( )  RATIONAL_B_SPLINE_SURFACE ( (
 ( 1.000000000000000000, 0.9510565162951535312, 1.000000000000000000, 0.9510565162951535312, 1.000000000000000000, 0.9510565162951535312, 1.000000000000000000, 0.9510565162951535312, 1.000000000000000000, 0.9510565162951535312, 1.000000000000000000, 0.9510565162951535312, 1.000000000000000000, 0.9510565162951535312, 1.000000000000000000, 0.9510565162951535312, 1.000000000000000000, 0.9510565162951535312, 1.000000000000000000, 0.9510565162951535312, 1.000000000000000000, 0.9510565162951535312, 1.000000000000000000, 0.9510565162951535312, 1.000000000000000000, 0.9510565162951535312, 1.000000000000000000, 0.9510565162951535312, 1.000000000000000000, 0.9510565162951535312, 1.000000000000000000, 0.9510565162951535312, 1.000000000000000000, 0.9510565162951535312, 1.000000000000000000, 0.9510565162951535312, 1.000000000000000000, 0.9510565162951535312, 1.000000000000000000, 0.9510565162951535312, 1.000000000000000000, 0.9510565162951535312, 1.000000000000000000, 0.9510565162951535312, 1.000000000000000000, 0.9510565162951535312, 1.000000000000000000, 0.9510565162951535312, 1.000000000000000000, 0.9510565162951535312, 1.000000000000000000, 0.9510565162951535312, 1.000000000000000000, 0.9510565162951535312, 1.000000000000000000, 0.9510565162951535312, 1.000000000000000000, 0.9510565162951535312, 1.000000000000000000, 0.9510565162951535312, 1.000000000000000000, 0.9510565162951535312, 1.000000000000000000, 0.9510565162951535312, 1.000000000000000000, 0.9510565162951535312, 1.000000000000000000, 0.9510565162951535312, 1.000000000000000000, 0.9510565162951535312, 1.000000000000000000, 0.9510565162951535312, 1.000000000000000000, 0.9510565162951535312, 1.000000000000000000, 0.9510565162951535312, 1.000000000000000000, 0.9510565162951535312, 1.000000000000000000, 0.9510565162951535312, 1.000000000000000000, 0.9510565162951535312, 1.000000000000000000, 0.9510565162951535312, 1.000000000000000000, 0.9510565162951535312, 1.000000000000000000, 0.9510565162951535312, 1.000000000000000000, 0.9510565162951535312, 1.000000000000000000, 0.9510565162951535312, 1.000000000000000000, 0.9510565162951535312, 1.000000000000000000, 0.9510565162951535312, 1.000000000000000000, 0.9510565162951535312, 1.000000000000000000, 0.9510565162951535312, 1.000000000000000000),
 ( 1.000000000000000000, 0.9510565162951535312, 1.000000000000000000, 0.9510565162951535312, 1.000000000000000000, 0.9510565162951535312, 1.000000000000000000, 0.9510565162951535312, 1.000000000000000000, 0.9510565162951535312, 1.000000000000000000, 0.9510565162951535312, 1.000000000000000000, 0.9510565162951535312, 1.000000000000000000, 0.9510565162951535312, 1.000000000000000000, 0.9510565162951535312, 1.000000000000000000, 0.9510565162951535312, 1.000000000000000000, 0.9510565162951535312, 1.000000000000000000, 0.9510565162951535312, 1.000000000000000000, 0.9510565162951535312, 1.000000000000000000, 0.9510565162951535312, 1.000000000000000000, 0.9510565162951535312, 1.000000000000000000, 0.9510565162951535312, 1.000000000000000000, 0.9510565162951535312, 1.000000000000000000, 0.9510565162951535312, 1.000000000000000000, 0.9510565162951535312, 1.000000000000000000, 0.9510565162951535312, 1.000000000000000000, 0.9510565162951535312, 1.000000000000000000, 0.9510565162951535312, 1.000000000000000000, 0.9510565162951535312, 1.000000000000000000, 0.9510565162951535312, 1.000000000000000000, 0.9510565162951535312, 1.000000000000000000, 0.9510565162951535312, 1.000000000000000000, 0.9510565162951535312, 1.000000000000000000, 0.9510565162951535312, 1.000000000000000000, 0.9510565162951535312, 1.000000000000000000, 0.9510565162951535312, 1.000000000000000000, 0.9510565162951535312, 1.000000000000000000, 0.9510565162951535312, 1.000000000000000000, 0.9510565162951535312, 1.000000000000000000, 0.9510565162951535312, 1.000000000000000000, 0.9510565162951535312, 1.000000000000000000, 0.9510565162951535312, 1.000000000000000000, 0.9510565162951535312, 1.000000000000000000, 0.9510565162951535312, 1.000000000000000000, 0.9510565162951535312, 1.000000000000000000, 0.9510565162951535312, 1.000000000000000000, 0.9510565162951535312, 1.000000000000000000, 0.9510565162951535312, 1.000000000000000000, 0.9510565162951535312, 1.000000000000000000, 0.9510565162951535312, 1.000000000000000000, 0.9510565162951535312, 1.000000000000000000, 0.9510565162951535312, 1.000000000000000000, 0.9510565162951535312, 1.000000000000000000, 0.9510565162951535312, 1.000000000000000000, 0.9510565162951535312, 1.000000000000000000, 0.9510565162951535312, 1.000000000000000000) ) ) 
 REPRESENTATION_ITEM ( '' )  SURFACE ( )  );
#71878=DIRECTION ( 'NONE',  ( 0.000000000000000000, 0.000000000000000000, 1.000000000000000000 ) ) ;
#71911=CARTESIAN_POINT ( 'NONE',  ( -31.48242569098778176, -7.251655820954945320, 93.02470426148724414 ) ) ;
#71915=CARTESIAN_POINT ( 'NONE',  ( -22.44159573604009950, -16.30477369853688430, 141.5750000027311728 ) ) ;
#72031=CARTESIAN_POINT ( 'NONE',  ( 8.906447517083050158, 27.41122689804195645, 147.4000000000000057 ) ) ;
#72062=CARTESIAN_POINT ( 'NONE',  ( -38.00000000000000711, 2.428612866367529932E-14, -7.749999994537626336 ) ) ;
#72073=ORIENTED_EDGE ( 'NONE', *, *, #94442, .T. ) ;
#72103=CARTESIAN_POINT ( 'NONE',  ( 31.68361083058364613, 1.948458647159017509, 102.2466786067742959 ) ) ;
#72120=CARTESIAN_POINT ( 'NONE',  ( -34.77074502975527537, -6.826893893699448768, 41.88499232265944983 ) ) ;
#72143=CARTESIAN_POINT ( 'NONE',  ( 32.00000000000000000, -1.163414459189985801E-14, 95.00000000000000000 ) ) ;
#72160=CARTESIAN_POINT ( 'NONE',  ( 8.571926809382603096, -26.38167802310801235, 145.4750000027311785 ) ) ;
#72164=ORIENTED_EDGE ( 'NONE', *, *, #169778, .T. ) ;
#72275=CARTESIAN_POINT ( 'NONE',  ( 23.48529157249600630, -32.32473071737749137, -7.299999999999998934 ) ) ;
#72314=EDGE_CURVE ( 'NONE', #103711, #21447, #68243, .T. ) ;
#72322=ORIENTED_EDGE ( 'NONE', *, *, #178834, .F. ) ;
#72341=EDGE_CURVE ( 'NONE', #153137, #111465, #181775, .T. ) ;
#72396=CARTESIAN_POINT ( 'NONE',  ( 28.82186960331498327, 9.364793116373570925, 141.0999999999999943 ) ) ;
#72398=CARTESIAN_POINT ( 'NONE',  ( -28.82186960331499392, -9.364793116373526516, 138.3500000054623911 ) ) ;
#72433=ADVANCED_FACE ( 'NONE', ( #149437, #180794 ), #72606, .F. ) ;
#72475=AXIS2_PLACEMENT_3D ( 'NONE', #152494, #199007, #60474 ) ;
#72606=PLANE ( 'NONE',  #167188 ) ;
#72609=CARTESIAN_POINT ( 'NONE',  ( 28.82186960331480208, -9.364793116373776982, 141.1500000054623740 ) ) ;
#72636=CARTESIAN_POINT ( 'NONE',  ( -36.91746825000001309, -11.99521256947794789, -10.52499999726881441 ) ) ;
#72705=EDGE_CURVE ( 'NONE', #106856, #142504, #151437, .T. ) ;
#72889=CARTESIAN_POINT ( 'NONE',  ( 29.86685920354754487, 21.69954338932564752, -1.924999997268813212 ) ) ;
#72896=CARTESIAN_POINT ( 'NONE',  ( -18.30394412277474103, -32.66729986584498135, -8.000000000000000000 ) ) ;
#72906=DIRECTION ( 'NONE',  ( -1.000000000000000000, 0.000000000000000000, 0.000000000000000000 ) ) ;
#72908=CARTESIAN_POINT ( 'NONE',  ( 11.40812507854755253, -35.11059874428192273, -2.524999997268813523 ) ) ;
#72915=EDGE_CURVE ( 'NONE', #150593, #136632, #92231, .T. ) ;
#72930=CARTESIAN_POINT ( 'NONE',  ( -32.63052366545711180, -0.9798963808688879729, 87.54781425814060469 ) ) ;
#72934=CARTESIAN_POINT ( 'NONE',  ( -27.73933785331498925, 2.428612866367529932E-14, 139.3750000027311842 ) ) ;
#72946=VERTEX_POINT ( 'NONE', #90729 ) ;
#72967=LINE ( 'NONE', #183117, #104758 ) ;
#73026=CARTESIAN_POINT ( 'NONE',  ( -3.573655867282028392E-15, 2.428612866367529932E-14, 139.9999999999999716 ) ) ;
#73079=CARTESIAN_POINT ( 'NONE',  ( 30.74264578624800137, -22.33583958711395212, -8.949999994537627401 ) ) ;
#73129=CARTESIAN_POINT ( 'NONE',  ( 31.65994483839895679, -2.419126180341553578, 102.1034561864645980 ) ) ;
#73135=CARTESIAN_POINT ( 'NONE',  ( 36.77035430826401097, 5.154579508995670523, 46.92692430510571455 ) ) ;
#73138=CARTESIAN_POINT ( 'NONE',  ( -34.67490716095264958, -3.335491994402104865, 51.73554620185603170 ) ) ;
#73162=CARTESIAN_POINT ( 'NONE',  ( 30.00000000000000711, -1.163414459189985801E-14, 95.00000000000000000 ) ) ;
#73167=CARTESIAN_POINT ( 'NONE',  ( -37.01127658466555914, 5.144934411046666156, 43.04759647146321555 ) ) ;
#73179=CARTESIAN_POINT ( 'NONE',  ( 17.14385361876520264, 23.59649016807275856, 144.1750000027311671 ) ) ;
#73219=DIRECTION ( 'NONE',  ( -0.8660254037844410391, 0.000000000000000000, 0.4999999999999958367 ) ) ;
#73290=CARTESIAN_POINT ( 'NONE',  ( -11.74264578624799782, -36.14014761921581709, -1.599999999999999867 ) ) ;
#73347=EDGE_CURVE ( 'NONE', #191417, #89861, #162075, .T. ) ;
#73351=ORIENTED_EDGE ( 'NONE', *, *, #142462, .F. ) ;
#73380=CARTESIAN_POINT ( 'NONE',  ( -37.45873412500000654, 2.428612866367529932E-14, -0.3124999986344065839 ) ) ;
#73392=AXIS2_PLACEMENT_3D ( 'NONE', #132346, #84818, #39334 ) ;
#73408=DIRECTION ( 'NONE',  ( 1.000000000000000000, 0.000000000000000000, 0.000000000000000000 ) ) ;
#73612=CARTESIAN_POINT ( 'NONE',  ( -28.82186960331499037, 2.428612866367529932E-14, 140.2500000054623683 ) ) ;
#73624=ORIENTED_EDGE ( 'NONE', *, *, #155268, .T. ) ;
#73638=CARTESIAN_POINT ( 'NONE',  ( 1.784210473542230573E-15, -29.16686587814331588, 141.8750000027311842 ) ) ;
#73645=DIRECTION ( 'NONE',  ( 1.000000000000000000, -0.000000000000000000, -0.000000000000000000 ) ) ;
#73707=ORIENTED_EDGE ( 'NONE', *, *, #4758, .F. ) ;
#73771=CARTESIAN_POINT ( 'NONE',  ( -6.019987952026119621E-15, 39.95163481335720235, -4.247842220587803475 ) ) ;
#73882=CARTESIAN_POINT ( 'NONE',  ( -29.86685920354755552, 21.69954338932564397, -5.324999997268814234 ) ) ;
#73888=CARTESIAN_POINT ( 'NONE',  ( -32.52061478538139028, -19.14287791848993336, -8.000000000000003553 ) ) ;
#73900=CARTESIAN_POINT ( 'NONE',  ( 11.40812507854754365, 35.11059874428196537, -3.724999997268813701 ) ) ;
#73992=DIRECTION ( 'NONE',  ( 0.000000000000000000, 0.000000000000000000, -1.000000000000000000 ) ) ;
#74000=DIRECTION ( 'NONE',  ( -8.551662891793917213E-31, 1.000000000000000000, 1.224646799147353207E-16 ) ) ;
#74009=VECTOR ( 'NONE', #2215, 1000.000000000000000 ) ;
#74034=DIRECTION ( 'NONE',  ( 0.000000000000000000, 0.000000000000000000, -1.000000000000000000 ) ) ;
#74069=CARTESIAN_POINT ( 'NONE',  ( -23.48529157249599919, -32.32473071737750558, -9.449999994537623849 ) ) ;
#74121=CARTESIAN_POINT ( 'NONE',  ( 36.77100073307799022, 4.779104515855422619, 47.74589100149061949 ) ) ;
#74147=DIRECTION ( 'NONE',  ( 0.000000000000000000, 0.000000000000000000, -1.000000000000000000 ) ) ;
#74152=AXIS2_PLACEMENT_3D ( 'NONE', #55824, #82132, #7304 ) ;
#74153=CARTESIAN_POINT ( 'NONE',  ( -37.36578165719733846, 3.357000025855910064, 40.62839678089418527 ) ) ;
#74159=CARTESIAN_POINT ( 'NONE',  ( 8.571926809382603096, -26.38167802310801235, 145.4750000027311785 ) ) ;
#74164=CARTESIAN_POINT ( 'NONE',  ( 17.14385361876520264, -23.59649016807271238, 147.5750000027311444 ) ) ;
#74233=CARTESIAN_POINT ( 'NONE',  ( 23.31738231874054890, -16.94106989632523508, 146.7999999999999829 ) ) ;
#74235=LINE ( 'NONE', #147083, #27273 ) ;
#74274=CARTESIAN_POINT ( 'NONE',  ( 23.48529157249599919, 32.32473071737754111, -6.700000000000001066 ) ) ;
#74326=CARTESIAN_POINT ( 'NONE',  ( 34.48171762721879929, 5.660481407866305936, 49.94458042978408940 ) ) ;
#74505=ORIENTED_EDGE ( 'NONE', *, *, #21468, .F. ) ;
#74588=CARTESIAN_POINT ( 'NONE',  ( 10.18315950979500251, 36.03432976468644000, -8.000000000000003553 ) ) ;
#74591=CARTESIAN_POINT ( 'NONE',  ( 17.81289503416611453, -24.51734667627695785, 140.9500000054623570 ) ) ;
#74620=CARTESIAN_POINT ( 'NONE',  ( 8.571926809382603096, -26.38167802310801235, 145.9750000027311785 ) ) ;
#74645=CARTESIAN_POINT ( 'NONE',  ( -28.82186960331499392, 9.364793116373565596, 148.1500000054624024 ) ) ;
#74667=CYLINDRICAL_SURFACE ( 'NONE', #17203, 7.500000000000000000 ) ;
#74756=B_SPLINE_CURVE_WITH_KNOTS ( 'NONE', 3,
 ( #190471, #192468, #21612, #23621, #191456, #85268, #177316, #66116, #70120, #127781, #100444, #131791, #112618, #54948, #174310, #35779, #195482, #71121, #39772, #179320, #27635, #163127, #194474, #104450, #26627, #132787, #73135, #118631, #74121, #121586, #42787, #166133, #24630, #56957, #55946, #101436, #40784, #89276, #59918, #151941, #103457, #88270 ),
 .UNSPECIFIED., .F., .F.,
 ( 4, 2, 2, 2, 2, 2, 2, 2, 2, 2, 2, 2, 2, 2, 2, 2, 2, 2, 2, 2, 4 ),
 ( 0.004226304204691699526, 0.005303825792898752590, 0.005842586587002279556, 0.006381347381105806522, 0.007458868969312861322, 0.008536390557519916988, 0.009613912145726972655, 0.01069143373393402832, 0.01123019452803756396, 0.01176895532214110307, 0.01284647691034817608, 0.01392399849855525083, 0.01446275929265878647, 0.01500152008676232558, 0.01607904167496940206, 0.01715656326317647334, 0.01823408485138354809, 0.01877284564548709067, 0.01931160643959063325, 0.02038912802779771494, 0.02146664961600480703 ),
 .UNSPECIFIED. ) ;
#74861=CARTESIAN_POINT ( 'NONE',  ( 11.40812507854754365, 35.11059874428196537, -7.724999997268813701 ) ) ;
#74867=CARTESIAN_POINT ( 'NONE',  ( 34.40575365382723305, 2.434396366613707396, 90.06480789948632548 ) ) ;
#74900=CARTESIAN_POINT ( 'NONE',  ( -31.56677620984798338, -3.765895691706333093, 101.5045925518948593 ) ) ;
#74905=DIRECTION ( 'NONE',  ( 0.8660254037844410391, 0.000000000000000000, 0.4999999999999958367 ) ) ;
#74971=EDGE_LOOP ( 'NONE', ( #1033, #56198 ) ) ;
#75044=CARTESIAN_POINT ( 'NONE',  ( 38.00000000000000000, 12.34694845685046616, -10.64999999453762491 ) ) ;
#75062=DIRECTION ( 'NONE',  ( 0.000000000000000000, 0.000000000000000000, 1.000000000000000000 ) ) ;
#75125=CARTESIAN_POINT ( 'NONE',  ( -36.77234560139673647, 5.215770478161305235, 46.75454185840153798 ) ) ;
#75131=CARTESIAN_POINT ( 'NONE',  ( 17.14385361876520264, 23.59649016807275856, 144.1750000027311671 ) ) ;
#75136=CARTESIAN_POINT ( 'NONE',  ( -17.14385361876520264, -23.59649016807271593, 145.1750000027311387 ) ) ;
#75181=FACE_OUTER_BOUND ( 'NONE', #169155, .T. ) ;
#75208=CARTESIAN_POINT ( 'NONE',  ( -27.73933785331498925, 2.428612866367529932E-14, 149.3750000027311842 ) ) ;
#75298=CARTESIAN_POINT ( 'NONE',  ( 34.36935609104189382, 7.254501760396902199, 46.91913033384989262 ) ) ;
#75534=DIRECTION ( 'NONE',  ( -0.06104853953485701173, -7.476289853398329258E-18, -0.9981347984218670311 ) ) ;
#75540=VECTOR ( 'NONE', #73408, 1000.000000000000000 ) ;
#75586=CARTESIAN_POINT ( 'NONE',  ( 31.99364916730973363, -1.163414459185697237E-14, 92.35000000000020748 ) ) ;
#75596=CARTESIAN_POINT ( 'NONE',  ( 1.784210473542230573E-15, -29.16686587814331588, 143.8750000027311557 ) ) ;
#75619=CARTESIAN_POINT ( 'NONE',  ( -35.69940131823277341, 0.4911691522781976293, 37.51200899188186355 ) ) ;
#75836=CARTESIAN_POINT ( 'NONE',  ( -11.40812507854754720, -35.11059874428192273, -8.724999997268813701 ) ) ;
#75837=CARTESIAN_POINT ( 'NONE',  ( -34.35276339089875108, 2.907959671212060559, 90.32815265678038941 ) ) ;
#75843=CARTESIAN_POINT ( 'NONE',  ( 34.52594549653174028, 0.3596637467104462083, 89.49999999999900524 ) ) ;
#75855=CARTESIAN_POINT ( 'NONE',  ( -5.950531402560715689E-15, 38.81732327939063509, -7.624999997268814056 ) ) ;
#75858=AXIS2_PLACEMENT_3D ( 'NONE', #19875, #161380, #128035 ) ;
#75917=CARTESIAN_POINT ( 'NONE',  ( 23.31738231874054534, 16.94106989632529192, 139.4500000054623570 ) ) ;
#75920=CARTESIAN_POINT ( 'NONE',  ( -28.82186960331480208, 9.364793116373830273, 141.9000000000000057 ) ) ;
#75921=ORIENTED_EDGE ( 'NONE', *, *, #68080, .F. ) ;
#75943=CARTESIAN_POINT ( 'NONE',  ( -31.37858599332832910, 5.662547894918618319, 99.94225302722342974 ) ) ;
#75959=CARTESIAN_POINT ( 'NONE',  ( 31.99999999999936051, 1.011767027235951731E-12, 92.30000000000021032 ) ) ;
#76028=CARTESIAN_POINT ( 'NONE',  ( -22.81625015709509441, -31.40387420917324590, -6.824999997268814234 ) ) ;
#76076=CARTESIAN_POINT ( 'NONE',  ( -28.82186960331483760, 9.364793116373787640, 143.9000000000000057 ) ) ;
#76080=EDGE_CURVE ( 'NONE', #193619, #120101, #90078, .T. ) ;
#76110=CARTESIAN_POINT ( 'NONE',  ( -32.00000000000000711, -5.180255960393304182E-15, 47.70000000000000284 ) ) ;
#76116=CARTESIAN_POINT ( 'NONE',  ( 1.784210473542230573E-15, -29.16686587814331588, 145.3750000027311842 ) ) ;
#76121=CARTESIAN_POINT ( 'NONE',  ( -5.359611314223446995E-15, 29.16686587814335496, 146.3750000027311842 ) ) ;
#76167=CYLINDRICAL_SURFACE ( 'NONE', #5201, 28.82186960331498682 ) ;
#76211=CARTESIAN_POINT ( 'NONE',  ( 28.82186960331498327, 2.781578969918950771E-14, 145.2500000054623683 ) ) ;
#76215=FACE_OUTER_BOUND ( 'NONE', #166207, .T. ) ;
#76397=ORIENTED_EDGE ( 'NONE', *, *, #178712, .T. ) ;
#76478=CARTESIAN_POINT ( 'NONE',  ( -36.91746825000001309, -11.99521256947794789, -2.524999997268813523 ) ) ;
#76530=CIRCLE ( 'NONE', #31358, 2.700000000000001066 ) ;
#76594=CARTESIAN_POINT ( 'NONE',  ( 1.784210473542230573E-15, -29.16686587814331588, 145.8750000027311273 ) ) ;
#76617=CARTESIAN_POINT ( 'NONE',  ( -28.82186960331499392, 9.364793116373565596, 144.1500000054623740 ) ) ;
#76637=DIRECTION ( 'NONE',  ( 0.000000000000000000, 0.000000000000000000, -1.000000000000000000 ) ) ;
#76706=CARTESIAN_POINT ( 'NONE',  ( -27.73933785331498925, -9.013057229001049109, 140.9750000027311785 ) ) ;
#76719=CARTESIAN_POINT ( 'NONE',  ( 28.82186960331498327, 2.428612866367529932E-14, 139.9999999999999716 ) ) ;
#76737=B_SPLINE_CURVE_WITH_KNOTS ( 'NONE', 3,
 ( #145709, #34556, #96215, #7191, #130534, #53713, #65876, #157904, #127550, #189251, #50728, #112386, #12225, #134564, #9219, #56722, #119391, #179078, #148730, #42549, #26394, #72896, #54707, #25403, #117381, #88033, #149721, #197230, #90028, #182054, #133548, #58691, #73888, #102218, #118393, #10218, #70886, #181074, #196252, #116379, #40549, #43537, #163907, #57721, #55709, #11221 ),
 .UNSPECIFIED., .F., .F.,
 ( 4, 2, 2, 2, 2, 2, 2, 2, 2, 2, 2, 2, 2, 2, 2, 2, 2, 2, 2, 2, 2, 2, 4 ),
 ( 0.000000000000000000, 0.004592541348721043692, 0.006888812023081562069, 0.009185082697442082181, 0.01148135337180260229, 0.01377762404616312067, 0.01837016539488416089, 0.02296270674360520112, 0.02755524809232623787, 0.02985151876668676665, 0.03214778944104729197, 0.03674033078976832872, 0.04133287213848937242, 0.04592541348721041611, 0.04822168416157093795, 0.05051795483593145980, 0.05511049618465248268, 0.05740676685901301146, 0.05970303753337353331, 0.06429557888209455618, 0.06659184955645508497, 0.06888812023081561375, 0.07348066157953664357 ),
 .UNSPECIFIED. ) ;
#76743=CARTESIAN_POINT ( 'NONE',  ( -3.573655867282028392E-15, 2.428612866367529932E-14, 139.9999999999999716 ) ) ;
#76761=CARTESIAN_POINT ( 'NONE',  ( -28.82186960331499392, 9.364793116373565596, 149.9000000000000057 ) ) ;
#76831=CARTESIAN_POINT ( 'NONE',  ( 11.40812507854755253, -35.11059874428192273, -8.524999997268814411 ) ) ;
#76912=ORIENTED_EDGE ( 'NONE', *, *, #59414, .T. ) ;
#76935=CARTESIAN_POINT ( 'NONE',  ( -31.60134953801818014, 3.338644055332177896, 101.7340227041930234 ) ) ;
#77019=CARTESIAN_POINT ( 'NONE',  ( -36.91746825000000598, 2.428612866367529932E-14, -9.124999997268814056 ) ) ;
#77033=ORIENTED_EDGE ( 'NONE', *, *, #155268, .F. ) ;
#77112=CARTESIAN_POINT ( 'NONE',  ( -17.14385361876520619, 23.59649016807275856, 146.5750000027311444 ) ) ;
#77271=VERTEX_POINT ( 'NONE', #11980 ) ;
#77276=CARTESIAN_POINT ( 'NONE',  ( 34.98624150382327969, 6.090157606732328865, 40.61607269374898266 ) ) ;
#77296=ADVANCED_FACE ( 'NONE', ( #102966 ), #86473, .T. ) ;
#77338=EDGE_CURVE ( 'NONE', #34628, #54169, #141446, .T. ) ;
#77426=ADVANCED_FACE ( 'NONE', ( #71633 ), #149473, .T. ) ;
#77432=CARTESIAN_POINT ( 'NONE',  ( 31.99999999999934275, 1.011436372600181938E-12, 95.00000000000021316 ) ) ;
#77464=ORIENTED_EDGE ( 'NONE', *, *, #18367, .F. ) ;
#77469=CARTESIAN_POINT ( 'NONE',  ( 11.40812507854755253, -35.11059874428192273, -4.024999997268814411 ) ) ;
#77540=FACE_BOUND ( 'NONE', #91970, .T. ) ;
#77557=CARTESIAN_POINT ( 'NONE',  ( -36.81601778013477855, -3.637449627666676122, 49.14141020753753963 ) ) ;
#77560=DIRECTION ( 'NONE',  ( -1.000000000000000000, 0.000000000000000000, 0.000000000000000000 ) ) ;
#77588=CARTESIAN_POINT ( 'NONE',  ( -17.14385361876520264, -23.59649016807271593, 145.6750000027311671 ) ) ;
#77612=CARTESIAN_POINT ( 'NONE',  ( -35.52763170759350686, 3.100152895725881930, 38.16632899394345912 ) ) ;
#77615=AXIS2_PLACEMENT_3D ( 'NONE', #41934, #102598, #195627 ) ;
#77633=DIRECTION ( 'NONE',  ( 0.000000000000000000, 0.000000000000000000, -1.000000000000000000 ) ) ;
#77634=CARTESIAN_POINT ( 'NONE',  ( 23.31738231874054890, -16.94106989632523508, 142.7999999999999829 ) ) ;
#77702=CARTESIAN_POINT ( 'NONE',  ( 22.44159573604009594, -16.30477369853687364, 143.6750000027311671 ) ) ;
#77822=CARTESIAN_POINT ( 'NONE',  ( 11.40812507854754365, 35.11059874428196537, -1.224999997268813479 ) ) ;
#77829=CARTESIAN_POINT ( 'NONE',  ( 33.86350577294170705, 5.311679113341320146, 93.56182321589975004 ) ) ;
#77841=CARTESIAN_POINT ( 'NONE',  ( -36.91746825000000598, -11.99521256947794789, -5.024999997268813523 ) ) ;
#78008=CARTESIAN_POINT ( 'NONE',  ( -22.81625015709509441, -31.40387420917324590, -4.824999997268813345 ) ) ;
#78091=CARTESIAN_POINT ( 'NONE',  ( -36.85386064174076637, 2.754345082724620752, 49.76404540304364588 ) ) ;
#78096=CARTESIAN_POINT ( 'NONE',  ( 17.14385361876520264, -23.59649016807271238, 147.5750000027311444 ) ) ;
#78101=CARTESIAN_POINT ( 'NONE',  ( -27.73933785331498925, -9.013057229001049109, 138.9750000027311785 ) ) ;
#78137=ORIENTED_EDGE ( 'NONE', *, *, #185806, .T. ) ;
#78208=CARTESIAN_POINT ( 'NONE',  ( -23.48529157249599919, -32.32473071737750558, -7.699999999999999289 ) ) ;
#78258=CARTESIAN_POINT ( 'NONE',  ( 34.46971384048857345, 7.497988128173094680, 44.47943501004273514 ) ) ;
#78415=CARTESIAN_POINT ( 'NONE',  ( 33.74160284725414982, -3.639722220971261635, 99.13931652913686321 ) ) ;
#78451=CARTESIAN_POINT ( 'NONE',  ( 22.81625015709510151, -31.40387420917324590, -3.924999997268811658 ) ) ;
#78541=CARTESIAN_POINT ( 'NONE',  ( -36.79334119018159299, -4.151185298968584014, 48.62628996558957084 ) ) ;
#78544=DIRECTION ( 'NONE',  ( 0.000000000000000000, 0.000000000000000000, -1.000000000000000000 ) ) ;
#78562=CIRCLE ( 'NONE', #46250, 28.82186960331498682 ) ;
#78573=CARTESIAN_POINT ( 'NONE',  ( -23.31738231874055600, 16.94106989632528837, 147.7999999999999829 ) ) ;
#78598=CARTESIAN_POINT ( 'NONE',  ( 1.993301997531345292E-15, -30.30510711980685912, 144.7500000054623399 ) ) ;
#78689=CARTESIAN_POINT ( 'NONE',  ( 27.73933785331498569, 2.768321779492822058E-14, 143.8750000027311842 ) ) ;
#78815=CARTESIAN_POINT ( 'NONE',  ( -29.86685920354755197, -21.69954338932560134, -8.924999997268812990 ) ) ;
#78816=CARTESIAN_POINT ( 'NONE',  ( -34.48736576873178450, 1.429538131128952561, 89.67663809442002787 ) ) ;
#78820=CARTESIAN_POINT ( 'NONE',  ( 34.42157296979474523, 2.272259278789490189, 89.98812102125175727 ) ) ;
#78895=VECTOR ( 'NONE', #54281, 1000.000000000000000 ) ;
#78930=CARTESIAN_POINT ( 'NONE',  ( -20.34036572606774484, 20.41983568886641365, 139.9999999999999716 ) ) ;
#78948=EDGE_CURVE ( 'NONE', #77271, #108481, #45400, .T. ) ;
#79005=CARTESIAN_POINT ( 'NONE',  ( 36.91746825000000598, -11.99521256947793546, -6.224999997268814589 ) ) ;
#79021=ORIENTED_EDGE ( 'NONE', *, *, #58712, .F. ) ;
#79032=EDGE_CURVE ( 'NONE', #1947, #50775, #70449, .T. ) ;
#79094=CARTESIAN_POINT ( 'NONE',  ( -22.44159573604010305, 16.30477369853692338, 142.6750000027311671 ) ) ;
#79099=CARTESIAN_POINT ( 'NONE',  ( -17.14385361876520264, -23.59649016807271593, 141.1750000027311671 ) ) ;
#79116=VECTOR ( 'NONE', #75062, 1000.000000000000000 ) ;
#79135=ORIENTED_EDGE ( 'NONE', *, *, #80827, .T. ) ;
#79191=EDGE_CURVE ( 'NONE', #90959, #72946, #154561, .T. ) ;
#79218=CARTESIAN_POINT ( 'NONE',  ( -28.82186960331499037, 2.428612866367529617E-14, 148.0000000000000000 ) ) ;
#79307=DIRECTION ( 'NONE',  ( -1.000000000000000000, 0.000000000000000000, 0.000000000000000000 ) ) ;
#79459=CARTESIAN_POINT ( 'NONE',  ( -29.86685920354755552, 21.69954338932564397, -2.824999997268813345 ) ) ;
#79533=CARTESIAN_POINT ( 'NONE',  ( -3.573655867282028392E-15, 2.428612866367529932E-14, 139.9999999999999716 ) ) ;
#79548=CARTESIAN_POINT ( 'NONE',  ( -36.77116682341763010, -5.223593267096957149, 46.75914592492878796 ) ) ;
#79578=CARTESIAN_POINT ( 'NONE',  ( -23.31738231874055245, -16.94106989632524574, 148.1999999999999886 ) ) ;
#79601=CARTESIAN_POINT ( 'NONE',  ( -27.73933785331498925, 2.428612866367529932E-14, 148.8750000027311842 ) ) ;
#79666=CARTESIAN_POINT ( 'NONE',  ( -23.48298174826590667, 32.32155151706776053, -2.047842220587803297 ) ) ;
#79694=CARTESIAN_POINT ( 'NONE',  ( -27.73933785331498925, 2.428612866367529932E-14, 144.8750000027311842 ) ) ;
#79806=ORIENTED_EDGE ( 'NONE', *, *, #186365, .F. ) ;
#79810=CARTESIAN_POINT ( 'NONE',  ( 28.82186960331498327, 2.781578969918950771E-14, 147.2500000054623683 ) ) ;
#79812=AXIS2_PLACEMENT_3D ( 'NONE', #184500, #157136, #199672 ) ;
#79820=CARTESIAN_POINT ( 'NONE',  ( -5.950531402560715689E-15, 38.81732327939063509, -7.124999997268814944 ) ) ;
#79823=CARTESIAN_POINT ( 'NONE',  ( -30.73962218707677962, -22.33364281372842441, -3.547842220587803297 ) ) ;
#79838=CARTESIAN_POINT ( 'NONE',  ( 29.86685920354754487, 21.69954338932564752, -5.924999997268813878 ) ) ;
#79873=CARTESIAN_POINT ( 'NONE',  ( 34.41611627805853857, -6.381310488372548662, 48.94841969467694298 ) ) ;
#79878=FACE_OUTER_BOUND ( 'NONE', #29669, .T. ) ;
#79968=EDGE_CURVE ( 'NONE', #136632, #2296, #51359, .T. ) ;
#80009=CARTESIAN_POINT ( 'NONE',  ( -36.91746825000001309, -11.99521256947794789, -5.024999997268813523 ) ) ;
#80063=CARTESIAN_POINT ( 'NONE',  ( -40.00000000000002842, 1.938754146708588393E-14, 0.000000000000000000 ) ) ;
#80093=CARTESIAN_POINT ( 'NONE',  ( -27.73933785331498925, -9.013057229001049109, 138.9750000027311785 ) ) ;
#80161=CARTESIAN_POINT ( 'NONE',  ( 22.44159573604009594, -16.30477369853687364, 144.1750000027311671 ) ) ;
#80250=ORIENTED_EDGE ( 'NONE', *, *, #105310, .T. ) ;
#80289=DIRECTION ( 'NONE',  ( 1.000000000000000000, -0.000000000000000000, -0.000000000000000000 ) ) ;
#80291=CARTESIAN_POINT ( 'NONE',  ( -3.573655867282028392E-15, 2.428612866367529932E-14, -8.000000000000000000 ) ) ;
#80320=CARTESIAN_POINT ( 'NONE',  ( -29.86685920354755552, 21.69954338932564397, -6.824999997268814234 ) ) ;
#80428=DIRECTION ( 'NONE',  ( 1.000000000000000000, 0.000000000000000000, 0.000000000000000000 ) ) ;
#80442=FACE_OUTER_BOUND ( 'NONE', #106675, .T. ) ;
#80486=VERTEX_POINT ( 'NONE', #119040 ) ;
#80516=FACE_OUTER_BOUND ( 'NONE', #15853, .T. ) ;
#80561=CARTESIAN_POINT ( 'NONE',  ( -28.82186960331499392, 9.364793116373565596, 149.9000000000000057 ) ) ;
#80585=CARTESIAN_POINT ( 'NONE',  ( 22.44159573604009239, 16.30477369853692693, 148.0750000027312012 ) ) ;
#80591=CARTESIAN_POINT ( 'NONE',  ( -32.00000000000000000, -1.130961319012580892E-14, 92.35000000000000853 ) ) ;
#80677=CARTESIAN_POINT ( 'NONE',  ( 17.14385361876520264, 23.59649016807275856, 146.1750000027311387 ) ) ;
#80697=CARTESIAN_POINT ( 'NONE',  ( 23.48298174826589246, 32.32155151706776053, -6.702157773949822150 ) ) ;
#80733=CARTESIAN_POINT ( 'NONE',  ( -23.31738231874055600, 16.94106989632528837, 149.7999999999999829 ) ) ;
#80801=CARTESIAN_POINT ( 'NONE',  ( -29.86685920354755552, 21.69954338932564397, -6.824999997268814234 ) ) ;
#80802=CARTESIAN_POINT ( 'NONE',  ( -33.75669036400348944, 3.362847000060358305, 99.36731340788949751 ) ) ;
#80827=EDGE_CURVE ( 'NONE', #162507, #188321, #146761, .T. ) ;
#80856=CARTESIAN_POINT ( 'NONE',  ( 35.44379935611745225, -3.753814927773954757, 38.50236686201311187 ) ) ;
#80861=FACE_OUTER_BOUND ( 'NONE', #85615, .T. ) ;
#80914=DIRECTION ( 'NONE',  ( 1.000000000000000000, 0.000000000000000000, 3.709348145883536076E-20 ) ) ;
#81041=CARTESIAN_POINT ( 'NONE',  ( -33.78625674316659655, -2.758724085166798456, 99.76151011743466768 ) ) ;
#81075=CARTESIAN_POINT ( 'NONE',  ( -17.14385361876520264, -23.59649016807271593, 139.1750000027311955 ) ) ;
#81079=CARTESIAN_POINT ( 'NONE',  ( 17.14385361876520264, 23.59649016807275856, 140.1750000027311955 ) ) ;
#81144=CARTESIAN_POINT ( 'NONE',  ( -17.14385361876520975, 23.59649016807275856, 145.0750000027311444 ) ) ;
#81218=CARTESIAN_POINT ( 'NONE',  ( 23.48529157249599919, 32.32473071737754111, -4.449999994537627401 ) ) ;
#81269=CARTESIAN_POINT ( 'NONE',  ( -35.24470855014510562, -4.955302550156636343, 39.34877664276075393 ) ) ;
#81299=CARTESIAN_POINT ( 'NONE',  ( 3.556970738554034288E-15, -38.81732327939057114, -6.124999997268812280 ) ) ;
#81384=CARTESIAN_POINT ( 'NONE',  ( 33.68492599513092500, -4.777136547582187198, 97.74919260172212887 ) ) ;
#81412=VERTEX_POINT ( 'NONE', #102262 ) ;
#81417=CARTESIAN_POINT ( 'NONE',  ( -29.86685920354755197, -21.69954338932560134, -8.424999997268812990 ) ) ;
#81506=CARTESIAN_POINT ( 'NONE',  ( 31.79921067246704780, -6.362367971534556688, 91.02144216243110009 ) ) ;
#81536=CARTESIAN_POINT ( 'NONE',  ( 1.993301997531345292E-15, -30.30510711980685912, 146.5000000000000000 ) ) ;
#81558=CARTESIAN_POINT ( 'NONE',  ( 8.571926809382597767, 26.38167802310806209, 148.2750000027311899 ) ) ;
#81579=CARTESIAN_POINT ( 'NONE',  ( -17.81289503416611097, -24.51734667627696496, 142.2999999999999829 ) ) ;
#81650=CARTESIAN_POINT ( 'NONE',  ( 8.571926809382603096, -26.38167802310801235, 139.4750000027311785 ) ) ;
#81760=ORIENTED_EDGE ( 'NONE', *, *, #113163, .F. ) ;
#81772=CARTESIAN_POINT ( 'NONE',  ( 22.81625015709509441, 31.40387420917330275, -7.324999997268812457 ) ) ;
#81800=EDGE_LOOP ( 'NONE', ( #5769, #171157, #186714, #29673 ) ) ;
#81827=CARTESIAN_POINT ( 'NONE',  ( 34.78522506798721992, -0.4968532545621706098, 52.50000000000000711 ) ) ;
#81834=ORIENTED_EDGE ( 'NONE', *, *, #41647, .T. ) ;
#81855=EDGE_CURVE ( 'NONE', #147696, #108375, #199920, .T. ) ;
#82016=CARTESIAN_POINT ( 'NONE',  ( -33.67956615508440876, -5.223713096473153961, 96.75862529643663379 ) ) ;
#82054=AXIS2_PLACEMENT_3D ( 'NONE', #82060, #99242, #83075 ) ;
#82056=CARTESIAN_POINT ( 'NONE',  ( 27.73933785331498569, 2.768321779492822058E-14, 139.8750000027311842 ) ) ;
#82060=CARTESIAN_POINT ( 'NONE',  ( 0.000000000000000000, 0.000000000000000000, 0.000000000000000000 ) ) ;
#82089=EDGE_CURVE ( 'NONE', #166090, #17663, #167461, .T. ) ;
#82108=TOROIDAL_SURFACE ( 'NONE', #40149, 2.700000000000000622, 0.2000000000000000111 ) ;
#82129=CARTESIAN_POINT ( 'NONE',  ( 17.14385361876520264, -23.59649016807270883, 148.0750000027312012 ) ) ;
#82132=DIRECTION ( 'NONE',  ( 0.000000000000000000, 0.000000000000000000, -1.000000000000000000 ) ) ;
#82177=DIRECTION ( 'NONE',  ( 0.000000000000000000, 0.000000000000000000, -1.000000000000000000 ) ) ;
#82209=CARTESIAN_POINT ( 'NONE',  ( 37.99999999999999289, 2.893978650043524126E-14, -2.749999994537626780 ) ) ;
#82219=PLANE ( 'NONE',  #176125 ) ;
#82260=CARTESIAN_POINT ( 'NONE',  ( 36.91746824999999177, 2.880721459617395097E-14, -6.124999997268813168 ) ) ;
#82294=CARTESIAN_POINT ( 'NONE',  ( -5.950531402560715689E-15, 38.81732327939063509, -1.124999997268813168 ) ) ;
#82385=CARTESIAN_POINT ( 'NONE',  ( 33.67973855159210217, -4.949490125723492007, 97.42538428767439029 ) ) ;
#82412=EDGE_LOOP ( 'NONE', ( #108595, #88475, #31396, #163957, #91192, #127283, #157629, #79806, #26971, #106148, #109218, #173862 ) ) ;
#82417=CARTESIAN_POINT ( 'NONE',  ( 36.91746824999999887, 11.99521256947799053, -9.524999997268812635 ) ) ;
#82461=EDGE_LOOP ( 'NONE', ( #143675, #197422 ) ) ;
#82512=CARTESIAN_POINT ( 'NONE',  ( 31.56677620984796917, -3.765895691706358850, 101.5045925518948593 ) ) ;
#82544=CARTESIAN_POINT ( 'NONE',  ( 17.14385361876520264, -23.59649016807271238, 140.0750000027311728 ) ) ;
#82566=CARTESIAN_POINT ( 'NONE',  ( -5.429308488886486681E-15, 30.30510711980690175, 141.7500000054623683 ) ) ;
#82671=CARTESIAN_POINT ( 'NONE',  ( 1.993301997531345686E-15, -30.30510711980685556, 148.5000000000000000 ) ) ;
#82675=CARTESIAN_POINT ( 'NONE',  ( 36.89607807516674143, -1.430951785632629036, 50.32279621992266527 ) ) ;
#82716=PRODUCT_DEFINITION_CONTEXT ( 'detailed design', #57191, 'design' ) ;
#82760=DIRECTION ( 'NONE',  ( -1.000000000000000000, 0.000000000000000000, 0.000000000000000000 ) ) ;
#82780=CARTESIAN_POINT ( 'NONE',  ( -11.40812507854755609, 35.11059874428196537, -5.024999997268813523 ) ) ;
#82818=VERTEX_POINT ( 'NONE', #143264 ) ;
#82831=CARTESIAN_POINT ( 'NONE',  ( -40.00200000000003087, -5.510910596163089556E-15, 37.50000000000000000 ) ) ;
#82838=CARTESIAN_POINT ( 'NONE',  ( 28.82186960331498327, 2.428612866367529932E-14, 150.0000000000000000 ) ) ;
#82853=CARTESIAN_POINT ( 'NONE',  ( 28.82186960331477010, -9.364793116373819615, 140.9000000000000057 ) ) ;
#82863=CARTESIAN_POINT ( 'NONE',  ( 11.74149087413294268, 36.13659316521247433, -4.602157773949822506 ) ) ;
#82870=DIRECTION ( 'NONE',  ( 1.000000000000000000, -0.000000000000000000, -0.000000000000000000 ) ) ;
#82881=CARTESIAN_POINT ( 'NONE',  ( -32.00000000000000000, -5.510910596163089556E-15, 45.00000000000000000 ) ) ;
#83053=EDGE_LOOP ( 'NONE', ( #163427, #130261, #89087, #150693 ) ) ;
#83070=CARTESIAN_POINT ( 'NONE',  ( -27.73933785331498925, 2.428612866367529932E-14, 147.3750000027311842 ) ) ;
#83075=DIRECTION ( 'NONE',  ( 1.000000000000000000, 0.000000000000000000, 0.000000000000000000 ) ) ;
#83104=FACE_OUTER_BOUND ( 'NONE', #32644, .T. ) ;
#83108=ORIENTED_EDGE ( 'NONE', *, *, #99422, .T. ) ;
#83144=CARTESIAN_POINT ( 'NONE',  ( 1.784210473542230573E-15, -29.16686587814331588, 145.8750000027311557 ) ) ;
#83221=CARTESIAN_POINT ( 'NONE',  ( -30.74264578624800492, 22.33583958711400186, -5.949999994537626513 ) ) ;
#83256=CARTESIAN_POINT ( 'NONE',  ( 31.45250202946434825, 4.971043627493195949, 100.6372900316468986 ) ) ;
#83259=ORIENTED_EDGE ( 'NONE', *, *, #139684, .T. ) ;
#83261=DIRECTION ( 'NONE',  ( 0.06104853953485701173, 0.000000000000000000, -0.9981347984218670311 ) ) ;
#83272=CARTESIAN_POINT ( 'NONE',  ( 3.556970738554033499E-15, -38.81732327939057825, -6.624999997268814056 ) ) ;
#83274=CARTESIAN_POINT ( 'NONE',  ( -35.63774670715083204, -1.952809719854284198, 37.74170157406051374 ) ) ;
#83302=CARTESIAN_POINT ( 'NONE',  ( 11.40812507854755253, -35.11059874428192273, -6.024999997268814411 ) ) ;
#83417=VERTEX_POINT ( 'NONE', #160868 ) ;
#83422=CARTESIAN_POINT ( 'NONE',  ( 30.74264578624799782, 22.33583958711400541, -0.7999999999999999334 ) ) ;
#83460=ADVANCED_FACE ( 'NONE', ( #4175 ), #128514, .T. ) ;
#83487=ADVANCED_FACE ( 'NONE', ( #99179 ), #112364, .F. ) ;
#83513=CARTESIAN_POINT ( 'NONE',  ( 32.36699822888682121, -3.753862658156253751, 88.50241378327223174 ) ) ;
#83542=CARTESIAN_POINT ( 'NONE',  ( -17.81289503416611097, -24.51734667627696496, 140.2999999999999545 ) ) ;
#83566=CARTESIAN_POINT ( 'NONE',  ( -5.429308488886486681E-15, 30.30510711980690175, 139.7500000054623683 ) ) ;
#83676=FACE_BOUND ( 'NONE', #142403, .T. ) ;
#83778=CARTESIAN_POINT ( 'NONE',  ( -29.86685920354755197, -21.69954338932560134, -8.424999997268812990 ) ) ;
#83779=CARTESIAN_POINT ( 'NONE',  ( -33.72265478998904342, 5.501106843017430137, 95.34580731367213957 ) ) ;
#83780=CARTESIAN_POINT ( 'NONE',  ( -40.00000000000002842, 1.938754146708588393E-14, 0.000000000000000000 ) ) ;
#83828=DIRECTION ( 'NONE',  ( 0.000000000000000000, 0.000000000000000000, 1.000000000000000000 ) ) ;
#83841=VERTEX_POINT ( 'NONE', #29166 ) ;
#83852=DIRECTION ( 'NONE',  ( -0.000000000000000000, -0.000000000000000000, -1.000000000000000000 ) ) ;
#83912=DIRECTION ( 'NONE',  ( 0.000000000000000000, 0.000000000000000000, 1.000000000000000000 ) ) ;
#83913=VECTOR ( 'NONE', #135052, 1000.000000000000227 ) ;
#83980=ADVANCED_FACE ( 'NONE', ( #199993 ), #61460, .F. ) ;
#83983=CARTESIAN_POINT ( 'NONE',  ( 34.12434206616184440, 14.08647367304311260, -8.000000000000001776 ) ) ;
#84064=CARTESIAN_POINT ( 'NONE',  ( -32.64453336272028139, 2.028832619897439204E-14, 87.50000000000000000 ) ) ;
#84068=CARTESIAN_POINT ( 'NONE',  ( -17.14385361876520619, 23.59649016807275856, 143.0750000027311444 ) ) ;
#84079=ORIENTED_EDGE ( 'NONE', *, *, #72341, .F. ) ;
#84139=CARTESIAN_POINT ( 'NONE',  ( -8.571926809382608425, 26.38167802310805854, 148.4750000027311785 ) ) ;
#84142=CARTESIAN_POINT ( 'NONE',  ( 37.99626262588765258, 2.893932880411085066E-14, 6.432029388270255055E-14 ) ) ;
#84214=CARTESIAN_POINT ( 'NONE',  ( 30.74264578624800137, -22.33583958711395212, -4.949999994537626513 ) ) ;
#84230=DIRECTION ( 'NONE',  ( 0.8660254037844410391, -0.000000000000000000, -0.4999999999999958367 ) ) ;
#84250=CARTESIAN_POINT ( 'NONE',  ( 31.25711108810727623, 6.845500155895383187, 98.07395821223764187 ) ) ;
#84253=ORIENTED_EDGE ( 'NONE', *, *, #45012, .F. ) ;
#84266=CARTESIAN_POINT ( 'NONE',  ( 36.91746824999999177, 2.880721459617395097E-14, -2.124999997268813168 ) ) ;
#84268=CARTESIAN_POINT ( 'NONE',  ( -34.38809498607734838, -6.739667044264582074, 48.29962152465627412 ) ) ;
#84270=CARTESIAN_POINT ( 'NONE',  ( -35.99626262588765968, 2.428612866367529932E-14, 2.000000000000000000 ) ) ;
#84298=CARTESIAN_POINT ( 'NONE',  ( -11.40812507854754720, -35.11059874428192273, -2.224999997268813701 ) ) ;
#84363=ORIENTED_EDGE ( 'NONE', *, *, #180435, .F. ) ;
#84420=CARTESIAN_POINT ( 'NONE',  ( 36.91746825000000598, -11.99521256947793546, -7.724999997268812812 ) ) ;
#84466=CARTESIAN_POINT ( 'NONE',  ( -30.00000000000000000, -5.510910596163089556E-15, 45.00000000000000000 ) ) ;
#84509=CARTESIAN_POINT ( 'NONE',  ( 30.73962218707677252, 22.33364281372847060, -6.547842220587804185 ) ) ;
#84527=ORIENTED_EDGE ( 'NONE', *, *, #49302, .T. ) ;
#84538=CARTESIAN_POINT ( 'NONE',  ( 1.993301997531345292E-15, -30.30510711980685912, 140.5000000000000000 ) ) ;
#84561=CARTESIAN_POINT ( 'NONE',  ( 22.44159573604009594, -16.30477369853687364, 143.6750000027311671 ) ) ;
#84567=CARTESIAN_POINT ( 'NONE',  ( -28.82186960331499037, 2.428612866367529932E-14, 144.2500000054623683 ) ) ;
#84596=PRODUCT_CONTEXT ( 'NONE', #151378, 'mechanical' ) ;
#84598=ORIENTED_EDGE ( 'NONE', *, *, #156164, .T. ) ;
#84656=CARTESIAN_POINT ( 'NONE',  ( 27.73933785331498925, -9.013057229001034898, 139.7750000027311899 ) ) ;
#84774=CARTESIAN_POINT ( 'NONE',  ( 27.73933785331498214, 9.013057229001095294, 148.4750000027311785 ) ) ;
#84783=ORIENTED_EDGE ( 'NONE', *, *, #71047, .F. ) ;
#84818=DIRECTION ( 'NONE',  ( 1.000000000000000000, 0.000000000000000000, 0.000000000000000000 ) ) ;
#84977=CARTESIAN_POINT ( 'NONE',  ( 31.37807670187659070, -19.48766232597224501, -7.999999999999996447 ) ) ;
#85051=AXIS2_PLACEMENT_3D ( 'NONE', #167235, #166244, #179434 ) ;
#85062=CARTESIAN_POINT ( 'NONE',  ( -32.42844225013699599, -3.321486864536487893, 88.27111922316775861 ) ) ;
#85066=CARTESIAN_POINT ( 'NONE',  ( -8.571926809382601320, -26.38167802310801591, 143.7750000027311899 ) ) ;
#85078=VERTEX_POINT ( 'NONE', #126123 ) ;
#85139=CARTESIAN_POINT ( 'NONE',  ( 30.00000000000000711, -1.071565949253934124E-14, 102.5000000000000142 ) ) ;
#85141=CARTESIAN_POINT ( 'NONE',  ( 22.44159573604009239, 16.30477369853692693, 148.0750000027312012 ) ) ;
#85217=CARTESIAN_POINT ( 'NONE',  ( -23.48529157249599919, -32.32473071737750558, -7.449999994537624737 ) ) ;
#85230=ORIENTED_EDGE ( 'NONE', *, *, #178148, .F. ) ;
#85254=CARTESIAN_POINT ( 'NONE',  ( 31.91717023173579193, 5.953136853522610572, 90.41250038490909446 ) ) ;
#85257=ORIENTED_EDGE ( 'NONE', *, *, #185806, .F. ) ;
#85268=CARTESIAN_POINT ( 'NONE',  ( 37.52489844900623694, 1.772207303729227856, 39.79021962610334384 ) ) ;
#85271=CARTESIAN_POINT ( 'NONE',  ( -34.72618186072388369, -2.417897188208103731, 52.10384489098235861 ) ) ;
#85294=DIRECTION ( 'NONE',  ( 0.000000000000000000, 0.000000000000000000, 1.000000000000000000 ) ) ;
#85299=CARTESIAN_POINT ( 'NONE',  ( -37.54602941011386008, 1.427078192699135162, 39.68530545529164755 ) ) ;
#85369=AXIS2_PLACEMENT_3D ( 'NONE', #3673, #175525, #126036 ) ;
#85416=ORIENTED_EDGE ( 'NONE', *, *, #65731, .F. ) ;
#85427=CARTESIAN_POINT ( 'NONE',  ( 36.91746824999999887, 11.99521256947799053, -5.524999997268812635 ) ) ;
#85524=EDGE_LOOP ( 'NONE', ( #23178, #49451 ) ) ;
#85530=VECTOR ( 'NONE', #180629, 1000.000000000000000 ) ;
#85536=ORIENTED_EDGE ( 'NONE', *, *, #123690, .F. ) ;
#85575=AXIS2_PLACEMENT_3D ( 'NONE', #145949, #132790, #103460 ) ;
#85583=CARTESIAN_POINT ( 'NONE',  ( -28.82186960331499037, 2.781578969918950771E-14, 139.9999999999999716 ) ) ;
#85615=EDGE_LOOP ( 'NONE', ( #15998, #72164, #195272, #9445 ) ) ;
#85684=CARTESIAN_POINT ( 'NONE',  ( 36.76875311564133142, -5.017346702420294235, 47.26027925686761932 ) ) ;
#85759=CARTESIAN_POINT ( 'NONE',  ( 24.68382089499486653, 27.82722013636965031, -8.000000000000003553 ) ) ;
#85762=CARTESIAN_POINT ( 'NONE',  ( 28.82186960331486958, -9.364793116373689941, 144.9000000000000057 ) ) ;
#85993=CARTESIAN_POINT ( 'NONE',  ( 24.42644823724867464, -27.78615197534793069, -8.000000000000001776 ) ) ;
#86041=DIRECTION ( 'NONE',  ( 0.06104853953485701173, 0.000000000000000000, -0.9981347984218670311 ) ) ;
#86042=CARTESIAN_POINT ( 'NONE',  ( -33.76764775315835010, -5.498935319396523802, 94.62547034095167930 ) ) ;
#86053=CARTESIAN_POINT ( 'NONE',  ( 31.99999999999970868, 4.794320942884877174E-13, 42.30000000000021743 ) ) ;
#86062=EDGE_LOOP ( 'NONE', ( #94788, #106290, #153550, #107477 ) ) ;
#86079=CARTESIAN_POINT ( 'NONE',  ( 17.14385361876520264, 23.59649016807275856, 146.6750000027311671 ) ) ;
#86085=CARTESIAN_POINT ( 'NONE',  ( 11.74149087413295156, -36.13659316521243881, -5.147842220587802942 ) ) ;
#86156=CARTESIAN_POINT ( 'NONE',  ( 27.73933785331498569, 9.013057229001093518, 147.9750000027311501 ) ) ;
#86176=DIRECTION ( 'NONE',  ( 0.000000000000000000, 0.000000000000000000, 1.000000000000000000 ) ) ;
#86229=CARTESIAN_POINT ( 'NONE',  ( -6.020228577223754586E-15, 39.95556452105416412, -10.24999999453762456 ) ) ;
#86265=CARTESIAN_POINT ( 'NONE',  ( 31.69373074887816344, 1.710217150889069782, 102.3065243757510956 ) ) ;
#86311=CARTESIAN_POINT ( 'NONE',  ( 29.86685920354754487, 21.69954338932564752, -7.424999997268813878 ) ) ;
#86366=LINE ( 'NONE', #164225, #194923 ) ;
#86436=CARTESIAN_POINT ( 'NONE',  ( 23.48529157249599919, 32.32473071737754111, -4.699999999999999289 ) ) ;
#86473=TOROIDAL_SURFACE ( 'NONE', #144602, 2.700000000000000622, 0.2000000000000000111 ) ;
#86554=CARTESIAN_POINT ( 'NONE',  ( -23.31738231874055245, -16.94106989632524574, 144.1999999999999886 ) ) ;
#86556=CARTESIAN_POINT ( 'NONE',  ( 1.993301997531345686E-15, -30.30510711980685556, 138.7500000054623683 ) ) ;
#86589=PRESENTATION_STYLE_ASSIGNMENT (( #161434 ) ) ;
#86608=CARTESIAN_POINT ( 'NONE',  ( 11.74149087413294268, 36.13659316521247433, -0.6021577739498229498 ) ) ;
#86685=CARTESIAN_POINT ( 'NONE',  ( 37.36625173109577958, -3.353228347065799309, 40.62582701645503391 ) ) ;
#86746=ADVANCED_FACE ( 'NONE', ( #92554 ), #95539, .T. ) ;
#86759=CARTESIAN_POINT ( 'NONE',  ( -20.62648400444483343, 31.81274089240160308, -7.999999999999996447 ) ) ;
#86778=CARTESIAN_POINT ( 'NONE',  ( -37.99626262588766679, 2.428612866367529932E-14, -5.747842220587803475 ) ) ;
#86813=CARTESIAN_POINT ( 'NONE',  ( -34.52932710190716392, 5.142084072295503461, 50.46524955901336540 ) ) ;
#86839=VECTOR ( 'NONE', #173072, 1000.000000000000000 ) ;
#86851=DIRECTION ( 'NONE',  ( 0.000000000000000000, 0.000000000000000000, -1.000000000000000000 ) ) ;
#87043=CARTESIAN_POINT ( 'NONE',  ( -34.11707783341799427, -4.368959606072635005, 91.63974055655047835 ) ) ;
#87082=CARTESIAN_POINT ( 'NONE',  ( -22.44159573604009950, -16.30477369853688430, 145.5750000027311728 ) ) ;
#87087=CARTESIAN_POINT ( 'NONE',  ( 3.765340386950246872E-15, -39.95163481335715971, -7.247842220587804363 ) ) ;
#87159=CARTESIAN_POINT ( 'NONE',  ( 8.571926809382603096, -26.38167802310801235, 141.9750000027312069 ) ) ;
#87233=CARTESIAN_POINT ( 'NONE',  ( 37.99999999999999289, 2.893978650043524126E-14, -10.74999999453762811 ) ) ;
#87244=DIRECTION ( 'NONE',  ( -1.000000000000000000, -0.000000000000000000, -0.000000000000000000 ) ) ;
#87400=DIRECTION ( 'NONE',  ( 0.000000000000000000, 0.000000000000000000, -1.000000000000000000 ) ) ;
#87423=CARTESIAN_POINT ( 'NONE',  ( 31.72709406046299918, -1.071565338629617092E-14, 102.5000000000000142 ) ) ;
#87438=CARTESIAN_POINT ( 'NONE',  ( -30.74264578624800492, 22.33583958711400186, -4.200000000000000178 ) ) ;
#87546=DIRECTION ( 'NONE',  ( -7.709882115452493155E-15, 0.000000000000000000, 1.000000000000000000 ) ) ;
#87554=CARTESIAN_POINT ( 'NONE',  ( 17.81289503416610742, 24.51734667627700404, 141.2999999999999829 ) ) ;
#87556=CARTESIAN_POINT ( 'NONE',  ( -28.82186960331499037, 2.428612866367529932E-14, 144.2500000054623683 ) ) ;
#87587=FILL_AREA_STYLE_COLOUR ( '', #27553 ) ;
#87605=CARTESIAN_POINT ( 'NONE',  ( -23.48298174826590667, 32.32155151706776053, -0.3021577739498228499 ) ) ;
#87752=CARTESIAN_POINT ( 'NONE',  ( -24.35524355471601510, 29.14552502360113095, -7.999999999999998224 ) ) ;
#87755=DIRECTION ( 'NONE',  ( 0.000000000000000000, 0.000000000000000000, -1.000000000000000000 ) ) ;
#87782=CARTESIAN_POINT ( 'NONE',  ( -5.359611314223446995E-15, 29.16686587814335496, 148.8750000027311842 ) ) ;
#87788=DIRECTION ( 'NONE',  ( 0.000000000000000000, 0.000000000000000000, -1.000000000000000000 ) ) ;
#88000=ORIENTED_EDGE ( 'NONE', *, *, #69759, .F. ) ;
#88018=ORIENTED_EDGE ( 'NONE', *, *, #66474, .F. ) ;
#88033=CARTESIAN_POINT ( 'NONE',  ( -25.76063610039751595, -27.36442781147108150, -7.999999999999992895 ) ) ;
#88068=CARTESIAN_POINT ( 'NONE',  ( -31.33613174426653458, -7.485780765379336010, 94.47638157584334806 ) ) ;
#88078=SURFACE_STYLE_FILL_AREA ( #91043 ) ;
#88219=CARTESIAN_POINT ( 'NONE',  ( -36.91746825000001309, -11.99521256947794789, -3.024999997268812635 ) ) ;
#88230=ORIENTED_EDGE ( 'NONE', *, *, #72705, .F. ) ;
#88270=CARTESIAN_POINT ( 'NONE',  ( 36.91128768240056246, 2.428612879436746321E-14, 50.50000000000002842 ) ) ;
#88273=CARTESIAN_POINT ( 'NONE',  ( -34.41611627805855278, -6.381310488372556655, 48.94841969467692877 ) ) ;
#88283=CARTESIAN_POINT ( 'NONE',  ( 67.00000000000000000, -1.163414459189985801E-14, 95.00000000000000000 ) ) ;
#88288=ORIENTED_EDGE ( 'NONE', *, *, #126225, .T. ) ;
#88314=CARTESIAN_POINT ( 'NONE',  ( -27.73933785331498925, -9.013057229001049109, 144.9750000027312069 ) ) ;
#88378=LINE ( 'NONE', #150072, #23600 ) ;
#88382=CARTESIAN_POINT ( 'NONE',  ( 8.906447517083057264, -27.41122689804191026, 146.5999999999999943 ) ) ;
#88427=CARTESIAN_POINT ( 'NONE',  ( -38.00000000000001421, 12.34694845685046438, -2.099999999999999645 ) ) ;
#88475=ORIENTED_EDGE ( 'NONE', *, *, #55774, .T. ) ;
#88483=B_SPLINE_CURVE_WITH_KNOTS ( 'NONE', 3,
 ( #192501, #133824, #115658, #196516, #85299, #180353, #41822, #103489, #12491, #74153, #54981, #165167, #149990, #11496, #100476, #73167, #162155, #57987, #194505, #55978, #119658, #42819, #104482, #166166, #183313, #75125, #138776, #32604, #29625, #184303, #92268, #136793, #90289, #59951, #78091, #152948, #31610, #257, #107436, #13461, #94257, #93260 ),
 .UNSPECIFIED., .F., .F.,
 ( 4, 2, 2, 2, 2, 2, 2, 2, 2, 2, 2, 2, 2, 2, 2, 2, 2, 2, 2, 2, 4 ),
 ( 0.004226304204691694322, 0.005303825792898751723, 0.005842586587002280424, 0.006381347381105809992, 0.007458868969312869128, 0.008536390557519929131, 0.009613912145726988268, 0.01069143373393404740, 0.01123019452803758825, 0.01176895532214112562, 0.01284647691034820384, 0.01392399849855528206, 0.01446275929265882290, 0.01500152008676236375, 0.01607904167496944370, 0.01715656326317651845, 0.01823408485138360013, 0.01877284564548713924, 0.01931160643959067488, 0.02038912802779774616, 0.02146664961600481397 ),
 .UNSPECIFIED. ) ;
#88527=ORIENTED_EDGE ( 'NONE', *, *, #141815, .T. ) ;
#88550=CARTESIAN_POINT ( 'NONE',  ( -5.429308488886486681E-15, 30.30510711980690175, 143.7500000054623399 ) ) ;
#88614=ORIENTED_EDGE ( 'NONE', *, *, #68093, .F. ) ;
#88624=AXIS2_PLACEMENT_3D ( 'NONE', #48582, #82870, #94064 ) ;
#88669=DIRECTION ( 'NONE',  ( 0.000000000000000000, 0.000000000000000000, -1.000000000000000000 ) ) ;
#88682=CIRCLE ( 'NONE', #140340, 7.500000000000000000 ) ;
#88726=CIRCLE ( 'NONE', #98352, 2.699999999999993960 ) ;
#88756=CARTESIAN_POINT ( 'NONE',  ( -3.417157638698077982, 37.49351071327306784, -7.999999999999996447 ) ) ;
#88759=DIRECTION ( 'NONE',  ( -1.000000000000000000, 0.000000000000000000, 0.000000000000000000 ) ) ;
#88785=CARTESIAN_POINT ( 'NONE',  ( 22.44159573604009594, -16.30477369853687364, 148.1750000027311671 ) ) ;
#88862=STYLED_ITEM ( 'NONE', ( #86589 ), #142731 ) ;
#88920=CARTESIAN_POINT ( 'NONE',  ( -30.73962218707678318, 22.33364281372846705, -3.947842220587803208 ) ) ;
#89029=CARTESIAN_POINT ( 'NONE',  ( -36.91746825000000598, 2.428612866367529932E-14, -1.124999997268813390 ) ) ;
#89036=CARTESIAN_POINT ( 'NONE',  ( -34.37111623004060590, -2.754365613946270219, 90.23597232697538573 ) ) ;
#89048=CARTESIAN_POINT ( 'NONE',  ( -11.40812507854755609, 35.11059874428196537, -3.524999997268813523 ) ) ;
#89080=( LENGTH_UNIT ( ) NAMED_UNIT ( * ) SI_UNIT ( .MILLI., .METRE. ) );
#89087=ORIENTED_EDGE ( 'NONE', *, *, #4758, .T. ) ;
#89220=CARTESIAN_POINT ( 'NONE',  ( -38.00000000000001421, 12.34694845685046438, -9.849999994537625980 ) ) ;
#89269=CARTESIAN_POINT ( 'NONE',  ( 31.72709406046299208, -0.4963711039037253525, 102.5000000000000284 ) ) ;
#89276=CARTESIAN_POINT ( 'NONE',  ( 36.88729982035407318, 1.776435236410516039, 50.21758054017369233 ) ) ;
#89288=DIRECTION ( 'NONE',  ( 0.000000000000000000, 0.000000000000000000, -1.000000000000000000 ) ) ;
#89307=CARTESIAN_POINT ( 'NONE',  ( 22.81625015709509441, 31.40387420917330275, -7.324999997268812457 ) ) ;
#89313=CARTESIAN_POINT ( 'NONE',  ( 8.571926809382597767, 26.38167802310806209, 144.2750000027311899 ) ) ;
#89318=CARTESIAN_POINT ( 'NONE',  ( -17.14385361876520619, 23.59649016807275856, 144.5750000027312012 ) ) ;
#89327=ORIENTED_EDGE ( 'NONE', *, *, #141481, .F. ) ;
#89344=EDGE_CURVE ( 'NONE', #72946, #56681, #171294, .T. ) ;
#89429=CARTESIAN_POINT ( 'NONE',  ( -11.74264578624799782, -36.14014761921581709, -3.600000000000000533 ) ) ;
#89476=ORIENTED_EDGE ( 'NONE', *, *, #139684, .F. ) ;
#89479=ORIENTED_EDGE ( 'NONE', *, *, #2987, .T. ) ;
#89480=CARTESIAN_POINT ( 'NONE',  ( 35.70266437024451278, 0.2453497911276426302, 37.50000000000002132 ) ) ;
#89491=ORIENTED_EDGE ( 'NONE', *, *, #54770, .T. ) ;
#89527=VERTEX_POINT ( 'NONE', #162263 ) ;
#89675=VECTOR ( 'NONE', #47233, 1000.000000000000114 ) ;
#89680=EDGE_CURVE ( 'NONE', #199732, #122026, #48616, .T. ) ;
#89682=CARTESIAN_POINT ( 'NONE',  ( -26.63278688795740834, 27.10001173645601114, -8.000000000000000000 ) ) ;
#89751=CARTESIAN_POINT ( 'NONE',  ( 6.465454559173637428, 36.91613723712380590, -7.999999999999996447 ) ) ;
#89762=CIRCLE ( 'NONE', #12284, 2.700000000000001066 ) ;
#89782=CARTESIAN_POINT ( 'NONE',  ( 27.73933785331498214, 9.013057229001095294, 144.4750000027311501 ) ) ;
#89861=VERTEX_POINT ( 'NONE', #87423 ) ;
#89885=CARTESIAN_POINT ( 'NONE',  ( 3.765340386950246872E-15, -39.95163481335715971, -3.502157773949823305 ) ) ;
#89980=CARTESIAN_POINT ( 'NONE',  ( -37.99626262588766679, 2.428612866367529932E-14, -8.000000000000000000 ) ) ;
#90022=CARTESIAN_POINT ( 'NONE',  ( -36.91746825000000598, 2.428612866367529932E-14, -7.124999997268813168 ) ) ;
#90028=CARTESIAN_POINT ( 'NONE',  ( -28.91127206596838306, -24.07972945715490809, -8.000000000000003553 ) ) ;
#90067=CARTESIAN_POINT ( 'NONE',  ( 27.73933785331498569, 2.768321779492822058E-14, 140.3750000027311842 ) ) ;
#90078=( BOUNDED_CURVE ( )  B_SPLINE_CURVE ( 2, ( #168838, #30343, #93989, #18167, #61656, #187036, #123324, #31339, #79823, #185018, #157665 ),
 .UNSPECIFIED., .F., .F. ) 
 B_SPLINE_CURVE_WITH_KNOTS ( ( 3, 2, 2, 2, 2, 3 ),
 ( 0.09999999999999997780, 0.1199999999999999678, 0.1399999999999999856, 0.1600000000000000033, 0.1799999999999999933, 0.2000000000000000111 ),
 .UNSPECIFIED. ) 
 CURVE ( )  GEOMETRIC_REPRESENTATION_ITEM ( )  RATIONAL_B_SPLINE_CURVE ( ( 1.000000000000000000, 0.9510565162951533091, 1.000000000000000000, 0.9510565162951535312, 1.000000000000000000, 0.9510565162951535312, 1.000000000000000000, 0.9510565162951535312, 1.000000000000000000, 0.9510565162951535312, 1.000000000000000000 ) ) 
 REPRESENTATION_ITEM ( '' )  );
#90127=CARTESIAN_POINT ( 'NONE',  ( -3.573655867282028392E-15, 2.428612866367529932E-14, 139.9999999999999716 ) ) ;
#90207=CARTESIAN_POINT ( 'NONE',  ( -23.48529157249599919, -32.32473071737750558, -11.44999999453762385 ) ) ;
#90232=ADVANCED_FACE ( 'NONE', ( #131932 ), #174476, .T. ) ;
#90252=CARTESIAN_POINT ( 'NONE',  ( 31.72709406046299918, -1.071565338629617092E-14, 102.5000000000000142 ) ) ;
#90289=CARTESIAN_POINT ( 'NONE',  ( -36.82860559483759033, 3.362349505172651298, 49.36759404993757983 ) ) ;
#90295=CARTESIAN_POINT ( 'NONE',  ( 22.44159573604009239, 16.30477369853692693, 144.0750000027311728 ) ) ;
#90300=CARTESIAN_POINT ( 'NONE',  ( 27.73933785331498569, 2.768321779492822058E-14, 141.8750000027311842 ) ) ;
#90331=ORIENTED_EDGE ( 'NONE', *, *, #32497, .T. ) ;
#90510=ORIENTED_EDGE ( 'NONE', *, *, #18810, .T. ) ;
#90549=ORIENTED_EDGE ( 'NONE', *, *, #142462, .T. ) ;
#90664=CARTESIAN_POINT ( 'NONE',  ( -37.99626262588766679, 2.428612866367529932E-14, -7.747842220587803475 ) ) ;
#90715=CARTESIAN_POINT ( 'NONE',  ( -3.573655867282028392E-15, 2.428612866367529932E-14, -8.000000000000000000 ) ) ;
#90729=CARTESIAN_POINT ( 'NONE',  ( 28.82186960331498327, 2.428612866367529932E-14, 139.9999999999999716 ) ) ;
#90749=FACE_BOUND ( 'NONE', #93809, .T. ) ;
#90760=CARTESIAN_POINT ( 'NONE',  ( -5.359611314223446995E-15, 29.16686587814335496, 146.8750000027311273 ) ) ;
#90767=CARTESIAN_POINT ( 'NONE',  ( 32.00000000000000000, -1.163414459189985801E-14, 95.00000000000000000 ) ) ;
#90783=CARTESIAN_POINT ( 'NONE',  ( 17.81289503416611453, -24.51734667627695785, 146.9500000054623570 ) ) ;
#90906=ADVANCED_FACE ( 'NONE', ( #76215 ), #107540, .T. ) ;
#90950=CARTESIAN_POINT ( 'NONE',  ( -28.82186960331499037, 2.428612866367529932E-14, 150.0000000000000000 ) ) ;
#90959=VERTEX_POINT ( 'NONE', #169216 ) ;
#90992=CARTESIAN_POINT ( 'NONE',  ( 22.81625015709510151, -31.40387420917324590, -1.924999997268813434 ) ) ;
#90993=CARTESIAN_POINT ( 'NONE',  ( -34.37139930337508531, 2.751904643975403797, 90.23455903727463578 ) ) ;
#90999=CARTESIAN_POINT ( 'NONE',  ( 33.85315667487628133, 2.428612866512670557E-14, 100.5000000000010232 ) ) ;
#91011=CARTESIAN_POINT ( 'NONE',  ( -11.40812507854755609, 35.11059874428196537, -5.524999997268813523 ) ) ;
#91043=FILL_AREA_STYLE ('',( #135601 ) ) ;
#91050=ORIENTED_EDGE ( 'NONE', *, *, #3703, .T. ) ;
#91073=ORIENTED_EDGE ( 'NONE', *, *, #103944, .T. ) ;
#91095=CARTESIAN_POINT ( 'NONE',  ( -32.36630342937671401, 3.758454152357579403, 88.50505952879542804 ) ) ;
#91179=CARTESIAN_POINT ( 'NONE',  ( -36.91746825000000598, 2.428612866367529932E-14, -5.124999997268813168 ) ) ;
#91192=ORIENTED_EDGE ( 'NONE', *, *, #72915, .T. ) ;
#91196=CARTESIAN_POINT ( 'NONE',  ( 28.82186960331498327, 2.428612866367529932E-14, 139.9999999999999716 ) ) ;
#91231=( BOUNDED_CURVE ( )  B_SPLINE_CURVE ( 2, ( #120867, #182567, #162395, #196757, #25912, #86556, #193755, #132066, #195764, #72398, #135081 ),
 .UNSPECIFIED., .F., .F. ) 
 B_SPLINE_CURVE_WITH_KNOTS ( ( 3, 2, 2, 2, 2, 3 ),
 ( 0.9000000000000007994, 0.9200000000000007061, 0.9400000000000003908, 0.9600000000000002975, 0.9800000000000002043, 1.000000000000000000 ),
 .UNSPECIFIED. ) 
 CURVE ( )  GEOMETRIC_REPRESENTATION_ITEM ( )  RATIONAL_B_SPLINE_CURVE ( ( 0.9999999999999981126, 0.9510565162951554186, 1.000000000000000000, 0.9510565162951535312, 1.000000000000000000, 0.9510565162951535312, 1.000000000000000000, 0.9510565162951535312, 1.000000000000000000, 0.9510565162951535312, 1.000000000000000000 ) ) 
 REPRESENTATION_ITEM ( '' )  );
#91264=CARTESIAN_POINT ( 'NONE',  ( -22.44159573604010305, 16.30477369853692338, 148.6750000027311671 ) ) ;
#91269=CARTESIAN_POINT ( 'NONE',  ( -22.44159573604010305, 16.30477369853692338, 146.6750000027311671 ) ) ;
#91381=CARTESIAN_POINT ( 'NONE',  ( 30.74264578624800137, -22.33583958711395212, -9.199999999999999289 ) ) ;
#91402=VECTOR ( 'NONE', #142591, 1000.000000000000000 ) ;
#91434=CARTESIAN_POINT ( 'NONE',  ( 35.09778042078743709, 5.635567127521242448, 40.04523299337174080 ) ) ;
#91503=CARTESIAN_POINT ( 'NONE',  ( 17.81289503416610742, 24.51734667627700404, 147.5500000054623513 ) ) ;
#91600=ADVANCED_FACE ( 'NONE', ( #37423 ), #99083, .F. ) ;
#91711=CARTESIAN_POINT ( 'NONE',  ( -37.06950394710835184, -4.940869137700751423, 42.55762898535584071 ) ) ;
#91727=ORIENTED_EDGE ( 'NONE', *, *, #89344, .T. ) ;
#91741=CARTESIAN_POINT ( 'NONE',  ( 22.44159573604009594, -16.30477369853687364, 146.1750000027311671 ) ) ;
#91765=CARTESIAN_POINT ( 'NONE',  ( 28.82186960331498327, 2.781578969918950771E-14, 147.2500000054623683 ) ) ;
#91788=CARTESIAN_POINT ( 'NONE',  ( 28.82186960331498327, 2.781578969918950771E-14, 143.0000000000000000 ) ) ;
#91856=CARTESIAN_POINT ( 'NONE',  ( 22.44159573604009239, 16.30477369853692693, 142.0750000027311728 ) ) ;
#91865=CIRCLE ( 'NONE', #4691, 30.82560697742735556 ) ;
#91871=CARTESIAN_POINT ( 'NONE',  ( -28.82186960331483760, 9.364793116373787640, 142.1500000054624024 ) ) ;
#91874=CARTESIAN_POINT ( 'NONE',  ( -30.73962218707678673, 22.33364281372846705, -6.202157773949823927 ) ) ;
#91970=EDGE_LOOP ( 'NONE', ( #177699, #19597 ) ) ;
#91981=CARTESIAN_POINT ( 'NONE',  ( 11.40812507854754365, 35.11059874428196537, -9.724999997268813701 ) ) ;
#91982=CARTESIAN_POINT ( 'NONE',  ( -34.02686120844016671, 4.767814797156207263, 92.23495037107731775 ) ) ;
#91999=CARTESIAN_POINT ( 'NONE',  ( 22.81625015709510151, -31.40387420917324590, -4.424999997268812990 ) ) ;
#92008=EDGE_LOOP ( 'NONE', ( #170051, #137333, #179464, #104029 ) ) ;
#92043=DIRECTION ( 'NONE',  ( 0.000000000000000000, 0.000000000000000000, -1.000000000000000000 ) ) ;
#92080=CARTESIAN_POINT ( 'NONE',  ( -23.31738231874055245, -16.94106989632524574, 142.4500000054623854 ) ) ;
#92091=CARTESIAN_POINT ( 'NONE',  ( -31.80025110837587832, 6.358902984670137037, 91.01589400111389239 ) ) ;
#92173=AXIS2_PLACEMENT_3D ( 'NONE', #49542, #92043, #111204 ) ;
#92181=CARTESIAN_POINT ( 'NONE',  ( 36.91746824999999177, 2.880721459617395097E-14, -8.124999997268814056 ) ) ;
#92231=B_SPLINE_CURVE_WITH_KNOTS ( 'NONE', 3,
 ( #93718, #1709, #153405, #152412, #16890, #46230, #170571, #15899, #183759, #154405, #77557, #78541, #199924, #704, #171568, #105909, #141217, #79548, #167595, #31068, #169571, #123059, #139229, #168572, #32062, #91711, #140216, #2708, #62376, #109884, #92716, #33057, #184745, #29090, #107884, #63385, #125062, #44252, #61387, #94712 ),
 .UNSPECIFIED., .F., .F.,
 ( 4, 2, 2, 2, 2, 2, 2, 2, 2, 2, 2, 2, 2, 2, 2, 2, 2, 2, 2, 4 ),
 ( 0.02146664961600481397, 0.02254346109514428556, 0.02362027257428375715, 0.02415867831385349468, 0.02469708405342323568, 0.02577389553256272461, 0.02685070701170221355, 0.02738911275127196149, 0.02792751849084170596, 0.02900432996998121224, 0.03008114144912071852, 0.03115795292826022828, 0.03223476440739973803, 0.03331157588653924778, 0.03438838736567875753, 0.03546519884481826035, 0.03600360458438801176, 0.03654201032395776316, 0.03761882180309726598, 0.03869563328223676879 ),
 .UNSPECIFIED. ) ;
#92235=CARTESIAN_POINT ( 'NONE',  ( 8.906447517083050158, 27.41122689804195645, 145.6500000054623740 ) ) ;
#92248=CARTESIAN_POINT ( 'NONE',  ( -37.99533089065118219, -0.2660902954431525469, -7.999999999999996447 ) ) ;
#92268=CARTESIAN_POINT ( 'NONE',  ( -36.79349492566039714, 4.147684444183149743, 48.62988885745599532 ) ) ;
#92274=CARTESIAN_POINT ( 'NONE',  ( 27.73933785331498569, 2.768321779492822058E-14, 147.8750000027311842 ) ) ;
#92301=EDGE_CURVE ( 'NONE', #129957, #68554, #106772, .T. ) ;
#92312=ORIENTED_EDGE ( 'NONE', *, *, #27194, .T. ) ;
#92368=CARTESIAN_POINT ( 'NONE',  ( -28.82186960331508985, -9.364793116373393289, 144.3500000054623627 ) ) ;
#92387=CARTESIAN_POINT ( 'NONE',  ( -3.573655867282028392E-15, 2.428612866367529932E-14, 2.000000000000000000 ) ) ;
#92439=CARTESIAN_POINT ( 'NONE',  ( 35.52763170759349265, 3.100152895725894808, 38.16632899394347334 ) ) ;
#92554=FACE_OUTER_BOUND ( 'NONE', #110893, .T. ) ;
#92628=CARTESIAN_POINT ( 'NONE',  ( 36.91746824999999177, 2.880721459617395097E-14, -3.624999997268813168 ) ) ;
#92716=CARTESIAN_POINT ( 'NONE',  ( -37.36625173109578668, -3.353228347065801973, 40.62582701645504102 ) ) ;
#92737=DIRECTION ( 'NONE',  ( 3.709348145883536076E-20, 0.000000000000000000, -1.000000000000000000 ) ) ;
#92747=CARTESIAN_POINT ( 'NONE',  ( -17.14385361876520619, 23.59649016807275856, 145.0750000027311728 ) ) ;
#92770=CARTESIAN_POINT ( 'NONE',  ( -17.81289503416611097, -24.51734667627696496, 140.2999999999999545 ) ) ;
#92771=CARTESIAN_POINT ( 'NONE',  ( -17.81289503416611808, 24.51734667627700404, 143.9500000054623854 ) ) ;
#92861=CARTESIAN_POINT ( 'NONE',  ( -22.44159573604009950, -16.30477369853688430, 141.0750000027311728 ) ) ;
#92889=EDGE_CURVE ( 'NONE', #191417, #60925, #110053, .T. ) ;
#92914=VECTOR ( 'NONE', #134855, 1000.000000000000000 ) ;
#92976=ORIENTED_EDGE ( 'NONE', *, *, #151903, .F. ) ;
#92987=CARTESIAN_POINT ( 'NONE',  ( 36.91746825000000598, -11.99521256947793546, -8.224999997268810148 ) ) ;
#92993=CARTESIAN_POINT ( 'NONE',  ( 33.81930014798969353, 1.942787237620516416, 100.1485738335251199 ) ) ;
#93005=CARTESIAN_POINT ( 'NONE',  ( 29.86685920354754842, -21.69954338932559068, -6.324999997268814234 ) ) ;
#93028=CARTESIAN_POINT ( 'NONE',  ( -31.60163464511078146, -3.334671618079672939, 101.7358725107059598 ) ) ;
#93092=CARTESIAN_POINT ( 'NONE',  ( -40.00200000000003087, -5.510910596163089556E-15, 37.50000000000000000 ) ) ;
#93099=FACE_OUTER_BOUND ( 'NONE', #140285, .T. ) ;
#93113=CARTESIAN_POINT ( 'NONE',  ( 35.99626262588764547, 2.869439944428138037E-14, 2.000000000000000000 ) ) ;
#93145=EDGE_CURVE ( 'NONE', #97386, #8281, #193801, .T. ) ;
#93177=CARTESIAN_POINT ( 'NONE',  ( -11.40812507854754720, -35.11059874428192273, -4.724999997268812812 ) ) ;
#93228=CARTESIAN_POINT ( 'NONE',  ( -5.429308488886486681E-15, 30.30510711980690175, 145.7500000054623115 ) ) ;
#93246=ORIENTED_EDGE ( 'NONE', *, *, #72314, .F. ) ;
#93260=CARTESIAN_POINT ( 'NONE',  ( -36.91128768240056246, 1.976579976310101802E-14, 50.50000000000002842 ) ) ;
#93265=CARTESIAN_POINT ( 'NONE',  ( 27.73933785331498925, -9.013057229001033122, 143.7750000027311614 ) ) ;
#93279=ORIENTED_EDGE ( 'NONE', *, *, #33197, .T. ) ;
#93300=EDGE_CURVE ( 'NONE', #71503, #189747, #38195, .T. ) ;
#93375=ORIENTED_EDGE ( 'NONE', *, *, #36793, .F. ) ;
#93380=CARTESIAN_POINT ( 'NONE',  ( 11.74264578624800315, -36.14014761921581709, -9.400000000000000355 ) ) ;
#93425=EDGE_CURVE ( 'NONE', #68071, #184655, #62290, .T. ) ;
#93431=CARTESIAN_POINT ( 'NONE',  ( 34.52932710190714261, 5.142084072295515895, 50.46524955901335829 ) ) ;
#93588=DIRECTION ( 'NONE',  ( -7.709882115452493155E-15, 0.000000000000000000, 1.000000000000000000 ) ) ;
#93627=CARTESIAN_POINT ( 'NONE',  ( -22.81625015709509441, -31.40387420917324590, -2.324999997268813789 ) ) ;
#93674=CARTESIAN_POINT ( 'NONE',  ( -38.00000000000001421, 12.34694845685046438, -1.849999994537626424 ) ) ;
#93718=CARTESIAN_POINT ( 'NONE',  ( -36.91128768240056246, 1.976579976310101802E-14, 50.50000000000002842 ) ) ;
#93749=CARTESIAN_POINT ( 'NONE',  ( -27.73933785331498925, 2.428612866367529932E-14, 145.3750000027311842 ) ) ;
#93773=CARTESIAN_POINT ( 'NONE',  ( -17.81289503416611097, -24.51734667627696496, 146.5500000054623229 ) ) ;
#93786=ORIENTED_EDGE ( 'NONE', *, *, #168639, .F. ) ;
#93809=EDGE_LOOP ( 'NONE', ( #57826, #149012 ) ) ;
#93835=CARTESIAN_POINT ( 'NONE',  ( -11.74149087413295511, 36.13659316521247433, -2.147842220587803830 ) ) ;
#93863=CARTESIAN_POINT ( 'NONE',  ( 17.14385361876520264, -23.59649016807270883, 145.5750000027311728 ) ) ;
#93879=CARTESIAN_POINT ( 'NONE',  ( 30.73962218707677252, 22.33364281372847060, -4.547842220587804185 ) ) ;
#93882=DIRECTION ( 'NONE',  ( -1.000000000000000000, 0.000000000000000000, 0.000000000000000000 ) ) ;
#93947=B_SPLINE_CURVE_WITH_KNOTS ( 'NONE', 3,
 ( #98182, #19392, #38548, #3216, #158879, #68874, #99200, #81041, #161885, #65875, #127549, #22380, #50727, #159886, #21375, #82016, #143712, #130533, #53712, #103217, #165892, #86042, #25401, #178068, #196251, #56720, #193233, #87043, #162884, #117379, #57720, #148728, #89036, #9217, #39535, #164899, #10216, #70884, #101193, #119390 ),
 .UNSPECIFIED., .F., .F.,
 ( 4, 2, 2, 2, 2, 2, 2, 2, 2, 2, 2, 2, 2, 2, 2, 2, 2, 2, 2, 4 ),
 ( 0.02158449572284441495, 0.02266158837400312348, 0.02373868102516183201, 0.02427722735074119495, 0.02481577367632055789, 0.02589286632747930458, 0.02696995897863805128, 0.02804705162979680144, 0.02912414428095554814, 0.02966269060653492495, 0.03020123693211429483, 0.03127832958327309010, 0.03235542223443187149, 0.03343251488559066675, 0.03450960753674945508, 0.03558670018790824341, 0.03612524651348764104, 0.03666379283906703174, 0.03774088549022580619, 0.03881797814138458758 ),
 .UNSPECIFIED. ) ;
#93979=DIRECTION ( 'NONE',  ( -0.000000000000000000, -0.000000000000000000, -1.000000000000000000 ) ) ;
#93986=CARTESIAN_POINT ( 'NONE',  ( -5.950531402560715689E-15, 38.81732327939063509, -7.624999997268814056 ) ) ;
#93989=CARTESIAN_POINT ( 'NONE',  ( 30.73962218707677607, -22.33364281372841376, -2.947842220587804096 ) ) ;
#93991=CARTESIAN_POINT ( 'NONE',  ( 33.67975787243658203, 4.948374891829404376, 97.42774497825463698 ) ) ;
#94012=DIRECTION ( 'NONE',  ( 1.000000000000000000, 0.000000000000000000, 0.000000000000000000 ) ) ;
#94037=CARTESIAN_POINT ( 'NONE',  ( 34.77754859679603072, -0.9869066695168891012, 52.45091671276828293 ) ) ;
#94042=CARTESIAN_POINT ( 'NONE',  ( -28.82186960331499037, 2.781578969918950771E-14, 139.9999999999999716 ) ) ;
#94064=DIRECTION ( 'NONE',  ( 0.000000000000000000, 0.000000000000000000, -1.000000000000000000 ) ) ;
#94111=CARTESIAN_POINT ( 'NONE',  ( -3.573655867282028392E-15, 2.428612866367529932E-14, 150.0000000000000000 ) ) ;
#94173=CARTESIAN_POINT ( 'NONE',  ( 36.91746824999999887, 11.99521256947799053, -6.024999997268811747 ) ) ;
#94224=CARTESIAN_POINT ( 'NONE',  ( 17.81289503416610742, 24.51734667627700404, 143.2999999999999829 ) ) ;
#94257=CARTESIAN_POINT ( 'NONE',  ( -36.91128768240056246, 0.3596143131121838366, 50.50000000000001421 ) ) ;
#94262=CARTESIAN_POINT ( 'NONE',  ( -27.73933785331498925, -9.013057229001049109, 140.9750000027311501 ) ) ;
#94375=CARTESIAN_POINT ( 'NONE',  ( 30.74264578624799782, 22.33583958711400541, -8.800000000000000711 ) ) ;
#94442=EDGE_CURVE ( 'NONE', #68071, #33122, #63847, .T. ) ;
#94483=ORIENTED_EDGE ( 'NONE', *, *, #51286, .T. ) ;
#94542=ORIENTED_EDGE ( 'NONE', *, *, #32687, .F. ) ;
#94588=CARTESIAN_POINT ( 'NONE',  ( 33.70754165857146489, -5.457863348371952306, 95.70317755519533875 ) ) ;
#94622=CARTESIAN_POINT ( 'NONE',  ( -11.40812507854754720, -35.11059874428192273, -2.224999997268813701 ) ) ;
#94712=CARTESIAN_POINT ( 'NONE',  ( -37.58407650405589351, 1.968340676919130544E-14, 39.49999999999996447 ) ) ;
#94742=CARTESIAN_POINT ( 'NONE',  ( 28.82186960331498327, 2.781578969918950771E-14, 149.0000000000000000 ) ) ;
#94766=CARTESIAN_POINT ( 'NONE',  ( 28.82186960331499392, -9.364793116373510529, 143.1500000054623740 ) ) ;
#94788=ORIENTED_EDGE ( 'NONE', *, *, #140094, .T. ) ;
#94792=VECTOR ( 'NONE', #37040, 1000.000000000000114 ) ;
#94812=ORIENTED_EDGE ( 'NONE', *, *, #15250, .F. ) ;
#94860=CARTESIAN_POINT ( 'NONE',  ( -17.14385361876520264, -23.59649016807271238, 143.1750000027311671 ) ) ;
#94863=ORIENTED_EDGE ( 'NONE', *, *, #162675, .F. ) ;
#94984=CARTESIAN_POINT ( 'NONE',  ( -22.81625015709510507, 31.40387420917330275, -2.924999997268813434 ) ) ;
#94985=CARTESIAN_POINT ( 'NONE',  ( -33.67975787243658203, 4.948374891829404376, 97.42774497825463698 ) ) ;
#94989=CARTESIAN_POINT ( 'NONE',  ( 34.52594549653173317, 2.428612888752089207E-14, 89.49999999999897682 ) ) ;
#95008=EDGE_LOOP ( 'NONE', ( #172912, #1511 ) ) ;
#95171=CARTESIAN_POINT ( 'NONE',  ( 29.86685920354754842, -21.69954338932559068, -4.324999997268814234 ) ) ;
#95173=EDGE_CURVE ( 'NONE', #8281, #60180, #130197, .T. ) ;
#95262=CARTESIAN_POINT ( 'NONE',  ( -5.359611314223446995E-15, 29.16686587814335496, 142.3750000027311557 ) ) ;
#95329=CARTESIAN_POINT ( 'NONE',  ( -35.99626262588765968, 2.428612866367529932E-14, -8.000000000000000000 ) ) ;
#95331=CARTESIAN_POINT ( 'NONE',  ( 17.14385361876520264, -23.59649016807270883, 146.0750000027311728 ) ) ;
#95352=CARTESIAN_POINT ( 'NONE',  ( -28.82186960331499037, 2.428612866367529932E-14, 144.2500000054623683 ) ) ;
#95494=CARTESIAN_POINT ( 'NONE',  ( 36.91746824999999177, 2.880721459617395097E-14, -5.624999997268813168 ) ) ;
#95539=CYLINDRICAL_SURFACE ( 'NONE', #112570, 37.99626262588765968 ) ;
#95601=CARTESIAN_POINT ( 'NONE',  ( -3.573655867282028392E-15, 2.428612866367529932E-14, 139.9999999999999716 ) ) ;
#95615=CARTESIAN_POINT ( 'NONE',  ( 36.91746825000000598, -11.99521256947793546, -1.724999997268813479 ) ) ;
#95705=CARTESIAN_POINT ( 'NONE',  ( 11.74149087413294268, 36.13659316521247433, -6.347842220587802231 ) ) ;
#95712=VECTOR ( 'NONE', #34109, 1000.000000000000000 ) ;
#95736=CARTESIAN_POINT ( 'NONE',  ( 17.81289503416610742, 24.51734667627700404, 149.2999999999999545 ) ) ;
#95743=( BOUNDED_CURVE ( )  B_SPLINE_CURVE ( 2, ( #90664, #25038, #180724, #163538, #89682 ),
 .UNSPECIFIED., .F., .F. ) 
 B_SPLINE_CURVE_WITH_KNOTS ( ( 3, 2, 3 ),
 ( 0.6000000000000000888, 0.6199999999999999956, 0.6253070713679935722 ),
 .UNSPECIFIED. ) 
 CURVE ( )  GEOMETRIC_REPRESENTATION_ITEM ( )  RATIONAL_B_SPLINE_CURVE ( ( 0.9999999999999997780, 0.9510565162951537532, 1.000000000000000000, 0.9870126719490075473, 0.9809178115826312494 ) ) 
 REPRESENTATION_ITEM ( '' )  );
#95760=CARTESIAN_POINT ( 'NONE',  ( -8.906447517083060816, 27.41122689804195645, 141.8500000054623911 ) ) ;
#95781=CARTESIAN_POINT ( 'NONE',  ( -28.82186960331499037, 2.428612866367529932E-14, 142.0000000000000000 ) ) ;
#95853=CARTESIAN_POINT ( 'NONE',  ( -8.571926809382601320, -26.38167802310801591, 141.2750000027311899 ) ) ;
#95931=DIRECTION ( 'NONE',  ( 0.000000000000000000, 0.000000000000000000, -1.000000000000000000 ) ) ;
#95978=CARTESIAN_POINT ( 'NONE',  ( -5.950531402560715689E-15, 38.81732327939063509, -9.124999997268815832 ) ) ;
#96030=CARTESIAN_POINT ( 'NONE',  ( 34.87614885797842845, -6.488895056989331778, 41.23117619273099876 ) ) ;
#96215=CARTESIAN_POINT ( 'NONE',  ( 11.33808637246520945, -35.21329618173263754, -8.000000000000000000 ) ) ;
#96250=CARTESIAN_POINT ( 'NONE',  ( -17.14385361876520264, -23.59649016807271593, 141.1750000027311671 ) ) ;
#96254=CARTESIAN_POINT ( 'NONE',  ( -31.99364916731038022, -1.163414459189985801E-14, 97.65000000000000568 ) ) ;
#96263=ORIENTED_EDGE ( 'NONE', *, *, #60352, .F. ) ;
#96321=CARTESIAN_POINT ( 'NONE',  ( -27.73933785331498925, -9.013057229001049109, 145.4750000027311785 ) ) ;
#96409=VERTEX_POINT ( 'NONE', #123273 ) ;
#96478=CARTESIAN_POINT ( 'NONE',  ( 29.86685920354754842, -21.69954338932559068, -3.824999997268813345 ) ) ;
#96527=DIRECTION ( 'NONE',  ( -0.000000000000000000, -0.000000000000000000, -1.000000000000000000 ) ) ;
#96561=DIRECTION ( 'NONE',  ( 1.000000000000000000, 0.000000000000000000, 0.000000000000000000 ) ) ;
#96565=CARTESIAN_POINT ( 'NONE',  ( 33.77897430376540200, -2.912663603757497999, 99.66889340242285300 ) ) ;
#96598=CARTESIAN_POINT ( 'NONE',  ( 36.91746824999999177, 2.880721459617395097E-14, -5.624999997268813168 ) ) ;
#96689=CARTESIAN_POINT ( 'NONE',  ( 31.23842136418743820, -7.314639034718686261, 96.67538241540152910 ) ) ;
#96718=CARTESIAN_POINT ( 'NONE',  ( 27.73933785331498925, -9.013057229001033122, 140.2750000027311330 ) ) ;
#96739=CARTESIAN_POINT ( 'NONE',  ( -28.82186960331499037, 2.428612866367529932E-14, 138.2500000054623683 ) ) ;
#96768=CARTESIAN_POINT ( 'NONE',  ( -28.82186960331499037, 2.428612866367529932E-14, 142.2500000054623683 ) ) ;
#96944=ORIENTED_EDGE ( 'NONE', *, *, #135116, .F. ) ;
#96957=CARTESIAN_POINT ( 'NONE',  ( -36.91746825000001309, 11.99521256947798342, -8.724999997268813701 ) ) ;
#97011=CARTESIAN_POINT ( 'NONE',  ( 34.40736802160862595, -7.501760008519349654, 45.46231226804130188 ) ) ;
#97146=DIRECTION ( 'NONE',  ( 0.000000000000000000, 0.000000000000000000, 1.000000000000000000 ) ) ;
#97229=CARTESIAN_POINT ( 'NONE',  ( -8.571926809382608425, 26.38167802310805854, 140.4750000027312069 ) ) ;
#97262=ORIENTED_EDGE ( 'NONE', *, *, #181788, .F. ) ;
#97301=CARTESIAN_POINT ( 'NONE',  ( 27.73933785331498925, -9.013057229001034898, 144.2750000027311899 ) ) ;
#97350=CYLINDRICAL_SURFACE ( 'NONE', #175621, 35.99626262588765258 ) ;
#97378=CARTESIAN_POINT ( 'NONE',  ( -30.74264578624800492, 22.33583958711400186, -3.949999994537626957 ) ) ;
#97386=VERTEX_POINT ( 'NONE', #33276 ) ;
#97417=CYLINDRICAL_SURFACE ( 'NONE', #21353, 28.82186960331498682 ) ;
#97428=CARTESIAN_POINT ( 'NONE',  ( 22.81625015709509441, 31.40387420917330275, -1.824999997268813567 ) ) ;
#97459=CARTESIAN_POINT ( 'NONE',  ( -22.81625015709509441, -31.40387420917324590, -4.324999997268813345 ) ) ;
#97473=CARTESIAN_POINT ( 'NONE',  ( 37.99626262588765258, 2.893932880411085066E-14, 2.000000000000000000 ) ) ;
#97477=VERTEX_POINT ( 'NONE', #154624 ) ;
#97546=DIRECTION ( 'NONE',  ( 0.000000000000000000, -1.000000000000000000, 0.000000000000000000 ) ) ;
#97578=CARTESIAN_POINT ( 'NONE',  ( 22.81625015709509441, 31.40387420917330275, -9.324999997268813345 ) ) ;
#97669=CARTESIAN_POINT ( 'NONE',  ( 31.24427474013727490, -7.030368782406881678, 97.62376346805382354 ) ) ;
#97700=CARTESIAN_POINT ( 'NONE',  ( -28.82186960331499392, 9.364793116373565596, 145.8999999999999773 ) ) ;
#97722=CARTESIAN_POINT ( 'NONE',  ( -28.82186960331499037, 2.428612866367529932E-14, 140.2500000054623683 ) ) ;
#97815=CARTESIAN_POINT ( 'NONE',  ( -37.99626262588766679, 2.428612866367529932E-14, -6.002157773949822861 ) ) ;
#97835=CARTESIAN_POINT ( 'NONE',  ( 37.06950394710834473, -4.940869137700747871, 42.55762898535583361 ) ) ;
#97869=DIRECTION ( 'NONE',  ( -1.000000000000000000, 0.000000000000000000, 0.000000000000000000 ) ) ;
#97875=CIRCLE ( 'NONE', #52723, 2.699999999999993960 ) ;
#97891=LINE ( 'NONE', #51421, #69212 ) ;
#97936=CARTESIAN_POINT ( 'NONE',  ( 29.86685920354754842, -21.69954338932559068, -7.824999997268813345 ) ) ;
#97937=CARTESIAN_POINT ( 'NONE',  ( -33.70206089117255743, 4.379927107397421082, 98.34612363080974262 ) ) ;
#98073=( BOUNDED_CURVE ( )  B_SPLINE_CURVE ( 2, ( #2707, #126052, #49219, #172562, #34048, #50220, #95705, #69356, #84509, #164388, #163379 ),
 .UNSPECIFIED., .F., .F. ) 
 B_SPLINE_CURVE_WITH_KNOTS ( ( 3, 2, 2, 2, 2, 3 ),
 ( 0.4000000000000000222, 0.4199999999999999845, 0.4400000000000000577, 0.4600000000000000755, 0.4800000000000000933, 0.5000000000000001110 ),
 .UNSPECIFIED. ) 
 CURVE ( )  GEOMETRIC_REPRESENTATION_ITEM ( )  RATIONAL_B_SPLINE_CURVE ( ( 1.000000000000000000, 0.9510565162951535312, 1.000000000000000000, 0.9510565162951535312, 1.000000000000000000, 0.9510565162951535312, 1.000000000000000000, 0.9510565162951535312, 1.000000000000000000, 0.9510565162951533091, 1.000000000000000222 ) ) 
 REPRESENTATION_ITEM ( '' )  );
#98102=AXIS2_PLACEMENT_3D ( 'NONE', #52351, #37182, #127191 ) ;
#98161=DIRECTION ( 'NONE',  ( 0.000000000000000000, 0.000000000000000000, 1.000000000000000000 ) ) ;
#98182=CARTESIAN_POINT ( 'NONE',  ( -33.85315667487628133, 2.014031266883448522E-14, 100.5000000000010232 ) ) ;
#98202=VERTEX_POINT ( 'NONE', #98402 ) ;
#98221=CARTESIAN_POINT ( 'NONE',  ( -22.44159573604009950, -16.30477369853688430, 147.5750000027312012 ) ) ;
#98226=CARTESIAN_POINT ( 'NONE',  ( -30.73962218707677962, -22.33364281372842441, -5.547842220587804185 ) ) ;
#98294=CARTESIAN_POINT ( 'NONE',  ( -27.73933785331498925, 2.428612866367529932E-14, 143.3750000027311842 ) ) ;
#98297=CARTESIAN_POINT ( 'NONE',  ( 28.82186960331498327, 2.781578969918950771E-14, 141.0000000000000000 ) ) ;
#98352=AXIS2_PLACEMENT_3D ( 'NONE', #145184, #193718, #191697 ) ;
#98377=FACE_OUTER_BOUND ( 'NONE', #163865, .T. ) ;
#98402=CARTESIAN_POINT ( 'NONE',  ( -27.73933785331498925, 2.428612866367529932E-14, 149.3750000027311842 ) ) ;
#98429=FACE_OUTER_BOUND ( 'NONE', #301, .T. ) ;
#98432=FACE_OUTER_BOUND ( 'NONE', #186903, .T. ) ;
#98449=UNCERTAINTY_MEASURE_WITH_UNIT (LENGTH_MEASURE( 1.000000000000000082E-05 ), #130067, 'distance_accuracy_value', 'NONE');
#98464=CARTESIAN_POINT ( 'NONE',  ( 22.81625015709509441, 31.40387420917330275, -1.324999997268813123 ) ) ;
#98549=FACE_OUTER_BOUND ( 'NONE', #189298, .T. ) ;
#98586=CARTESIAN_POINT ( 'NONE',  ( -22.81625015709510507, 31.40387420917330275, -8.924999997268814766 ) ) ;
#98649=ORIENTED_EDGE ( 'NONE', *, *, #8154, .T. ) ;
#98661=CARTESIAN_POINT ( 'NONE',  ( -32.00000000000000711, -1.163414459189985801E-14, 95.00000000000000000 ) ) ;
#98675=ADVANCED_FACE ( 'NONE', ( #116506 ), #178194, .F. ) ;
#98679=CARTESIAN_POINT ( 'NONE',  ( 31.27032343591156049, -7.501918430611449473, 95.46114142609056330 ) ) ;
#98698=ORIENTED_EDGE ( 'NONE', *, *, #5174, .T. ) ;
#98709=CARTESIAN_POINT ( 'NONE',  ( -17.81289503416611097, -24.51734667627696496, 142.2999999999999829 ) ) ;
#98732=CARTESIAN_POINT ( 'NONE',  ( -28.82186960331499392, -9.364793116373526516, 140.3500000054623627 ) ) ;
#98773=ORIENTED_EDGE ( 'NONE', *, *, #149591, .F. ) ;
#98831=AXIS2_PLACEMENT_3D ( 'NONE', #101428, #163119, #148958 ) ;
#98840=CARTESIAN_POINT ( 'NONE',  ( -34.78522506798723413, -4.592425496937305498E-15, 52.50000000000000000 ) ) ;
#98913=( BOUNDED_CURVE ( )  B_SPLINE_CURVE ( 2, ( #120361, #150726, #69880, #105203, #131549, #180087, #166890, #151711, #28390, #178069, #101194 ),
 .UNSPECIFIED., .F., .T. ) 
 B_SPLINE_CURVE_WITH_KNOTS ( ( 3, 2, 2, 2, 2, 3 ),
 ( 0.8000000000000000444, 0.8200000000000000622, 0.8399999999999999689, 0.8599999999999999867, 0.8800000000000000044, 0.9000000000000000222 ),
 .UNSPECIFIED. ) 
 CURVE ( )  GEOMETRIC_REPRESENTATION_ITEM ( )  RATIONAL_B_SPLINE_CURVE ( ( 1.000000000000000000, 0.9510565162951535312, 1.000000000000000000, 0.9510565162951535312, 1.000000000000000000, 0.9510565162951535312, 1.000000000000000000, 0.9510565162951535312, 1.000000000000000000, 0.9510565162951535312, 1.000000000000000000 ) ) 
 REPRESENTATION_ITEM ( '' )  );
#98946=CARTESIAN_POINT ( 'NONE',  ( 29.86685920354754842, -21.69954338932559068, -3.824999997268813345 ) ) ;
#99083=CYLINDRICAL_SURFACE ( 'NONE', #45439, 2.649999999999999467 ) ;
#99110=LINE ( 'NONE', #116289, #115061 ) ;
#99154=CARTESIAN_POINT ( 'NONE',  ( -3.573655867282028392E-15, 2.428612866367529932E-14, 139.9999999999999716 ) ) ;
#99179=FACE_OUTER_BOUND ( 'NONE', #46528, .T. ) ;
#99200=CARTESIAN_POINT ( 'NONE',  ( -33.80025371042792415, -2.440809870420988403, 99.93203653199840630 ) ) ;
#99233=VERTEX_POINT ( 'NONE', #93113 ) ;
#99238=CARTESIAN_POINT ( 'NONE',  ( 1.784210473542230573E-15, -29.16686587814331588, 143.8750000027311557 ) ) ;
#99242=DIRECTION ( 'NONE',  ( 0.000000000000000000, 0.000000000000000000, 1.000000000000000000 ) ) ;
#99262=CIRCLE ( 'NONE', #121796, 5.500000000001017852 ) ;
#99313=CARTESIAN_POINT ( 'NONE',  ( -27.73933785331498925, 9.013057229001088189, 145.2750000027311899 ) ) ;
#99354=DIRECTION ( 'NONE',  ( 0.000000000000000000, 1.000000000000000000, -1.224646799147353207E-16 ) ) ;
#99390=CARTESIAN_POINT ( 'NONE',  ( -23.48529157249600985, 32.32473071737754111, -4.049999994537626158 ) ) ;
#99422=EDGE_CURVE ( 'NONE', #180473, #175994, #154978, .T. ) ;
#99426=DIRECTION ( 'NONE',  ( 1.000000000000000000, -0.000000000000000000, -0.000000000000000000 ) ) ;
#99443=CARTESIAN_POINT ( 'NONE',  ( -5.950531402560715689E-15, 38.81732327939063509, -1.624999997268813612 ) ) ;
#99445=CARTESIAN_POINT ( 'NONE',  ( -34.77754859679605204, -0.9869066695169159686, 52.45091671276826872 ) ) ;
#99460=ADVANCED_FACE ( 'NONE', ( #107289 ), #1099, .F. ) ;
#99474=CARTESIAN_POINT ( 'NONE',  ( -29.86685920354755552, 21.69954338932564397, -4.824999997268814234 ) ) ;
#99597=CARTESIAN_POINT ( 'NONE',  ( 29.86685920354754487, 21.69954338932564752, -7.424999997268813878 ) ) ;
#99694=ORIENTED_EDGE ( 'NONE', *, *, #112389, .T. ) ;
#99716=CARTESIAN_POINT ( 'NONE',  ( 23.31738231874054534, 16.94106989632529192, 141.1999999999999886 ) ) ;
#99739=CARTESIAN_POINT ( 'NONE',  ( 22.44159573604009239, 16.30477369853692693, 144.0750000027311728 ) ) ;
#99937=ORIENTED_EDGE ( 'NONE', *, *, #72705, .T. ) ;
#100008=ORIENTED_EDGE ( 'NONE', *, *, #130121, .T. ) ;
#100026=DIRECTION ( 'NONE',  ( -0.000000000000000000, -1.000000000000000000, 0.000000000000000000 ) ) ;
#100200=LINE ( 'NONE', #67868, #86839 ) ;
#100242=CARTESIAN_POINT ( 'NONE',  ( -17.14385361876520619, 23.59649016807275856, 141.0750000027311728 ) ) ;
#100276=DIRECTION ( 'NONE',  ( -1.000000000000000000, 0.000000000000000000, 0.000000000000000000 ) ) ;
#100315=DIRECTION ( 'NONE',  ( 0.000000000000000000, 0.000000000000000000, 1.000000000000000000 ) ) ;
#100395=CARTESIAN_POINT ( 'NONE',  ( -38.00000000000001421, -12.34694845685042708, -3.649999994537627135 ) ) ;
#100430=CARTESIAN_POINT ( 'NONE',  ( 31.28760401664903412, 6.510460035718195648, 98.73157056914057250 ) ) ;
#100444=CARTESIAN_POINT ( 'NONE',  ( 37.32565804592077541, 3.633088190964871789, 40.85532123380855296 ) ) ;
#100445=DIRECTION ( 'NONE',  ( 0.000000000000000000, 0.000000000000000000, -1.000000000000000000 ) ) ;
#100476=CARTESIAN_POINT ( 'NONE',  ( -37.07039049082557369, 4.937524616431669067, 42.55055737136175509 ) ) ;
#100495=ORIENTED_EDGE ( 'NONE', *, *, #190781, .T. ) ;
#100520=ORIENTED_EDGE ( 'NONE', *, *, #40971, .T. ) ;
#100526=CARTESIAN_POINT ( 'NONE',  ( 28.82186960331498327, 2.781578969918950771E-14, 143.0000000000000000 ) ) ;
#100570=CARTESIAN_POINT ( 'NONE',  ( -67.00000000000000000, -1.163414459189985801E-14, 89.49999999999897682 ) ) ;
#100595=CARTESIAN_POINT ( 'NONE',  ( -5.950531402560715689E-15, 38.81732327939063509, -9.124999997268815832 ) ) ;
#100674=CARTESIAN_POINT ( 'NONE',  ( -37.99626262588766679, 2.428612866367529932E-14, 2.000000000000000000 ) ) ;
#100690=ORIENTED_EDGE ( 'NONE', *, *, #79968, .F. ) ;
#100706=FACE_OUTER_BOUND ( 'NONE', #111424, .T. ) ;
#100746=( NAMED_UNIT ( * ) SI_UNIT ( $, .STERADIAN. ) SOLID_ANGLE_UNIT ( ) );
#100841=CARTESIAN_POINT ( 'NONE',  ( -28.82186960331504721, -9.364793116373462567, 148.0999999999999943 ) ) ;
#100916=CARTESIAN_POINT ( 'NONE',  ( -21.90810111552704242, 30.97181472859550411, -7.999999999999996447 ) ) ;
#100931=ORIENTED_EDGE ( 'NONE', *, *, #69397, .F. ) ;
#100947=CARTESIAN_POINT ( 'NONE',  ( -27.73933785331498925, -9.013057229001049109, 147.4750000027311785 ) ) ;
#100971=CARTESIAN_POINT ( 'NONE',  ( -34.87691056670620071, 6.486286472422003513, 41.22672555304435349 ) ) ;
#100974=EDGE_CURVE ( 'NONE', #60986, #113568, #119498, .T. ) ;
#101047=( BOUNDED_CURVE ( )  B_SPLINE_CURVE ( 2, ( #79218, #3369, #64057, #33715, #157062, #18559, #72031, #134719, #56874, #26544, #146871 ),
 .UNSPECIFIED., .F., .F. ) 
 B_SPLINE_CURVE_WITH_KNOTS ( ( 3, 2, 2, 2, 2, 3 ),
 ( 0.2000000000000001776, 0.2200000000000001954, 0.2400000000000002132, 0.2600000000000002309, 0.2800000000000003042, 0.3000000000000002665 ),
 .UNSPECIFIED. ) 
 CURVE ( )  GEOMETRIC_REPRESENTATION_ITEM ( )  RATIONAL_B_SPLINE_CURVE ( ( 0.9999999999999995559, 0.9510565162951539753, 1.000000000000000000, 0.9510565162951535312, 1.000000000000000000, 0.9510565162951535312, 1.000000000000000000, 0.9510565162951535312, 1.000000000000000000, 0.9510565162951528650, 1.000000000000000666 ) ) 
 REPRESENTATION_ITEM ( '' )  );
#101148=CARTESIAN_POINT ( 'NONE',  ( 33.65002604405838582, -15.23243535768875923, -8.000000000000003553 ) ) ;
#101193=CARTESIAN_POINT ( 'NONE',  ( -34.52594549653174028, -0.3594300054053902183, 89.49999999999896261 ) ) ;
#101194=CARTESIAN_POINT ( 'NONE',  ( 37.99626262588765258, 2.893932880411085066E-14, -1.002157773949823083 ) ) ;
#101234=CARTESIAN_POINT ( 'NONE',  ( 22.44159573604009594, -16.30477369853687364, 146.1750000027311671 ) ) ;
#101310=CARTESIAN_POINT ( 'NONE',  ( 1.784210473542230573E-15, -29.16686587814331588, 139.8750000027312126 ) ) ;
#101320=CARTESIAN_POINT ( 'NONE',  ( -67.00000000000000000, -5.510910596163089556E-15, 45.00000000000000000 ) ) ;
#101330=FACE_OUTER_BOUND ( 'NONE', #106686, .T. ) ;
#101362=VECTOR ( 'NONE', #52075, 1000.000000000000000 ) ;
#101384=CARTESIAN_POINT ( 'NONE',  ( -30.74264578624800492, 22.33583958711400186, -7.949999994537626513 ) ) ;
#101422=CARTESIAN_POINT ( 'NONE',  ( 31.23718726401124712, 7.254977440570237412, 96.91727682732810933 ) ) ;
#101428=CARTESIAN_POINT ( 'NONE',  ( 31.99364916730971231, 1.011436372600181938E-12, 95.00000000000021316 ) ) ;
#101436=CARTESIAN_POINT ( 'NONE',  ( 36.86581981986046230, 2.436233122106823412, 49.93429970834161935 ) ) ;
#101439=CARTESIAN_POINT ( 'NONE',  ( -34.51183469268316628, -7.447092774749549449, 43.98515247788456861 ) ) ;
#101468=B_SPLINE_CURVE_WITH_KNOTS ( 'NONE', 3,
 ( #191035, #20181, #128347, #174873, #157717, #52509, #188066, #80856, #67682, #65689, #48554, #172891, #34370, #51521, #96030, #19206, #189067, #111199, #64707, #142532, #143514, #97011, #127354, #170890, #4011, #159685, #63712, #110207, #35359, #79873, #2032, #113183, #50539, #125387, #36338, #32382, #18216, #144517, #158692, #3031, #94037, #81827, #155715 ),
 .UNSPECIFIED., .F., .F.,
 ( 4, 2, 2, 2, 2, 2, 2, 2, 2, 2, 2, 2, 2, 1, 2, 2, 2, 2, 2, 2, 2, 4 ),
 ( 0.04122229388621100749, 0.04269295678691726464, 0.04416361968762351486, 0.04489895113797664344, 0.04563428258832977202, 0.04710494548903602224, 0.04857560838974227940, 0.04931093984009540798, 0.05004627129044854350, 0.05151693419115481454, 0.05298759709186107864, 0.05445825999256734967, 0.05519359144292047825, 0.05592892289327359989, 0.05666425434362672153, 0.05739958579397984317, 0.05887024869468611421, 0.06034091159539237831, 0.06181157449609863547, 0.06254690594645176405, 0.06328223739680489957, 0.06475290029751117060 ),
 .UNSPECIFIED. ) ;
#101484=EDGE_LOOP ( 'NONE', ( #35122, #73624, #99694, #176507 ) ) ;
#101537=AXIS2_PLACEMENT_3D ( 'NONE', #98661, #160355, #1692 ) ;
#101569=CIRCLE ( 'NONE', #53065, 2.649999999999999467 ) ;
#101599=CARTESIAN_POINT ( 'NONE',  ( -38.00000000000000711, 2.428612866367529932E-14, -6.000000000000000000 ) ) ;
#101712=DIRECTION ( 'NONE',  ( 0.000000000000000000, 0.000000000000000000, 1.000000000000000000 ) ) ;
#101721=CARTESIAN_POINT ( 'NONE',  ( -17.81289503416611097, -24.51734667627696496, 144.2999999999999829 ) ) ;
#101756=DIRECTION ( 'NONE',  ( 0.000000000000000000, 0.000000000000000000, 1.000000000000000000 ) ) ;
#101781=ORIENTED_EDGE ( 'NONE', *, *, #59844, .T. ) ;
#101932=CARTESIAN_POINT ( 'NONE',  ( -28.82186960331499037, 2.781578969918950771E-14, 139.9999999999999716 ) ) ;
#101935=LINE ( 'NONE', #164618, #160660 ) ;
#101970=DIRECTION ( 'NONE',  ( -6.982962677686266711E-15, 0.000000000000000000, 1.000000000000000000 ) ) ;
#102084=DIRECTION ( 'NONE',  ( 0.000000000000000000, 0.000000000000000000, -1.000000000000000000 ) ) ;
#102215=CARTESIAN_POINT ( 'NONE',  ( 40.00000000000001421, 2.428612866367529932E-14, 0.000000000000000000 ) ) ;
#102218=CARTESIAN_POINT ( 'NONE',  ( -33.63107349886310971, -17.13970281212090185, -7.999999999999998224 ) ) ;
#102230=CARTESIAN_POINT ( 'NONE',  ( 29.86685920354754842, -21.69954338932559068, -2.324999997268813345 ) ) ;
#102252=CARTESIAN_POINT ( 'NONE',  ( -31.24427474013728201, -7.030368782406874573, 97.62376346805388039 ) ) ;
#102257=CARTESIAN_POINT ( 'NONE',  ( 8.571926809382603096, -26.38167802310801235, 143.9750000027312069 ) ) ;
#102262=CARTESIAN_POINT ( 'NONE',  ( 30.00000000000000711, -1.163414459189985801E-14, 87.50000000000000000 ) ) ;
#102269=ORIENTED_EDGE ( 'NONE', *, *, #157283, .T. ) ;
#102328=CARTESIAN_POINT ( 'NONE',  ( 1.784210473542230573E-15, -29.16686587814331588, 147.3750000027311842 ) ) ;
#102403=CARTESIAN_POINT ( 'NONE',  ( 23.48529157249599919, 32.32473071737754111, -8.449999994537625625 ) ) ;
#102439=CARTESIAN_POINT ( 'NONE',  ( 32.64453336272027428, 0.4913919212617400833, 87.49999999999998579 ) ) ;
#102446=CARTESIAN_POINT ( 'NONE',  ( 31.51098639601625351, -4.378554692192639486, 101.0941514966582986 ) ) ;
#102456=CARTESIAN_POINT ( 'NONE',  ( -34.37176626784630429, -7.314009959508100955, 46.67821535514400466 ) ) ;
#102523=AXIS2_PLACEMENT_3D ( 'NONE', #123062, #78544, #77560 ) ;
#102567=LINE ( 'NONE', #19984, #20250 ) ;
#102598=DIRECTION ( 'NONE',  ( 1.000000000000000000, 0.000000000000000000, 0.000000000000000000 ) ) ;
#102613=CARTESIAN_POINT ( 'NONE',  ( -38.00000000000001421, -12.34694845685042708, -3.899999999999999911 ) ) ;
#102700=CARTESIAN_POINT ( 'NONE',  ( -37.99626262588766679, 2.428612866367529932E-14, -3.747842220587803475 ) ) ;
#102728=CARTESIAN_POINT ( 'NONE',  ( -8.906447517083060816, 27.41122689804195645, 141.5999999999999943 ) ) ;
#102737=ADVANCED_FACE ( 'NONE', ( #102993 ), #134346, .T. ) ;
#102859=CARTESIAN_POINT ( 'NONE',  ( 37.58407650405590061, -0.3597885541503427764, 39.49999999999997868 ) ) ;
#102916=CARTESIAN_POINT ( 'NONE',  ( -8.906447517083060816, 27.41122689804195645, 145.5999999999999943 ) ) ;
#102930=CARTESIAN_POINT ( 'NONE',  ( 15.17009418914603280, 34.12532338773831242, -7.999999999999996447 ) ) ;
#102966=FACE_OUTER_BOUND ( 'NONE', #140921, .T. ) ;
#102983=CARTESIAN_POINT ( 'NONE',  ( -34.80630918731043977, 6.717782050307405939, 41.65621224074541828 ) ) ;
#102993=FACE_OUTER_BOUND ( 'NONE', #160392, .T. ) ;
#103040=CARTESIAN_POINT ( 'NONE',  ( 30.00000000000000000, -1.163414459189985801E-14, 95.00000000000000000 ) ) ;
#103180=ORIENTED_EDGE ( 'NONE', *, *, #199664, .T. ) ;
#103195=VECTOR ( 'NONE', #49671, 1000.000000000000000 ) ;
#103211=CARTESIAN_POINT ( 'NONE',  ( -36.91746825000001309, -11.99521256947794789, -3.024999997268812635 ) ) ;
#103217=CARTESIAN_POINT ( 'NONE',  ( -33.72427247603956602, -5.492275790717718209, 95.34298344322783691 ) ) ;
#103257=CARTESIAN_POINT ( 'NONE',  ( 17.14385361876520264, 23.59649016807275856, 144.6750000027311671 ) ) ;
#103270=ORIENTED_EDGE ( 'NONE', *, *, #54728, .F. ) ;
#103290=CARTESIAN_POINT ( 'NONE',  ( 17.81289503416610742, 24.51734667627700404, 139.5500000054623229 ) ) ;
#103342=ADVANCED_FACE ( 'NONE', ( #98429 ), #186113, .T. ) ;
#103404=CARTESIAN_POINT ( 'NONE',  ( 30.74264578624800137, -22.33583958711395212, -10.94999999453762562 ) ) ;
#103443=CARTESIAN_POINT ( 'NONE',  ( 32.63002904509641411, 0.9908434387721892778, 87.54952558906809656 ) ) ;
#103457=CARTESIAN_POINT ( 'NONE',  ( 36.91128768240057667, 0.3596143131121917191, 50.50000000000004263 ) ) ;
#103460=DIRECTION ( 'NONE',  ( 0.000000000000000000, 0.000000000000000000, -1.000000000000000000 ) ) ;
#103489=CARTESIAN_POINT ( 'NONE',  ( -37.47229216401453300, 2.437641287457621875, 40.05669362136318767 ) ) ;
#103501=CARTESIAN_POINT ( 'NONE',  ( -27.73933785331498925, 9.013057229001089965, 142.7750000027311899 ) ) ;
#103574=CARTESIAN_POINT ( 'NONE',  ( -32.42786921226274899, 3.325810949901248037, 88.27324663263314619 ) ) ;
#103575=CARTESIAN_POINT ( 'NONE',  ( 28.82186960331498327, 2.781578969918950771E-14, 147.0000000000000000 ) ) ;
#103616=CARTESIAN_POINT ( 'NONE',  ( 38.00000000000000711, -12.34694845685040754, -5.099999999999999645 ) ) ;
#103711=VERTEX_POINT ( 'NONE', #195997 ) ;
#103724=CARTESIAN_POINT ( 'NONE',  ( 31.99999999999934275, 1.011436372600181938E-12, 95.00000000000021316 ) ) ;
#103734=CARTESIAN_POINT ( 'NONE',  ( -17.81289503416611808, 24.51734667627700404, 143.9500000054623854 ) ) ;
#103745=ADVANCED_FACE ( 'NONE', ( #23129 ), #150926, .F. ) ;
#103931=CARTESIAN_POINT ( 'NONE',  ( 22.33498979914476479, 29.77355716069116198, -8.000000000000000000 ) ) ;
#103934=CARTESIAN_POINT ( 'NONE',  ( -8.906447517083053711, -27.41122689804191026, 140.6500000054623740 ) ) ;
#103944=EDGE_CURVE ( 'NONE', #170159, #187938, #14259, .T. ) ;
#103985=CARTESIAN_POINT ( 'NONE',  ( -34.36946425582528519, 7.112708652184207558, 47.39170078794325747 ) ) ;
#104029=ORIENTED_EDGE ( 'NONE', *, *, #176156, .T. ) ;
#104094=CARTESIAN_POINT ( 'NONE',  ( -37.99626262588766679, 2.428612866367529932E-14, -3.747842220587803475 ) ) ;
#104165=DIRECTION ( 'NONE',  ( -1.000000000000000000, -0.000000000000000000, -0.000000000000000000 ) ) ;
#104205=CARTESIAN_POINT ( 'NONE',  ( -36.91746825000001309, 11.99521256947798342, -3.224999997268813257 ) ) ;
#104222=CARTESIAN_POINT ( 'NONE',  ( -37.99626262588766679, 2.428612866367529932E-14, 2.000000000000000000 ) ) ;
#104224=CARTESIAN_POINT ( 'NONE',  ( 22.81625015709509441, 31.40387420917330275, -1.824999997268813345 ) ) ;
#104245=CARTESIAN_POINT ( 'NONE',  ( -31.54463713289767313, -7.108708273820908197, 92.55936662351709288 ) ) ;
#104255=SURFACE_STYLE_USAGE ( .BOTH. , #27437 ) ;
#104263=ORIENTED_EDGE ( 'NONE', *, *, #141788, .T. ) ;
#104282=CARTESIAN_POINT ( 'NONE',  ( 28.82186960331521419, 9.364793116373263615, 139.3500000054624195 ) ) ;
#104283=EDGE_CURVE ( 'NONE', #55000, #60925, #26905, .T. ) ;
#104397=CARTESIAN_POINT ( 'NONE',  ( -38.00000000000001421, -12.34694845685042708, -11.64999999453762669 ) ) ;
#104450=CARTESIAN_POINT ( 'NONE',  ( 36.78335851983071336, 5.362873614019889601, 46.23361200806721882 ) ) ;
#104482=CARTESIAN_POINT ( 'NONE',  ( -36.80083376053583066, 5.466397602639213815, 45.70522705241149453 ) ) ;
#104489=CARTESIAN_POINT ( 'NONE',  ( 8.571926809382597767, 26.38167802310806209, 148.2750000027311899 ) ) ;
#104495=CARTESIAN_POINT ( 'NONE',  ( -27.73933785331498925, -9.013057229001049109, 142.9750000027312069 ) ) ;
#104603=CARTESIAN_POINT ( 'NONE',  ( -11.74264578624799782, -36.14014761921581709, -5.599999999999999645 ) ) ;
#104655=CARTESIAN_POINT ( 'NONE',  ( 34.67272174748971736, 7.108278434163713300, 42.55803597338272226 ) ) ;
#104758=VECTOR ( 'NONE', #57790, 1000.000000000000000 ) ;
#104796=VECTOR ( 'NONE', #59517, 1000.000000000000000 ) ;
#104804=CYLINDRICAL_SURFACE ( 'NONE', #133924, 5.500000000000032863 ) ;
#104954=CARTESIAN_POINT ( 'NONE',  ( 22.44159573604009594, -16.30477369853687364, 142.1750000027311671 ) ) ;
#105196=CARTESIAN_POINT ( 'NONE',  ( -36.91746825000000598, 2.428612866367529932E-14, -11.12499999726881228 ) ) ;
#105203=CARTESIAN_POINT ( 'NONE',  ( -23.48298174826589602, -32.32155151706772500, -1.702157773949823039 ) ) ;
#105247=SHAPE_REPRESENTATION_RELATIONSHIP ( 'NONE' , 'NONE' ,  #31381, #35157 ) ;
#105254=ORIENTED_EDGE ( 'NONE', *, *, #113740, .T. ) ;
#105308=CARTESIAN_POINT ( 'NONE',  ( -36.91746825000000598, 2.428612866367529932E-14, -0.6249999972688132788 ) ) ;
#105310=EDGE_CURVE ( 'NONE', #98202, #180473, #86366, .T. ) ;
#105313=CARTESIAN_POINT ( 'NONE',  ( 31.79999999999970939, 4.794320942884876164E-13, 42.30000000000021743 ) ) ;
#105382=CARTESIAN_POINT ( 'NONE',  ( -36.91746825000001309, 11.99521256947798342, -3.224999997268813257 ) ) ;
#105395=LINE ( 'NONE', #25600, #40457 ) ;
#105430=CARTESIAN_POINT ( 'NONE',  ( 31.64627301717022689, -2.653341670344218084, 102.0192792579183418 ) ) ;
#105474=CARTESIAN_POINT ( 'NONE',  ( 17.14385361876520264, 23.59649016807275856, 146.1750000027311387 ) ) ;
#105479=CARTESIAN_POINT ( 'NONE',  ( 22.44159573604009594, -16.30477369853687364, 145.6750000027311671 ) ) ;
#105547=CIRCLE ( 'NONE', #18382, 2.649999999999999467 ) ;
#105587=CARTESIAN_POINT ( 'NONE',  ( 38.00000000000000000, 12.34694845685046616, -6.899999999999999467 ) ) ;
#105639=CARTESIAN_POINT ( 'NONE',  ( 34.77757469352545172, 0.9858555240219483151, 52.45108825929359142 ) ) ;
#105658=AXIS2_PLACEMENT_3D ( 'NONE', #63616, #20086, #124282 ) ;
#105710=CARTESIAN_POINT ( 'NONE',  ( -36.91746825000000598, 11.99521256947798520, -0.7249999972688133676 ) ) ;
#105895=FACE_OUTER_BOUND ( 'NONE', #122257, .T. ) ;
#105909=CARTESIAN_POINT ( 'NONE',  ( -36.76911729423384401, -4.939512937650264668, 47.42567687524350362 ) ) ;
#105930=CARTESIAN_POINT ( 'NONE',  ( 28.82186960331498327, 2.428612866367529932E-14, 139.9999999999999716 ) ) ;
#105940=CARTESIAN_POINT ( 'NONE',  ( 22.44159573604009239, 16.30477369853692693, 144.5750000027311728 ) ) ;
#105965=CARTESIAN_POINT ( 'NONE',  ( 23.31738231874054890, -16.94106989632523508, 147.0500000054623797 ) ) ;
#106051=CARTESIAN_POINT ( 'NONE',  ( -27.73933785331498925, -9.013057229001049109, 139.4750000027311785 ) ) ;
#106148=ORIENTED_EDGE ( 'NONE', *, *, #3703, .F. ) ;
#106179=CARTESIAN_POINT ( 'NONE',  ( 29.86685920354754842, -21.69954338932559068, -1.824999997268813345 ) ) ;
#106185=CARTESIAN_POINT ( 'NONE',  ( 33.74157273865942130, 3.640299887980672722, 99.13851753912355491 ) ) ;
#106197=CARTESIAN_POINT ( 'NONE',  ( 29.86685920354754842, -21.69954338932559068, -4.324999997268814234 ) ) ;
#106205=ORIENTED_EDGE ( 'NONE', *, *, #92889, .F. ) ;
#106229=( NAMED_UNIT ( * ) PLANE_ANGLE_UNIT ( ) SI_UNIT ( $, .RADIAN. ) );
#106236=EDGE_CURVE ( 'NONE', #58436, #50775, #115755, .T. ) ;
#106290=ORIENTED_EDGE ( 'NONE', *, *, #124857, .T. ) ;
#106329=DIRECTION ( 'NONE',  ( 0.000000000000000000, 0.000000000000000000, -1.000000000000000000 ) ) ;
#106366=CARTESIAN_POINT ( 'NONE',  ( -29.86685920354755552, 21.69954338932564397, -3.324999997268813345 ) ) ;
#106456=CARTESIAN_POINT ( 'NONE',  ( 27.73933785331498214, 9.013057229001095294, 147.9750000027311501 ) ) ;
#106461=CARTESIAN_POINT ( 'NONE',  ( 27.73933785331498569, 2.768321779492822058E-14, 143.8750000027311842 ) ) ;
#106576=DIRECTION ( 'NONE',  ( 0.000000000000000000, -0.000000000000000000, 1.000000000000000000 ) ) ;
#106628=CARTESIAN_POINT ( 'NONE',  ( 35.24576003106573552, 4.949822944371136124, 39.34410620168028316 ) ) ;
#106675=EDGE_LOOP ( 'NONE', ( #77464, #58154, #111412, #73707, #44984, #89476, #94542, #7392, #12942, #192992, #58333 ) ) ;
#106686=EDGE_LOOP ( 'NONE', ( #157166, #195820, #7416, #46421 ) ) ;
#106697=CARTESIAN_POINT ( 'NONE',  ( -17.81289503416611808, 24.51734667627700404, 147.9500000054623854 ) ) ;
#106772=CIRCLE ( 'NONE', #19594, 37.99626262588765968 ) ;
#106817=CARTESIAN_POINT ( 'NONE',  ( 22.81625015709510151, -31.40387420917324590, -1.924999997268813434 ) ) ;
#106856=VERTEX_POINT ( 'NONE', #145725 ) ;
#106928=CARTESIAN_POINT ( 'NONE',  ( -17.14385361876520619, 23.59649016807275856, 147.0750000027311728 ) ) ;
#106951=CARTESIAN_POINT ( 'NONE',  ( 28.82186960331498327, 9.364793116373570925, 147.3500000054623627 ) ) ;
#106972=CARTESIAN_POINT ( 'NONE',  ( 37.99626262588765258, 2.893932880411085066E-14, -6.747842220587804363 ) ) ;
#107039=CARTESIAN_POINT ( 'NONE',  ( -27.73933785331498925, 9.013057229001088189, 148.7750000027311899 ) ) ;
#107132=ORIENTED_EDGE ( 'NONE', *, *, #112783, .T. ) ;
#107164=CARTESIAN_POINT ( 'NONE',  ( 36.91746824999999177, 2.880721459617395097E-14, -10.12499999726881583 ) ) ;
#107222=ORIENTED_EDGE ( 'NONE', *, *, #124857, .F. ) ;
#107267=CARTESIAN_POINT ( 'NONE',  ( -31.65987002919144899, 2.420393710425506661, 102.1029948765363997 ) ) ;
#107274=DIRECTION ( 'NONE',  ( 1.000000000000000000, 0.000000000000000000, 0.000000000000000000 ) ) ;
#107278=DIRECTION ( 'NONE',  ( 0.000000000000000000, 0.000000000000000000, -1.000000000000000000 ) ) ;
#107289=FACE_OUTER_BOUND ( 'NONE', #193819, .T. ) ;
#107306=DIRECTION ( 'NONE',  ( 0.000000000000000000, 0.000000000000000000, -1.000000000000000000 ) ) ;
#107350=CARTESIAN_POINT ( 'NONE',  ( -29.86685920354755197, -21.69954338932560134, -4.924999997268813878 ) ) ;
#107361=EDGE_LOOP ( 'NONE', ( #89491, #93279, #199405, #19440 ) ) ;
#107404=CARTESIAN_POINT ( 'NONE',  ( -17.81289503416611808, 24.51734667627700404, 145.9500000054623854 ) ) ;
#107416=CARTESIAN_POINT ( 'NONE',  ( -23.48298174826589602, -32.32155151706772500, -7.702157773949822150 ) ) ;
#107436=CARTESIAN_POINT ( 'NONE',  ( -36.89613260305527831, 1.429147721188399389, 50.32345767270690118 ) ) ;
#107442=CARTESIAN_POINT ( 'NONE',  ( -8.571926809382608425, 26.38167802310805854, 144.4750000027312069 ) ) ;
#107477=ORIENTED_EDGE ( 'NONE', *, *, #111650, .F. ) ;
#107517=CARTESIAN_POINT ( 'NONE',  ( 22.44159573604009239, 16.30477369853692693, 148.5750000027312012 ) ) ;
#107540=CYLINDRICAL_SURFACE ( 'NONE', #35607, 7.500000000000007105 ) ;
#107555=CARTESIAN_POINT ( 'NONE',  ( 37.99999999999999289, 2.893978650043524126E-14, -9.000000000000001776 ) ) ;
#107607=CARTESIAN_POINT ( 'NONE',  ( 35.41256452865196991, 3.967314244253455691, 38.63057146076393877 ) ) ;
#107796=CARTESIAN_POINT ( 'NONE',  ( -22.81625015709510507, 31.40387420917330275, -0.9249999972688132122 ) ) ;
#107880=CONICAL_SURFACE ( 'NONE', #14676, 40.00000000000002132, 0.06108652381980166773 ) ;
#107884=CARTESIAN_POINT ( 'NONE',  ( -37.48574882824303955, -2.272739345372926767, 39.98829423970373398 ) ) ;
#107916=CARTESIAN_POINT ( 'NONE',  ( 22.44159573604009239, 16.30477369853692693, 146.5750000027312012 ) ) ;
#107940=CARTESIAN_POINT ( 'NONE',  ( -5.429308488886486681E-15, 30.30510711980690175, 147.7500000054623683 ) ) ;
#107954=ORIENTED_EDGE ( 'NONE', *, *, #13961, .F. ) ;
#108031=CARTESIAN_POINT ( 'NONE',  ( -8.571926809382601320, -26.38167802310801591, 143.2750000027311899 ) ) ;
#108047=CARTESIAN_POINT ( 'NONE',  ( 11.74149087413294268, 36.13659316521247433, -4.347842220587804007 ) ) ;
#108160=CARTESIAN_POINT ( 'NONE',  ( -36.91746825000000598, 2.428612866367529932E-14, -0.6249999972688132788 ) ) ;
#108166=CARTESIAN_POINT ( 'NONE',  ( 34.51819068884489639, 0.7175229865516599137, 89.53493623002428592 ) ) ;
#108179=CARTESIAN_POINT ( 'NONE',  ( 22.81625015709509441, 31.40387420917330275, -5.824999997268813345 ) ) ;
#108264=ADVANCED_FACE ( 'NONE', ( #180431, #116730 ), #40894, .F. ) ;
#108268=CARTESIAN_POINT ( 'NONE',  ( -32.63002904509643542, 0.9908434387722265813, 87.54952558906812499 ) ) ;
#108269=AXIS2_PLACEMENT_3D ( 'NONE', #199644, #45952, #182497 ) ;
#108327=TOROIDAL_SURFACE ( 'NONE', #195096, 2.700000000000000622, 0.2000000000000000111 ) ;
#108355=CARTESIAN_POINT ( 'NONE',  ( -11.40812507854755609, 35.11059874428196537, -9.524999997268816188 ) ) ;
#108375=VERTEX_POINT ( 'NONE', #178419 ) ;
#108419=CIRCLE ( 'NONE', #114913, 2.649999999999999467 ) ;
#108445=CARTESIAN_POINT ( 'NONE',  ( -27.73933785331498925, 9.013057229001089965, 144.7750000027311614 ) ) ;
#108481=VERTEX_POINT ( 'NONE', #147075 ) ;
#108503=EDGE_CURVE ( 'NONE', #150593, #60986, #102567, .T. ) ;
#108595=ORIENTED_EDGE ( 'NONE', *, *, #13466, .F. ) ;
#108669=ORIENTED_EDGE ( 'NONE', *, *, #53035, .F. ) ;
#108700=ORIENTED_EDGE ( 'NONE', *, *, #114298, .T. ) ;
#108717=EDGE_CURVE ( 'NONE', #85078, #187938, #88378, .T. ) ;
#108769=CARTESIAN_POINT ( 'NONE',  ( -31.80000000000000782, -5.510910596163089556E-15, 42.29999999999999716 ) ) ;
#108802=CARTESIAN_POINT ( 'NONE',  ( -5.950531402560715689E-15, 38.81732327939063509, -5.124999997268813168 ) ) ;
#108845=ORIENTED_EDGE ( 'NONE', *, *, #149178, .T. ) ;
#108846=CARTESIAN_POINT ( 'NONE',  ( -23.48529157249600985, 32.32473071737754111, -6.049999994537625270 ) ) ;
#108908=ORIENTED_EDGE ( 'NONE', *, *, #118105, .F. ) ;
#108922=CARTESIAN_POINT ( 'NONE',  ( 22.44159573604009594, -16.30477369853687364, 144.1750000027311671 ) ) ;
#108946=CARTESIAN_POINT ( 'NONE',  ( -35.44323460151743888, 3.757829821678503546, 38.50466947567799991 ) ) ;
#108967=CARTESIAN_POINT ( 'NONE',  ( 30.73962218707677607, -22.33364281372841376, -6.947842220587805429 ) ) ;
#109036=CARTESIAN_POINT ( 'NONE',  ( -8.571926809382608425, 26.38167802310805854, 144.4750000027312069 ) ) ;
#109053=CARTESIAN_POINT ( 'NONE',  ( -8.906447517083060816, 27.41122689804195645, 141.8500000054623911 ) ) ;
#109134=CARTESIAN_POINT ( 'NONE',  ( -3.573655867282028392E-15, 2.428612866367529932E-14, 139.9999999999999716 ) ) ;
#109162=CARTESIAN_POINT ( 'NONE',  ( -22.81625015709509441, -31.40387420917324590, -8.824999997268811569 ) ) ;
#109167=CARTESIAN_POINT ( 'NONE',  ( 33.71430530369729439, 4.147805181855619416, 98.62971388258593208 ) ) ;
#109218=ORIENTED_EDGE ( 'NONE', *, *, #127529, .F. ) ;
#109263=CARTESIAN_POINT ( 'NONE',  ( -31.64990063023044442, 6.823060802858329943, 91.87658598273998223 ) ) ;
#109348=CARTESIAN_POINT ( 'NONE',  ( -5.950531402560715689E-15, 38.81732327939063509, -3.624999997268813168 ) ) ;
#109409=CARTESIAN_POINT ( 'NONE',  ( -3.573655867282028392E-15, 2.428612866367529932E-14, 2.000000000000000000 ) ) ;
#109437=CARTESIAN_POINT ( 'NONE',  ( 27.73933785331498569, 2.768321779492822058E-14, 141.8750000027311842 ) ) ;
#109450=ORIENTED_EDGE ( 'NONE', *, *, #51790, .F. ) ;
#109491=CARTESIAN_POINT ( 'NONE',  ( 32.00000000000000000, -1.130961319012580892E-14, 97.65000000000000568 ) ) ;
#109533=CARTESIAN_POINT ( 'NONE',  ( 28.82186960331491221, -9.364793116373624215, 145.1500000054623740 ) ) ;
#109696=ORIENTED_EDGE ( 'NONE', *, *, #144706, .T. ) ;
#109762=CARTESIAN_POINT ( 'NONE',  ( 33.84943726220063098, -0.7253354391803923384, 100.4638154892406021 ) ) ;
#109868=FACE_OUTER_BOUND ( 'NONE', #135068, .T. ) ;
#109884=CARTESIAN_POINT ( 'NONE',  ( -37.32596994906253229, -3.631267627803094644, 40.85341334860915907 ) ) ;
#109914=CARTESIAN_POINT ( 'NONE',  ( 28.82186960331499392, -9.364793116373510529, 146.8999999999999773 ) ) ;
#109940=CARTESIAN_POINT ( 'NONE',  ( 23.31738231874054534, 16.94106989632529192, 147.4500000054623854 ) ) ;
#109954=ORIENTED_EDGE ( 'NONE', *, *, #70616, .T. ) ;
#109977=ORIENTED_EDGE ( 'NONE', *, *, #93425, .T. ) ;
#110034=CARTESIAN_POINT ( 'NONE',  ( -27.73933785331498925, 2.428612866367529932E-14, 142.8750000027311842 ) ) ;
#110050=CARTESIAN_POINT ( 'NONE',  ( 23.31738231874054534, 16.94106989632529192, 141.4500000054623854 ) ) ;
#110053=LINE ( 'NONE', #153566, #128978 ) ;
#110151=CARTESIAN_POINT ( 'NONE',  ( -3.573655867282028392E-15, 2.428612866367529932E-14, -0.1220970790697140096 ) ) ;
#110157=CARTESIAN_POINT ( 'NONE',  ( -22.81625015709509441, -31.40387420917324590, -4.324999997268812457 ) ) ;
#110174=CARTESIAN_POINT ( 'NONE',  ( 11.40812507854755253, -35.11059874428192273, -4.524999997268813523 ) ) ;
#110182=ORIENTED_EDGE ( 'NONE', *, *, #154932, .T. ) ;
#110207=CARTESIAN_POINT ( 'NONE',  ( 34.38809498607732706, -6.739667044264573192, 48.29962152465627412 ) ) ;
#110212=CARTESIAN_POINT ( 'NONE',  ( 34.12434206616184440, 14.08647367304311260, -8.000000000000001776 ) ) ;
#110234=PLANE ( 'NONE',  #172618 ) ;
#110339=CARTESIAN_POINT ( 'NONE',  ( -37.99626262588766679, 2.428612866367529932E-14, -6.002157773949822861 ) ) ;
#110342=CARTESIAN_POINT ( 'NONE',  ( 22.81625015709510151, -31.40387420917324590, -8.424999997268812990 ) ) ;
#110394=CARTESIAN_POINT ( 'NONE',  ( 28.82186960331507208, 9.364793116373459014, 145.3500000054623911 ) ) ;
#110431=CARTESIAN_POINT ( 'NONE',  ( -5.359611314223446995E-15, 29.16686587814335496, 148.8750000027311842 ) ) ;
#110436=CARTESIAN_POINT ( 'NONE',  ( -27.73933785331498925, 2.428612866367529932E-14, 140.8750000027311842 ) ) ;
#110502=CARTESIAN_POINT ( 'NONE',  ( 22.44159573604009239, 16.30477369853692693, 142.5750000027311728 ) ) ;
#110523=CARTESIAN_POINT ( 'NONE',  ( 67.00000000000000000, -5.510910596163089556E-15, 39.49999999999996447 ) ) ;
#110551=FACE_BOUND ( 'NONE', #195349, .T. ) ;
#110587=ORIENTED_EDGE ( 'NONE', *, *, #18566, .F. ) ;
#110625=ADVANCED_FACE ( 'NONE', ( #44634 ), #28493, .F. ) ;
#110626=DIRECTION ( 'NONE',  ( 0.000000000000000000, 0.000000000000000000, -1.000000000000000000 ) ) ;
#110651=ADVANCED_FACE ( 'NONE', ( #93099 ), #45622, .F. ) ;
#110665=CARTESIAN_POINT ( 'NONE',  ( -11.40812507854755609, 35.11059874428196537, -1.024999997268813301 ) ) ;
#110754=CARTESIAN_POINT ( 'NONE',  ( 34.52594549653173317, 2.428612888752089207E-14, 89.49999999999897682 ) ) ;
#110789=CARTESIAN_POINT ( 'NONE',  ( 3.556970738554033499E-15, -38.81732327939057825, -4.124999997268814056 ) ) ;
#110861=CARTESIAN_POINT ( 'NONE',  ( 32.00000000000000000, -1.163414459189985801E-14, 95.00000000000000000 ) ) ;
#110878=CARTESIAN_POINT ( 'NONE',  ( 32.63052366545710470, -0.9798963808689128419, 87.54781425814060469 ) ) ;
#110893=EDGE_LOOP ( 'NONE', ( #153664, #114582, #83259, #175632 ) ) ;
#110906=CARTESIAN_POINT ( 'NONE',  ( 8.906447517083050158, 27.41122689804195645, 149.4000000000000057 ) ) ;
#110928=CARTESIAN_POINT ( 'NONE',  ( -28.82186960331499037, 2.428612866367529932E-14, 139.9999999999999716 ) ) ;
#110929=CARTESIAN_POINT ( 'NONE',  ( 17.81289503416610742, 24.51734667627700404, 141.5500000054623797 ) ) ;
#110973=ORIENTED_EDGE ( 'NONE', *, *, #177696, .T. ) ;
#111022=CARTESIAN_POINT ( 'NONE',  ( 8.571926809382603096, -26.38167802310801235, 141.4750000027312069 ) ) ;
#111139=DIRECTION ( 'NONE',  ( 0.000000000000000000, 0.000000000000000000, -1.000000000000000000 ) ) ;
#111146=CARTESIAN_POINT ( 'NONE',  ( -11.40812507854755609, 35.11059874428196537, -9.024999997268814411 ) ) ;
#111147=CARTESIAN_POINT ( 'NONE',  ( -33.85315667487628133, 2.014031266883448522E-14, 100.5000000000010232 ) ) ;
#111199=CARTESIAN_POINT ( 'NONE',  ( 34.67225235875022804, -7.109416101192572945, 42.56171885070867944 ) ) ;
#111204=DIRECTION ( 'NONE',  ( -1.000000000000000000, 0.000000000000000000, 0.000000000000000000 ) ) ;
#111224=CARTESIAN_POINT ( 'NONE',  ( 37.99626262588765258, 2.893932880411085066E-14, -5.002157773949823749 ) ) ;
#111230=CARTESIAN_POINT ( 'NONE',  ( 8.906447517083050158, 27.41122689804195645, 141.4000000000000057 ) ) ;
#111400=CARTESIAN_POINT ( 'NONE',  ( -32.00000000000000000, -1.096058885236868847E-14, 100.5000000000010232 ) ) ;
#111405=CARTESIAN_POINT ( 'NONE',  ( 3.765340386950246872E-15, -39.95163481335715971, -7.502157773949823749 ) ) ;
#111412=ORIENTED_EDGE ( 'NONE', *, *, #121041, .T. ) ;
#111424=EDGE_LOOP ( 'NONE', ( #139914, #172899 ) ) ;
#111430=CARTESIAN_POINT ( 'NONE',  ( -27.73933785331498925, -9.013057229001049109, 142.9750000027312069 ) ) ;
#111434=CARTESIAN_POINT ( 'NONE',  ( 22.44159573604009239, 16.30477369853692693, 140.0750000027311728 ) ) ;
#111465=VERTEX_POINT ( 'NONE', #128408 ) ;
#111501=CARTESIAN_POINT ( 'NONE',  ( 8.571926809382597767, 26.38167802310806209, 146.7750000027311899 ) ) ;
#111561=ADVANCED_FACE ( 'NONE', ( #64765, #125445 ), #159751, .F. ) ;
#111633=CARTESIAN_POINT ( 'NONE',  ( -35.44379935611748067, -3.753814927773975185, 38.50236686201313319 ) ) ;
#111650=EDGE_CURVE ( 'NONE', #120101, #167889, #65748, .T. ) ;
#111665=CARTESIAN_POINT ( 'NONE',  ( -36.91746825000000598, -11.99521256947794789, -4.524999997268813523 ) ) ;
#111752=CARTESIAN_POINT ( 'NONE',  ( 34.25242159400494302, -3.629837513186700448, 90.85215659754990725 ) ) ;
#111785=CARTESIAN_POINT ( 'NONE',  ( -36.91746825000001309, -11.99521256947794789, -10.52499999726881441 ) ) ;
#111875=CARTESIAN_POINT ( 'NONE',  ( 31.64921935833421429, -6.825000981063964467, 91.88079052344200193 ) ) ;
#111906=CARTESIAN_POINT ( 'NONE',  ( -17.14385361876520264, -23.59649016807271593, 139.6750000027311955 ) ) ;
#111930=CARTESIAN_POINT ( 'NONE',  ( -28.82186960331499392, 9.364793116373565596, 142.1500000054623740 ) ) ;
#112023=CARTESIAN_POINT ( 'NONE',  ( 17.14385361876520264, -23.59649016807270883, 143.5750000027311728 ) ) ;
#112034=CIRCLE ( 'NONE', #44219, 2.649999999999999467 ) ;
#112043=CYLINDRICAL_SURFACE ( 'NONE', #98102, 2.649999999999992806 ) ;
#112144=CARTESIAN_POINT ( 'NONE',  ( 29.86685920354754842, -21.69954338932559068, -5.824999997268813345 ) ) ;
#112169=AXIS2_PLACEMENT_3D ( 'NONE', #57443, #119116, #180797 ) ;
#112200=DIRECTION ( 'NONE',  ( 1.000000000000000000, -0.000000000000000000, 6.982962677686266711E-15 ) ) ;
#112228=FACE_OUTER_BOUND ( 'NONE', #8167, .T. ) ;
#112335=FACE_OUTER_BOUND ( 'NONE', #71340, .T. ) ;
#112364=CYLINDRICAL_SURFACE ( 'NONE', #34927, 28.82186960331498682 ) ;
#112386=CARTESIAN_POINT ( 'NONE',  ( -0.6913667201904812876, -37.16948018716584556, -7.999999999999996447 ) ) ;
#112389=EDGE_CURVE ( 'NONE', #24708, #114881, #123583, .T. ) ;
#112392=DIRECTION ( 'NONE',  ( 0.000000000000000000, 0.000000000000000000, -1.000000000000000000 ) ) ;
#112422=CARTESIAN_POINT ( 'NONE',  ( -17.14385361876520619, 23.59649016807275856, 142.5750000027312012 ) ) ;
#112491=CARTESIAN_POINT ( 'NONE',  ( -22.44159573604009950, -16.30477369853688430, 147.5750000027312012 ) ) ;
#112568=CARTESIAN_POINT ( 'NONE',  ( 23.48529157249600630, -32.32473071737749137, -3.049999994537627490 ) ) ;
#112570=AXIS2_PLACEMENT_3D ( 'NONE', #65203, #126862, #186595 ) ;
#112610=FACE_OUTER_BOUND ( 'NONE', #123706, .T. ) ;
#112618=CARTESIAN_POINT ( 'NONE',  ( 37.19778934971984796, 4.370295695334257324, 41.64163531972153720 ) ) ;
#112621=CARTESIAN_POINT ( 'NONE',  ( -35.50125023021173121, -3.320518091344054401, 38.27062242752714383 ) ) ;
#112652=CARTESIAN_POINT ( 'NONE',  ( 36.91746824999999887, -11.99521256947793546, -3.724999997268813257 ) ) ;
#112737=CARTESIAN_POINT ( 'NONE',  ( 33.85315667487628133, 2.428612866512670557E-14, 100.5000000000010232 ) ) ;
#112770=CARTESIAN_POINT ( 'NONE',  ( -38.00000000000001421, 12.34694845685046438, -0.09999999999999989453 ) ) ;
#112783=EDGE_CURVE ( 'NONE', #131569, #130647, #97875, .T. ) ;
#112797=AXIS2_PLACEMENT_3D ( 'NONE', #108769, #97546, #16767 ) ;
#112862=CARTESIAN_POINT ( 'NONE',  ( 31.45337032948814482, -4.959272002022362180, 100.6317495573355671 ) ) ;
#112892=CARTESIAN_POINT ( 'NONE',  ( 8.906447517083050158, 27.41122689804195645, 147.4000000000000057 ) ) ;
#112913=CARTESIAN_POINT ( 'NONE',  ( -17.81289503416611097, -24.51734667627696496, 140.5500000054623513 ) ) ;
#112935=CIRCLE ( 'NONE', #19422, 37.99626262588765968 ) ;
#112979=CARTESIAN_POINT ( 'NONE',  ( -6.019987952026119621E-15, 39.95163481335720235, -2.247842220587802586 ) ) ;
#113024=DIRECTION ( 'NONE',  ( 1.000000000000000000, 0.000000000000000000, 0.000000000000000000 ) ) ;
#113026=CARTESIAN_POINT ( 'NONE',  ( 36.99122028029233178, -5.215067209438918994, 43.21662174228440989 ) ) ;
#113126=CARTESIAN_POINT ( 'NONE',  ( -22.81625015709509441, -31.40387420917324590, -6.324999997268815122 ) ) ;
#113163=EDGE_CURVE ( 'NONE', #175994, #180473, #78562, .T. ) ;
#113183=CARTESIAN_POINT ( 'NONE',  ( 34.48175918554795061, -5.660046887242162761, 49.94512835368023218 ) ) ;
#113207=CARTESIAN_POINT ( 'NONE',  ( 23.48298174826589246, 32.32155151706776053, -4.702157773949823927 ) ) ;
#113407=CARTESIAN_POINT ( 'NONE',  ( -27.73933785331498925, 2.428612866367529932E-14, 149.3750000027311842 ) ) ;
#113477=CARTESIAN_POINT ( 'NONE',  ( -8.571926809382608425, 26.38167802310805854, 144.9750000027312069 ) ) ;
#113555=CARTESIAN_POINT ( 'NONE',  ( -38.00000000000001421, -12.34694845685042708, -5.649999994537625803 ) ) ;
#113568=VERTEX_POINT ( 'NONE', #36884 ) ;
#113605=CARTESIAN_POINT ( 'NONE',  ( -32.00000000000000000, -5.186379194389042044E-15, 42.35000000000000853 ) ) ;
#113606=CARTESIAN_POINT ( 'NONE',  ( 22.81625015709510151, -31.40387420917324590, -4.424999997268812990 ) ) ;
#113637=CARTESIAN_POINT ( 'NONE',  ( 11.40812507854755253, -35.11059874428192273, -4.024999997268814411 ) ) ;
#113740=EDGE_CURVE ( 'NONE', #26356, #177652, #59235, .T. ) ;
#113757=CARTESIAN_POINT ( 'NONE',  ( 23.48529157249599919, 32.32473071737754111, -0.6999999999999998446 ) ) ;
#113830=CYLINDRICAL_SURFACE ( 'NONE', #85369, 37.99626262588765968 ) ;
#113847=CARTESIAN_POINT ( 'NONE',  ( 32.53128430053961750, -2.419343514923771199, 87.89668391837237493 ) ) ;
#113865=ORIENTED_EDGE ( 'NONE', *, *, #17662, .T. ) ;
#113876=CARTESIAN_POINT ( 'NONE',  ( -28.82186960331499392, 9.364793116373565596, 147.8999999999999488 ) ) ;
#113898=CARTESIAN_POINT ( 'NONE',  ( 8.906447517083057264, -27.41122689804191026, 138.8500000054623911 ) ) ;
#113969=ADVANCED_FACE ( 'NONE', ( #148081 ), #135902, .T. ) ;
#114009=CARTESIAN_POINT ( 'NONE',  ( 36.82872320124401000, -3.359544971329622598, 49.36946820683672854 ) ) ;
#114112=CARTESIAN_POINT ( 'NONE',  ( -5.950531402560715689E-15, 38.81732327939063509, -3.124999997268813168 ) ) ;
#114188=CARTESIAN_POINT ( 'NONE',  ( 31.79999999999932214, 1.011436372600181938E-12, 97.70000000000020179 ) ) ;
#114274=CARTESIAN_POINT ( 'NONE',  ( -40.00200000000003087, -5.510910596163089556E-15, 45.00000000000000000 ) ) ;
#114298=EDGE_CURVE ( 'NONE', #85078, #38003, #34922, .T. ) ;
#114317=CARTESIAN_POINT ( 'NONE',  ( 36.91746825000000598, -11.99521256947793546, -10.22499999726881548 ) ) ;
#114332=ORIENTED_EDGE ( 'NONE', *, *, #135116, .T. ) ;
#114365=DIRECTION ( 'NONE',  ( 0.000000000000000000, 0.000000000000000000, -1.000000000000000000 ) ) ;
#114404=CARTESIAN_POINT ( 'NONE',  ( -17.14385361876520619, 23.59649016807275856, 145.0750000027311728 ) ) ;
#114437=CARTESIAN_POINT ( 'NONE',  ( 67.00000000000000000, -1.163414459189985801E-14, 89.49999999999897682 ) ) ;
#114476=CARTESIAN_POINT ( 'NONE',  ( -22.44159573604010305, 16.30477369853692338, 147.1750000027311671 ) ) ;
#114522=CARTESIAN_POINT ( 'NONE',  ( -38.00373040315628970, 1.963201398428686990E-14, -0.1220970790697140096 ) ) ;
#114560=CARTESIAN_POINT ( 'NONE',  ( 30.74264578624800137, -22.33583958711395212, -2.949999994537626957 ) ) ;
#114570=FACE_OUTER_BOUND ( 'NONE', #85524, .T. ) ;
#114582=ORIENTED_EDGE ( 'NONE', *, *, #178148, .T. ) ;
#114609=CARTESIAN_POINT ( 'NONE',  ( 36.91746824999999887, 11.99521256947799053, -2.024999997268813523 ) ) ;
#114643=CARTESIAN_POINT ( 'NONE',  ( -22.81625015709510507, 31.40387420917330275, -2.924999997268813434 ) ) ;
#114700=AXIS2_PLACEMENT_3D ( 'NONE', #125340, #170847, #32338 ) ;
#114769=CARTESIAN_POINT ( 'NONE',  ( 22.81625015709510151, -31.40387420917324590, -9.924999997268814766 ) ) ;
#114881=VERTEX_POINT ( 'NONE', #95329 ) ;
#114892=CARTESIAN_POINT ( 'NONE',  ( 23.31738231874054890, -16.94106989632523508, 142.7999999999999829 ) ) ;
#114894=CARTESIAN_POINT ( 'NONE',  ( -34.52594549653173317, 2.005792002353502844E-14, 89.49999999999897682 ) ) ;
#114913=AXIS2_PLACEMENT_3D ( 'NONE', #42699, #27544, #74034 ) ;
#114916=CARTESIAN_POINT ( 'NONE',  ( -28.82186960331499392, -9.364793116373526516, 138.3500000054623911 ) ) ;
#114927=( NAMED_UNIT ( * ) PLANE_ANGLE_UNIT ( ) SI_UNIT ( $, .RADIAN. ) );
#114937=CARTESIAN_POINT ( 'NONE',  ( 1.993301997531345686E-15, -30.30510711980685556, 142.5000000000000000 ) ) ;
#114970=VECTOR ( 'NONE', #75534, 1000.000000000000114 ) ;
#115061=VECTOR ( 'NONE', #191142, 1000.000000000000000 ) ;
#115121=DIRECTION ( 'NONE',  ( 0.000000000000000000, 0.000000000000000000, -1.000000000000000000 ) ) ;
#115308=EDGE_CURVE ( 'NONE', #57298, #60581, #14053, .T. ) ;
#115341=CARTESIAN_POINT ( 'NONE',  ( 35.73712089830454630, -9.569067683169670602, -7.999999999999996447 ) ) ;
#115409=ORIENTED_EDGE ( 'NONE', *, *, #59945, .F. ) ;
#115422=CARTESIAN_POINT ( 'NONE',  ( -31.23842136418743820, -7.314639034718686261, 96.67538241540150068 ) ) ;
#115426=CARTESIAN_POINT ( 'NONE',  ( 27.73933785331498925, -9.013057229001033122, 144.2750000027311899 ) ) ;
#115430=CARTESIAN_POINT ( 'NONE',  ( -37.99626262588766679, 2.428612866367529932E-14, -5.747842220587803475 ) ) ;
#115496=VECTOR ( 'NONE', #163614, 1000.000000000000000 ) ;
#115578=CARTESIAN_POINT ( 'NONE',  ( -23.48529157249599919, -32.32473071737750558, -3.449999994537626957 ) ) ;
#115613=CARTESIAN_POINT ( 'NONE',  ( 31.80025110837587832, 6.358902984670138814, 91.01589400111390660 ) ) ;
#115628=FACE_OUTER_BOUND ( 'NONE', #107361, .T. ) ;
#115658=CARTESIAN_POINT ( 'NONE',  ( -37.57676386873053076, 0.7175261378074869745, 39.53500980800841802 ) ) ;
#115755=LINE ( 'NONE', #100570, #101362 ) ;
#115780=CARTESIAN_POINT ( 'NONE',  ( 22.81625015709510151, -31.40387420917324590, -5.924999997268812990 ) ) ;
#115898=CARTESIAN_POINT ( 'NONE',  ( 28.82186960331498327, 9.364793116373570925, 145.1000000000000227 ) ) ;
#115949=CARTESIAN_POINT ( 'NONE',  ( -8.906447517083053711, -27.41122689804191026, 146.6500000054623740 ) ) ;
#115964=VERTEX_POINT ( 'NONE', #85139 ) ;
#116012=CARTESIAN_POINT ( 'NONE',  ( 1.784210473542230573E-15, -29.16686587814331588, 139.3750000027311842 ) ) ;
#116030=CARTESIAN_POINT ( 'NONE',  ( 36.88736642480385086, -1.774289666830916490, 50.21844423102493948 ) ) ;
#116056=ADVANCED_FACE ( 'NONE', ( #131662 ), #56830, .F. ) ;
#116289=CARTESIAN_POINT ( 'NONE',  ( -37.99626262588766679, 2.428612866367529932E-14, 2.000000000000000000 ) ) ;
#116331=CARTESIAN_POINT ( 'NONE',  ( 35.74560708664564856, 9.537923430963926918, -7.999999999999994671 ) ) ;
#116379=CARTESIAN_POINT ( 'NONE',  ( -36.89467761628205267, -8.593610866466510956, -7.999999999999994671 ) ) ;
#116413=CARTESIAN_POINT ( 'NONE',  ( -32.57158834789616009, -1.949426887445991685, 87.75361764676915755 ) ) ;
#116418=CARTESIAN_POINT ( 'NONE',  ( 27.73933785331498569, 2.768321779492822058E-14, 144.3750000027311842 ) ) ;
#116506=FACE_OUTER_BOUND ( 'NONE', #128502, .T. ) ;
#116571=CARTESIAN_POINT ( 'NONE',  ( 11.74264578624799427, 36.14014761921585972, -10.34999999453762598 ) ) ;
#116580=VERTEX_POINT ( 'NONE', #181182 ) ;
#116607=CARTESIAN_POINT ( 'NONE',  ( 31.60134953801815172, 3.338644055332157468, 101.7340227041929950 ) ) ;
#116621=DIRECTION ( 'NONE',  ( -1.000000000000000000, -0.000000000000000000, -0.000000000000000000 ) ) ;
#116623=CARTESIAN_POINT ( 'NONE',  ( -34.40736802160862595, -7.501760008519349654, 45.46231226804128767 ) ) ;
#116650=CARTESIAN_POINT ( 'NONE',  ( 23.76721391575371811, -30.09498488473221656, -7.911512314823321290 ) ) ;
#116730=FACE_BOUND ( 'NONE', #140317, .T. ) ;
#116735=DIRECTION ( 'NONE',  ( 0.000000000000000000, 0.000000000000000000, -1.000000000000000000 ) ) ;
#116758=CARTESIAN_POINT ( 'NONE',  ( 31.79999999999934346, 1.011436372600181938E-12, 95.00000000000021316 ) ) ;
#116772=CARTESIAN_POINT ( 'NONE',  ( 38.00000000000000711, -12.34694845685040754, -7.100000000000000533 ) ) ;
#116795=EDGE_CURVE ( 'NONE', #111465, #56681, #62082, .T. ) ;
#116835=EDGE_CURVE ( 'NONE', #60581, #57298, #135633, .T. ) ;
#116880=LINE ( 'NONE', #132054, #94792 ) ;
#116882=DIRECTION ( 'NONE',  ( 1.000000000000000000, 0.000000000000000000, -0.000000000000000000 ) ) ;
#116890=CARTESIAN_POINT ( 'NONE',  ( 23.31738231874054534, 16.94106989632529192, 143.1999999999999886 ) ) ;
#116943=CARTESIAN_POINT ( 'NONE',  ( -11.74149087413295511, 36.13659316521247433, -0.4021577739498228832 ) ) ;
#116948=ORIENTED_EDGE ( 'NONE', *, *, #169870, .T. ) ;
#117080=CARTESIAN_POINT ( 'NONE',  ( 8.906447517083050158, 27.41122689804195645, 145.4000000000000057 ) ) ;
#117095=CARTESIAN_POINT ( 'NONE',  ( 13.06108300879906103, 35.02243372997630644, -7.999999999999996447 ) ) ;
#117098=CARTESIAN_POINT ( 'NONE',  ( 23.31738231874054890, -16.94106989632523508, 144.7999999999999829 ) ) ;
#117112=VERTEX_POINT ( 'NONE', #105308 ) ;
#117128=CARTESIAN_POINT ( 'NONE',  ( -28.82186960331499037, 2.428612866367529932E-14, 144.0000000000000000 ) ) ;
#117149=CARTESIAN_POINT ( 'NONE',  ( -35.24576003106574973, 4.949822944371127242, 39.34410620168027606 ) ) ;
#117155=DIRECTION ( 'NONE',  ( 1.000000000000000000, 0.000000000000000000, 0.000000000000000000 ) ) ;
#117158=CARTESIAN_POINT ( 'NONE',  ( -3.573655867282028392E-15, 2.428612866367529932E-14, 2.000000000000000000 ) ) ;
#117188=CARTESIAN_POINT ( 'NONE',  ( -30.00000000000000000, -5.510910596163089556E-15, 45.00000000000000000 ) ) ;
#117379=CARTESIAN_POINT ( 'NONE',  ( -34.25242159400493591, -3.629837513186700892, 90.85215659754989304 ) ) ;
#117381=CARTESIAN_POINT ( 'NONE',  ( -23.43257786332091186, -29.32469887945705622, -7.999999999999994671 ) ) ;
#117393=CARTESIAN_POINT ( 'NONE',  ( 22.81625015709510151, -31.40387420917324590, -2.424999997268812990 ) ) ;
#117416=CARTESIAN_POINT ( 'NONE',  ( -31.37911219714120037, -7.435064219939695462, 93.98466263399197373 ) ) ;
#117420=CARTESIAN_POINT ( 'NONE',  ( -22.44159573604010305, 16.30477369853692338, 145.1750000027311671 ) ) ;
#117494=CARTESIAN_POINT ( 'NONE',  ( -8.571926809382608425, 26.38167802310805854, 140.9750000027312069 ) ) ;
#117536=CARTESIAN_POINT ( 'NONE',  ( -40.00200000000003087, -1.163414459189985801E-14, 87.50000000000000000 ) ) ;
#117568=CARTESIAN_POINT ( 'NONE',  ( 30.74264578624799782, 22.33583958711400541, -10.54999999453762705 ) ) ;
#117606=CARTESIAN_POINT ( 'NONE',  ( 31.48310541436861243, 7.250236049019784801, 93.01911755558080586 ) ) ;
#117611=STYLED_ITEM ( 'NONE', ( #148772 ), #35157 ) ;
#117615=CARTESIAN_POINT ( 'NONE',  ( 32.57158834789613877, -1.949426887446015888, 87.75361764676912912 ) ) ;
#117623=DIRECTION ( 'NONE',  ( 1.000000000000000000, 0.000000000000000000, 0.000000000000000000 ) ) ;
#117738=CARTESIAN_POINT ( 'NONE',  ( -32.15509708611487127, 4.949069787320341973, 89.34338315600297165 ) ) ;
#117782=CARTESIAN_POINT ( 'NONE',  ( 11.74264578624799427, 36.14014761921585972, -4.599999999999999645 ) ) ;
#117831=ORIENTED_EDGE ( 'NONE', *, *, #127434, .T. ) ;
#117858=PRODUCT_DEFINITION ( 'UNKNOWN', '', #169553, #82716 ) ;
#117904=CARTESIAN_POINT ( 'NONE',  ( 28.82186960331499392, -9.364793116373510529, 142.9000000000000057 ) ) ;
#117920=ORIENTED_EDGE ( 'NONE', *, *, #180435, .T. ) ;
#117957=CARTESIAN_POINT ( 'NONE',  ( 23.48298174826589246, 32.32155151706776053, -0.7021577739498228166 ) ) ;
#118105=EDGE_CURVE ( 'NONE', #130010, #153137, #54053, .T. ) ;
#118113=CARTESIAN_POINT ( 'NONE',  ( -17.81289503416611097, -24.51734667627696496, 144.2999999999999829 ) ) ;
#118162=CARTESIAN_POINT ( 'NONE',  ( -34.61352925372423783, 7.251504142776767914, 43.02394063628852194 ) ) ;
#118201=EDGE_LOOP ( 'NONE', ( #145989, #69959, #22366, #108908, #17911, #167198, #3407, #129546, #125080, #24198, #164920, #89327, #93375 ) ) ;
#118377=ORIENTED_EDGE ( 'NONE', *, *, #106236, .F. ) ;
#118385=CARTESIAN_POINT ( 'NONE',  ( -36.91746825000001309, 11.99521256947798342, -1.224999997268813035 ) ) ;
#118393=CARTESIAN_POINT ( 'NONE',  ( -33.98078611207405686, -16.46121673129812990, -8.000000000000001776 ) ) ;
#118427=ORIENTED_EDGE ( 'NONE', *, *, #43889, .F. ) ;
#118428=CARTESIAN_POINT ( 'NONE',  ( -31.26372923869873688, -6.750542664803635518, 98.30470173274466106 ) ) ;
#118432=CARTESIAN_POINT ( 'NONE',  ( 27.73933785331498925, -9.013057229001033122, 142.2750000027311899 ) ) ;
#118507=CARTESIAN_POINT ( 'NONE',  ( 17.14385361876520264, -23.59649016807270883, 140.0750000027311728 ) ) ;
#118553=AXIS2_PLACEMENT_3D ( 'NONE', #114188, #100026, #177897 ) ;
#118580=CARTESIAN_POINT ( 'NONE',  ( 36.91746824999999177, 2.880721459617395097E-14, -2.124999997268813168 ) ) ;
#118631=CARTESIAN_POINT ( 'NONE',  ( 36.76795047837062924, 4.947931209100013383, 47.42876213711300437 ) ) ;
#118649=ORIENTED_EDGE ( 'NONE', *, *, #140094, .F. ) ;
#118674=CARTESIAN_POINT ( 'NONE',  ( -27.73933785331498925, 2.428612866367529932E-14, 142.8750000027311842 ) ) ;
#118697=CIRCLE ( 'NONE', #121843, 5.500000000000032863 ) ;
#118747=CARTESIAN_POINT ( 'NONE',  ( -31.68361083058365679, 1.948458647159044155, 102.2466786067743101 ) ) ;
#118790=CARTESIAN_POINT ( 'NONE',  ( 11.74264578624799427, 36.14014761921585972, -2.600000000000000533 ) ) ;
#118842=ORIENTED_EDGE ( 'NONE', *, *, #21468, .T. ) ;
#118910=CARTESIAN_POINT ( 'NONE',  ( 1.993301997531345292E-15, -30.30510711980685912, 142.4999999999999716 ) ) ;
#118912=CARTESIAN_POINT ( 'NONE',  ( 23.31738231874054534, 16.94106989632529192, 143.4500000054623854 ) ) ;
#118927=ORIENTED_EDGE ( 'NONE', *, *, #92889, .T. ) ;
#118975=VERTEX_POINT ( 'NONE', #159357 ) ;
#119040=CARTESIAN_POINT ( 'NONE',  ( -30.82560697742735911, 1.994931101954655383E-14, 150.0000000000000000 ) ) ;
#119113=CARTESIAN_POINT ( 'NONE',  ( 20.47950280166127968, 31.12035828766152790, -8.000000000000000000 ) ) ;
#119116=DIRECTION ( 'NONE',  ( 0.000000000000000000, 0.000000000000000000, 1.000000000000000000 ) ) ;
#119164=CARTESIAN_POINT ( 'NONE',  ( -34.75593525676444528, 1.707450833175019334, 52.30717240064831230 ) ) ;
#119343=EDGE_CURVE ( 'NONE', #188321, #147696, #98073, .T. ) ;
#119359=FACE_OUTER_BOUND ( 'NONE', #182247, .T. ) ;
#119384=CARTESIAN_POINT ( 'NONE',  ( 22.81625015709509441, 31.40387420917330275, -3.824999997268813345 ) ) ;
#119390=CARTESIAN_POINT ( 'NONE',  ( -34.52594549653173317, 2.005792002353502844E-14, 89.49999999999897682 ) ) ;
#119391=CARTESIAN_POINT ( 'NONE',  ( -11.25158478316796185, -35.59826842325142593, -8.000000000000005329 ) ) ;
#119424=CARTESIAN_POINT ( 'NONE',  ( -32.58888545195123498, -1.708444646721626770, 87.69298048441147841 ) ) ;
#119498=CIRCLE ( 'NONE', #6440, 5.500000000000032863 ) ;
#119540=CARTESIAN_POINT ( 'NONE',  ( 38.00373040315627549, 2.428612866367529932E-14, -0.1220970790697140096 ) ) ;
#119575=CARTESIAN_POINT ( 'NONE',  ( -30.74264578624800492, -22.33583958711396278, -11.54999999453762527 ) ) ;
#119629=CARTESIAN_POINT ( 'NONE',  ( -34.54531151325589633, -4.968019249220468225, 50.63996542006479729 ) ) ;
#119658=CARTESIAN_POINT ( 'NONE',  ( -36.86305638906667781, 5.498848518248649064, 44.61989603102465196 ) ) ;
#119664=CARTESIAN_POINT ( 'NONE',  ( -27.73933785331498925, 9.013057229001089965, 146.7750000027312183 ) ) ;
#119669=CARTESIAN_POINT ( 'NONE',  ( 8.571926809382597767, 26.38167802310806209, 142.2750000027311899 ) ) ;
#119732=DIRECTION ( 'NONE',  ( 1.000000000000000000, -0.000000000000000000, -0.000000000000000000 ) ) ;
#119777=CARTESIAN_POINT ( 'NONE',  ( -38.00000000000001421, 12.34694845685046438, -4.100000000000000533 ) ) ;
#119826=CARTESIAN_POINT ( 'NONE',  ( 34.38590767368158652, 6.751198732549910986, 48.30327006964592584 ) ) ;
#120087=CARTESIAN_POINT ( 'NONE',  ( 4.205191997947069993, 37.27545319588617190, -8.000000000000000000 ) ) ;
#120090=CARTESIAN_POINT ( 'NONE',  ( 1.993301997531345686E-15, -30.30510711980685556, 140.7500000054623683 ) ) ;
#120101=VERTEX_POINT ( 'NONE', #102700 ) ;
#120116=CARTESIAN_POINT ( 'NONE',  ( -27.73933785331498925, 9.013057229001089965, 143.2750000027311899 ) ) ;
#120217=CARTESIAN_POINT ( 'NONE',  ( 11.74149087413295156, -36.13659316521243881, -3.402157773949823216 ) ) ;
#120246=CARTESIAN_POINT ( 'NONE',  ( -37.99626262588766679, 2.428612866367529932E-14, -2.002157773949823305 ) ) ;
#120361=CARTESIAN_POINT ( 'NONE',  ( -37.99626262588766679, 2.428612866367529932E-14, -2.002157773949823305 ) ) ;
#120430=CARTESIAN_POINT ( 'NONE',  ( -5.429308488886486681E-15, 30.30510711980690175, 139.7500000054623683 ) ) ;
#120543=CARTESIAN_POINT ( 'NONE',  ( -11.74264578624800670, 36.14014761921585972, -8.149999994537626691 ) ) ;
#120554=ORIENTED_EDGE ( 'NONE', *, *, #169979, .T. ) ;
#120557=ORIENTED_EDGE ( 'NONE', *, *, #8921, .T. ) ;
#120640=CARTESIAN_POINT ( 'NONE',  ( -5.359611314223446995E-15, 29.16686587814335496, 142.3750000027311557 ) ) ;
#120644=CARTESIAN_POINT ( 'NONE',  ( -67.00000000000000000, -1.163414459189985801E-14, 95.00000000000000000 ) ) ;
#120746=CARTESIAN_POINT ( 'NONE',  ( -23.48529157249599919, -32.32473071737750558, -3.699999999999999734 ) ) ;
#120793=( BOUNDED_CURVE ( )  B_SPLINE_CURVE ( 2, ( #45386, #107039, #162999, #168711, #84139, #24505, #69996, #179191, #85141, #86156, #193346, #147846, #9332, #70998, #132665, #102328, #164018, #25514, #154548, #187892, #157537, #200063, #50364, #46372, #63535, #123200, #184890, #80677, #170715, #32206, #1853, #33202, #3833, #93863, #850, #171712, #185896, #19031, #155541, #142353, #79694, #17035, #141364, #139369, #109036, #2851, #186906, #62523, #65512, #30213, #78689, #125210, #77702, #112023, #48377, #153548, #108031, #94860, #140366, #61531, #110034, #169717, #34192, #127173, #188883, #156541, #16043, #126196, #91856, #124196, #18040, #47381, #64529, #49359, #111022, #172708, #95853, #15045, #92861, #76706, #138382, #31210, #23010, #144339, #176704, #67503, #35180, #177702, #70510, #52334, #68498, #84656, #160517, #128171, #81650, #116012, #147354, #5827, #145338, #159504, #38178 ),
 .UNSPECIFIED., .F., .T. ) 
 B_SPLINE_CURVE_WITH_KNOTS ( ( 3, 2, 2, 2, 2, 2, 2, 2, 2, 2, 2, 2, 2, 2, 2, 2, 2, 2, 2, 2, 2, 2, 2, 2, 2, 2, 2, 2, 2, 2, 2, 2, 2, 2, 2, 2, 2, 2, 2, 2, 2, 2, 2, 2, 2, 2, 2, 2, 2, 2, 3 ),
 ( 0.000000000000000000, 0.02000000000000000042, 0.04000000000000000083, 0.05999999999999999778, 0.08000000000000000167, 0.1000000000000000056, 0.1199999999999999956, 0.1400000000000000133, 0.1600000000000000033, 0.1799999999999999933, 0.2000000000000000111, 0.2200000000000000011, 0.2399999999999999911, 0.2600000000000000089, 0.2800000000000000266, 0.2999999999999999889, 0.3200000000000000067, 0.3400000000000000244, 0.3599999999999999867, 0.3800000000000000044, 0.4000000000000000222, 0.4199999999999999845, 0.4400000000000000022, 0.4600000000000000200, 0.4799999999999999822, 0.5000000000000000000, 0.5200000000000000178, 0.5400000000000000355, 0.5600000000000000533, 0.5799999999999999600, 0.5999999999999999778, 0.6199999999999999956, 0.6400000000000000133, 0.6600000000000000311, 0.6800000000000000488, 0.6999999999999999556, 0.7199999999999999734, 0.7399999999999999911, 0.7600000000000000089, 0.7800000000000000266, 0.8000000000000000444, 0.8199999999999999512, 0.8399999999999999689, 0.8599999999999999867, 0.8800000000000000044, 0.9000000000000000222, 0.9200000000000000400, 0.9399999999999999467, 0.9599999999999999645, 0.9799999999999999822, 1.000000000000000000 ),
 .UNSPECIFIED. ) 
 CURVE ( )  GEOMETRIC_REPRESENTATION_ITEM ( )  RATIONAL_B_SPLINE_CURVE ( ( 1.000000000000000000, 0.9510565162951535312, 1.000000000000000000, 0.9510565162951535312, 1.000000000000000000, 0.9510565162951535312, 1.000000000000000000, 0.9510565162951535312, 1.000000000000000000, 0.9510565162951535312, 1.000000000000000000, 0.9510565162951535312, 1.000000000000000000, 0.9510565162951535312, 1.000000000000000000, 0.9510565162951535312, 1.000000000000000000, 0.9510565162951535312, 1.000000000000000000, 0.9510565162951535312, 1.000000000000000000, 0.9510565162951535312, 1.000000000000000000, 0.9510565162951535312, 1.000000000000000000, 0.9510565162951535312, 1.000000000000000000, 0.9510565162951535312, 1.000000000000000000, 0.9510565162951535312, 1.000000000000000000, 0.9510565162951535312, 1.000000000000000000, 0.9510565162951535312, 1.000000000000000000, 0.9510565162951535312, 1.000000000000000000, 0.9510565162951535312, 1.000000000000000000, 0.9510565162951535312, 1.000000000000000000, 0.9510565162951535312, 1.000000000000000000, 0.9510565162951535312, 1.000000000000000000, 0.9510565162951535312, 1.000000000000000000, 0.9510565162951535312, 1.000000000000000000, 0.9510565162951535312, 1.000000000000000000, 0.9510565162951535312, 1.000000000000000000, 0.9510565162951535312, 1.000000000000000000, 0.9510565162951535312, 1.000000000000000000, 0.9510565162951535312, 1.000000000000000000, 0.9510565162951535312, 1.000000000000000000, 0.9510565162951535312, 1.000000000000000000, 0.9510565162951535312, 1.000000000000000000, 0.9510565162951535312, 1.000000000000000000, 0.9510565162951535312, 1.000000000000000000, 0.9510565162951535312, 1.000000000000000000, 0.9510565162951535312, 1.000000000000000000, 0.9510565162951535312, 1.000000000000000000, 0.9510565162951535312, 1.000000000000000000, 0.9510565162951535312, 1.000000000000000000, 0.9510565162951535312, 1.000000000000000000, 0.9510565162951535312, 1.000000000000000000, 0.9510565162951535312, 1.000000000000000000, 0.9510565162951535312, 1.000000000000000000, 0.9510565162951535312, 1.000000000000000000, 0.9510565162951535312, 1.000000000000000000, 0.9510565162951535312, 1.000000000000000000, 0.9510565162951535312, 1.000000000000000000, 0.9510565162951535312, 1.000000000000000000, 0.9510565162951535312, 1.000000000000000000, 0.9510565162951535312, 1.000000000000000000 ) ) 
 REPRESENTATION_ITEM ( '' )  );
#120797=CARTESIAN_POINT ( 'NONE',  ( 34.45218533337745725, 5.971079431359537892, 49.56529461667047798 ) ) ;
#120867=CARTESIAN_POINT ( 'NONE',  ( 28.82186960331498327, 2.781578969918950771E-14, 139.2500000054623683 ) ) ;
#120879=AXIS2_PLACEMENT_3D ( 'NONE', #174773, #21080, #95931 ) ;
#120903=VECTOR ( 'NONE', #100276, 1000.000000000000000 ) ;
#120923=CARTESIAN_POINT ( 'NONE',  ( -37.99626262588765968, 12.34573411038917179, -0.1021577739498228665 ) ) ;
#120998=AXIS2_PLACEMENT_3D ( 'NONE', #140110, #153301, #155296 ) ;
#121041=EDGE_CURVE ( 'NONE', #117112, #200018, #11713, .T. ) ;
#121053=AXIS2_PLACEMENT_3D ( 'NONE', #92387, #15568, #47899 ) ;
#121057=AXIS2_PLACEMENT_3D ( 'NONE', #176305, #69110, #20606 ) ;
#121105=CARTESIAN_POINT ( 'NONE',  ( -27.73933785331498925, 9.013057229001089965, 141.2750000027311614 ) ) ;
#121130=CARTESIAN_POINT ( 'NONE',  ( 8.906447517083050158, 27.41122689804195645, 147.6500000054623740 ) ) ;
#121347=CARTESIAN_POINT ( 'NONE',  ( -5.950531402560715689E-15, 38.81732327939063509, -1.124999997268812946 ) ) ;
#121353=CARTESIAN_POINT ( 'NONE',  ( 33.82491520367208437, 1.773434586730185503, 100.2093774297293720 ) ) ;
#121415=EDGE_CURVE ( 'NONE', #136724, #103711, #112935, .T. ) ;
#121437=CARTESIAN_POINT ( 'NONE',  ( 8.906447517083057264, -27.41122689804191026, 142.8500000054623911 ) ) ;
#121535=CARTESIAN_POINT ( 'NONE',  ( 11.40812507854755253, -35.11059874428192273, -8.524999997268814411 ) ) ;
#121584=CARTESIAN_POINT ( 'NONE',  ( -8.906447517083060816, 27.41122689804195645, 143.5999999999999943 ) ) ;
#121586=CARTESIAN_POINT ( 'NONE',  ( 36.78370799935940028, 4.380135692641565548, 48.34576877258189143 ) ) ;
#121624=CARTESIAN_POINT ( 'NONE',  ( 27.73933785331498569, 2.768321779492822058E-14, 143.8750000027311842 ) ) ;
#121629=CARTESIAN_POINT ( 'NONE',  ( -8.571926809382601320, -26.38167802310801591, 141.2750000027311899 ) ) ;
#121634=LINE ( 'NONE', #42835, #180147 ) ;
#121652=VECTOR ( 'NONE', #176223, 1000.000000000000114 ) ;
#121792=CARTESIAN_POINT ( 'NONE',  ( 34.80630918731041845, 6.717782050307409492, 41.65621224074541828 ) ) ;
#121796=AXIS2_PLACEMENT_3D ( 'NONE', #56945, #99426, #130763 ) ;
#121843=AXIS2_PLACEMENT_3D ( 'NONE', #134283, #70606, #58423 ) ;
#121982=( BOUNDED_CURVE ( )  B_SPLINE_CURVE ( 2, ( #75208, #185369, #136879, #198565, #60035, #122694, #184383, #45864, #107517, #126656, #36637, #160997, #188359, #82129, #158008, #49837, #20479, #175171, #112491, #189357, #140842, #173187, #114476, #5303, #33669, #190341, #111501, #144819, #37649, #19499, #35653, #51817, #127657, #95331, #48848, #83144, #176179, #34663, #174185, #96321, #143822, #99313, #3325, #81144, #113477, #6303, #172184, #142825, #157016, #18514, #22492, #97301, #80161, #158987, #2331, #66987, #129635, #64012, #67981, #191331, #98294, #159996, #52809, #125681, #128646, #187379, #141833, #64998, #110502, #4305, #65987, #50834, #21483, #7301, #87159, #152553, #39649, #29235, #55821, #180197, #131664, #8320, #44397, #14041, #117494, #56832, #177188, #145818, #122210, #68986, #130650, #192344, #53826, #118507, #194353, #101310, #38661, #40659, #199065, #106051, #167737 ),
 .UNSPECIFIED., .F., .T. ) 
 B_SPLINE_CURVE_WITH_KNOTS ( ( 3, 2, 2, 2, 2, 2, 2, 2, 2, 2, 2, 2, 2, 2, 2, 2, 2, 2, 2, 2, 2, 2, 2, 2, 2, 2, 2, 2, 2, 2, 2, 2, 2, 2, 2, 2, 2, 2, 2, 2, 2, 2, 2, 2, 2, 2, 2, 2, 2, 2, 3 ),
 ( 0.000000000000000000, 0.02000000000000000042, 0.04000000000000000083, 0.05999999999999999778, 0.08000000000000000167, 0.1000000000000000056, 0.1199999999999999956, 0.1400000000000000133, 0.1600000000000000033, 0.1799999999999999933, 0.2000000000000000111, 0.2200000000000000011, 0.2399999999999999911, 0.2600000000000000089, 0.2800000000000000266, 0.2999999999999999889, 0.3200000000000000067, 0.3400000000000000244, 0.3599999999999999867, 0.3800000000000000044, 0.4000000000000000222, 0.4199999999999999845, 0.4400000000000000022, 0.4600000000000000200, 0.4799999999999999822, 0.5000000000000000000, 0.5200000000000000178, 0.5400000000000000355, 0.5600000000000000533, 0.5799999999999999600, 0.5999999999999999778, 0.6199999999999999956, 0.6400000000000000133, 0.6600000000000000311, 0.6800000000000000488, 0.6999999999999999556, 0.7199999999999999734, 0.7399999999999999911, 0.7600000000000000089, 0.7800000000000000266, 0.8000000000000000444, 0.8199999999999999512, 0.8399999999999999689, 0.8599999999999999867, 0.8800000000000000044, 0.9000000000000000222, 0.9200000000000000400, 0.9399999999999999467, 0.9599999999999999645, 0.9799999999999999822, 1.000000000000000000 ),
 .UNSPECIFIED. ) 
 CURVE ( )  GEOMETRIC_REPRESENTATION_ITEM ( )  RATIONAL_B_SPLINE_CURVE ( ( 1.000000000000000000, 0.9510565162951535312, 1.000000000000000000, 0.9510565162951535312, 1.000000000000000000, 0.9510565162951535312, 1.000000000000000000, 0.9510565162951535312, 1.000000000000000000, 0.9510565162951535312, 1.000000000000000000, 0.9510565162951535312, 1.000000000000000000, 0.9510565162951535312, 1.000000000000000000, 0.9510565162951535312, 1.000000000000000000, 0.9510565162951535312, 1.000000000000000000, 0.9510565162951535312, 1.000000000000000000, 0.9510565162951535312, 1.000000000000000000, 0.9510565162951535312, 1.000000000000000000, 0.9510565162951535312, 1.000000000000000000, 0.9510565162951535312, 1.000000000000000000, 0.9510565162951535312, 1.000000000000000000, 0.9510565162951535312, 1.000000000000000000, 0.9510565162951535312, 1.000000000000000000, 0.9510565162951535312, 1.000000000000000000, 0.9510565162951535312, 1.000000000000000000, 0.9510565162951535312, 1.000000000000000000, 0.9510565162951535312, 1.000000000000000000, 0.9510565162951535312, 1.000000000000000000, 0.9510565162951535312, 1.000000000000000000, 0.9510565162951535312, 1.000000000000000000, 0.9510565162951535312, 1.000000000000000000, 0.9510565162951535312, 1.000000000000000000, 0.9510565162951535312, 1.000000000000000000, 0.9510565162951535312, 1.000000000000000000, 0.9510565162951535312, 1.000000000000000000, 0.9510565162951535312, 1.000000000000000000, 0.9510565162951535312, 1.000000000000000000, 0.9510565162951535312, 1.000000000000000000, 0.9510565162951535312, 1.000000000000000000, 0.9510565162951535312, 1.000000000000000000, 0.9510565162951535312, 1.000000000000000000, 0.9510565162951535312, 1.000000000000000000, 0.9510565162951535312, 1.000000000000000000, 0.9510565162951535312, 1.000000000000000000, 0.9510565162951535312, 1.000000000000000000, 0.9510565162951535312, 1.000000000000000000, 0.9510565162951535312, 1.000000000000000000, 0.9510565162951535312, 1.000000000000000000, 0.9510565162951535312, 1.000000000000000000, 0.9510565162951535312, 1.000000000000000000, 0.9510565162951535312, 1.000000000000000000, 0.9510565162951535312, 1.000000000000000000, 0.9510565162951535312, 1.000000000000000000, 0.9510565162951535312, 1.000000000000000000, 0.9510565162951535312, 1.000000000000000000, 0.9510565162951535312, 1.000000000000000000 ) ) 
 REPRESENTATION_ITEM ( '' )  );
#122026=VERTEX_POINT ( 'NONE', #161127 ) ;
#122076=DIRECTION ( 'NONE',  ( 1.000000000000000000, 0.000000000000000000, 0.000000000000000000 ) ) ;
#122084=VERTEX_POINT ( 'NONE', #84270 ) ;
#122097=CARTESIAN_POINT ( 'NONE',  ( -27.73933785331498925, 2.428612866367529932E-14, 143.3750000027311842 ) ) ;
#122116=CARTESIAN_POINT ( 'NONE',  ( 31.99999999999932143, 1.011436372600181938E-12, 97.70000000000020179 ) ) ;
#122122=CARTESIAN_POINT ( 'NONE',  ( 28.82186960331498327, 9.364793116373570925, 145.3500000054623627 ) ) ;
#122210=CARTESIAN_POINT ( 'NONE',  ( 22.44159573604009239, 16.30477369853692693, 140.5750000027311728 ) ) ;
#122257=EDGE_LOOP ( 'NONE', ( #117920, #176811, #179521, #50799, #61576 ) ) ;
#122336=CARTESIAN_POINT ( 'NONE',  ( 22.81625015709510151, -31.40387420917324590, -8.424999997268812990 ) ) ;
#122337=CARTESIAN_POINT ( 'NONE',  ( -34.29436769411893238, 3.356737774573908872, 90.62828869849683144 ) ) ;
#122344=CARTESIAN_POINT ( 'NONE',  ( 33.67954790872092730, 5.223285087354250678, 96.76001495611576786 ) ) ;
#122441=CARTESIAN_POINT ( 'NONE',  ( -32.57470439124678308, 1.954246231034509895, 87.74243420032608753 ) ) ;
#122451=ORIENTED_EDGE ( 'NONE', *, *, #58814, .F. ) ;
#122463=CARTESIAN_POINT ( 'NONE',  ( 32.00000000000000000, -5.510910596163089556E-15, 45.00000000000000000 ) ) ;
#122527=CARTESIAN_POINT ( 'NONE',  ( -36.91746825000001309, 11.99521256947798342, -9.224999997268813701 ) ) ;
#122582=CARTESIAN_POINT ( 'NONE',  ( -8.906447517083060816, 27.41122689804195645, 145.8500000054623627 ) ) ;
#122619=CARTESIAN_POINT ( 'NONE',  ( 17.14385361876520264, -23.59649016807271238, 143.5750000027312012 ) ) ;
#122624=CARTESIAN_POINT ( 'NONE',  ( -8.571926809382601320, -26.38167802310801591, 147.2750000027311899 ) ) ;
#122694=CARTESIAN_POINT ( 'NONE',  ( -5.359611314223446995E-15, 29.16686587814335851, 148.8750000027311842 ) ) ;
#122731=CARTESIAN_POINT ( 'NONE',  ( 38.00000000000000000, 12.34694845685046616, -8.899999999999996803 ) ) ;
#122783=CARTESIAN_POINT ( 'NONE',  ( 34.51210051733096407, 7.446700168151136445, 43.98226744806001420 ) ) ;
#122833=CYLINDRICAL_SURFACE ( 'NONE', #185293, 5.500000000000032863 ) ;
#122841=ORIENTED_EDGE ( 'NONE', *, *, #19233, .T. ) ;
#123059=CARTESIAN_POINT ( 'NONE',  ( -36.86261346499077263, -5.499032313789903093, 44.62661474502114345 ) ) ;
#123062=CARTESIAN_POINT ( 'NONE',  ( -3.573655867282028392E-15, 2.428612866367529932E-14, -8.000000000000000000 ) ) ;
#123079=LINE ( 'NONE', #105930, #178682 ) ;
#123089=CARTESIAN_POINT ( 'NONE',  ( 17.14385361876520264, 23.59649016807275856, 146.6750000027311671 ) ) ;
#123113=CARTESIAN_POINT ( 'NONE',  ( -28.82186960331499037, 2.428612866367529932E-14, 144.2500000054623683 ) ) ;
#123135=CARTESIAN_POINT ( 'NONE',  ( 28.82186960331480208, -9.364793116373776982, 142.9000000000000057 ) ) ;
#123200=CARTESIAN_POINT ( 'NONE',  ( -5.359611314223446995E-15, 29.16686587814335851, 146.3750000027311842 ) ) ;
#123235=FACE_OUTER_BOUND ( 'NONE', #173045, .T. ) ;
#123253=CARTESIAN_POINT ( 'NONE',  ( 8.906447517083050158, 27.41122689804195645, 149.4000000000000057 ) ) ;
#123273=CARTESIAN_POINT ( 'NONE',  ( 29.43349580481983452, 2.428612866367529932E-14, 139.9999999999999716 ) ) ;
#123321=CARTESIAN_POINT ( 'NONE',  ( 3.556970738554033499E-15, -38.81732327939057825, -8.624999997268814056 ) ) ;
#123324=CARTESIAN_POINT ( 'NONE',  ( -11.74149087413294623, -36.13659316521243881, -3.347842220587804007 ) ) ;
#123327=CARTESIAN_POINT ( 'NONE',  ( 33.70615967800006985, 5.466638699193797635, 95.70352821367445983 ) ) ;
#123340=CARTESIAN_POINT ( 'NONE',  ( -11.40812507854754720, -35.11059874428192273, -6.724999997268813701 ) ) ;
#123379=DIRECTION ( 'NONE',  ( 0.000000000000000000, 0.000000000000000000, 1.000000000000000000 ) ) ;
#123403=CARTESIAN_POINT ( 'NONE',  ( 28.82186960331498327, 2.781578969918950771E-14, 141.0000000000000000 ) ) ;
#123424=CARTESIAN_POINT ( 'NONE',  ( -31.48310541436861953, 7.250236049019783913, 93.01911755558079165 ) ) ;
#123510=CARTESIAN_POINT ( 'NONE',  ( 11.40812507854754365, 35.11059874428196537, -5.724999997268812812 ) ) ;
#123583=CIRCLE ( 'NONE', #178620, 35.99626262588765258 ) ;
#123600=CARTESIAN_POINT ( 'NONE',  ( 27.73933785331498214, 9.013057229001095294, 145.9750000027311785 ) ) ;
#123605=CARTESIAN_POINT ( 'NONE',  ( -27.73933785331498925, 9.013057229001089965, 140.7750000027311899 ) ) ;
#123635=ORIENTED_EDGE ( 'NONE', *, *, #149591, .T. ) ;
#123690=EDGE_CURVE ( 'NONE', #53763, #98202, #61885, .T. ) ;
#123706=EDGE_LOOP ( 'NONE', ( #147544, #6011, #150712 ) ) ;
#123712=CARTESIAN_POINT ( 'NONE',  ( -30.74264578624800492, -22.33583958711396278, -9.799999999999998934 ) ) ;
#123762=CARTESIAN_POINT ( 'NONE',  ( 34.75593525676444528, 1.707450833175044425, 52.30717240064831941 ) ) ;
#123954=CARTESIAN_POINT ( 'NONE',  ( -36.91746825000001309, -11.99521256947794789, -4.524999997268813523 ) ) ;
#124077=CARTESIAN_POINT ( 'NONE',  ( 22.44159573604009239, 16.30477369853692693, 142.5750000027311728 ) ) ;
#124103=CARTESIAN_POINT ( 'NONE',  ( -5.429308488886486681E-15, 30.30510711980690175, 143.7500000054623399 ) ) ;
#124142=ORIENTED_EDGE ( 'NONE', *, *, #141815, .F. ) ;
#124196=CARTESIAN_POINT ( 'NONE',  ( 27.73933785331498569, 9.013057229001093518, 141.9750000027311785 ) ) ;
#124199=EDGE_LOOP ( 'NONE', ( #178647, #126982 ) ) ;
#124218=CARTESIAN_POINT ( 'NONE',  ( -3.573655867282028392E-15, 2.428612866367529932E-14, 6.432029388270255055E-14 ) ) ;
#124282=DIRECTION ( 'NONE',  ( -7.855351589328939542E-15, 0.000000000000000000, 1.000000000000000000 ) ) ;
#124319=DIRECTION ( 'NONE',  ( 1.000000000000000000, 0.000000000000000000, 0.000000000000000000 ) ) ;
#124326=CARTESIAN_POINT ( 'NONE',  ( -11.40812507854754720, -35.11059874428192273, -2.224999997268813701 ) ) ;
#124331=EDGE_CURVE ( 'NONE', #180473, #170159, #159880, .T. ) ;
#124386=CARTESIAN_POINT ( 'NONE',  ( 37.99626262588765258, 2.893932880411085066E-14, -1.002157773949823083 ) ) ;
#124441=CARTESIAN_POINT ( 'NONE',  ( -37.99626262588766679, 2.428612866367529932E-14, 2.000000000000000000 ) ) ;
#124522=CARTESIAN_POINT ( 'NONE',  ( -29.86685920354755552, 21.69954338932564397, -7.324999997268814234 ) ) ;
#124610=CARTESIAN_POINT ( 'NONE',  ( -17.14385361876520619, 23.59649016807275856, 149.0750000027311728 ) ) ;
#124725=CARTESIAN_POINT ( 'NONE',  ( -38.00000000000001421, 12.34694845685046438, -8.099999999999997868 ) ) ;
#124857=EDGE_CURVE ( 'NONE', #162507, #60180, #100200, .T. ) ;
#124883=VECTOR ( 'NONE', #159704, 1000.000000000000000 ) ;
#124972=CARTESIAN_POINT ( 'NONE',  ( 11.40812507854754365, 35.11059874428196537, -3.224999997268813701 ) ) ;
#125062=CARTESIAN_POINT ( 'NONE',  ( -37.54768727782017379, -1.429952535790612433, 39.67699414429139892 ) ) ;
#125080=ORIENTED_EDGE ( 'NONE', *, *, #137780, .F. ) ;
#125092=CARTESIAN_POINT ( 'NONE',  ( -17.81289503416611097, -24.51734667627696496, 146.2999999999999829 ) ) ;
#125117=CARTESIAN_POINT ( 'NONE',  ( 23.31738231874054534, 16.94106989632529192, 143.4500000054623854 ) ) ;
#125207=ORIENTED_EDGE ( 'NONE', *, *, #6551, .T. ) ;
#125210=CARTESIAN_POINT ( 'NONE',  ( 27.73933785331498925, -9.013057229001034898, 143.7750000027311614 ) ) ;
#125335=CARTESIAN_POINT ( 'NONE',  ( -22.81625015709510507, 31.40387420917330275, -8.924999997268814766 ) ) ;
#125340=CARTESIAN_POINT ( 'NONE',  ( -32.00000000000000000, -1.163414459189985801E-14, 95.00000000000000000 ) ) ;
#125353=CARTESIAN_POINT ( 'NONE',  ( -36.91746825000000598, 11.99521256947798520, -7.224999997268813701 ) ) ;
#125387=CARTESIAN_POINT ( 'NONE',  ( 34.57969012852954904, -4.582005219005605312, 50.95785156492174650 ) ) ;
#125416=CARTESIAN_POINT ( 'NONE',  ( -5.429308488886486681E-15, 30.30510711980690175, 141.5000000000000000 ) ) ;
#125445=FACE_OUTER_BOUND ( 'NONE', #82461, .T. ) ;
#125522=CARTESIAN_POINT ( 'NONE',  ( 36.91746825000000598, -11.99521256947793546, -8.224999997268810148 ) ) ;
#125572=CARTESIAN_POINT ( 'NONE',  ( 23.31738231874054534, 16.94106989632529192, 143.1999999999999886 ) ) ;
#125584=CARTESIAN_POINT ( 'NONE',  ( 37.99626262588768100, -12.34573411038909008, -7.102157773949824282 ) ) ;
#125602=CARTESIAN_POINT ( 'NONE',  ( 34.78522506798721992, 2.428612866353961525E-14, 52.50000000000000000 ) ) ;
#125607=CARTESIAN_POINT ( 'NONE',  ( 1.784210473542230573E-15, -29.16686587814331588, 139.3750000027311842 ) ) ;
#125681=CARTESIAN_POINT ( 'NONE',  ( -17.14385361876520975, 23.59649016807275856, 143.0750000027311444 ) ) ;
#125878=CARTESIAN_POINT ( 'NONE',  ( 31.99999999999968736, 4.791014396527177230E-13, 45.00000000000022027 ) ) ;
#125928=CARTESIAN_POINT ( 'NONE',  ( 34.42160027699925706, -2.272024392515961999, 89.98798656105708460 ) ) ;
#125962=CARTESIAN_POINT ( 'NONE',  ( -5.950531402560715689E-15, 38.81732327939063509, -3.124999997268813168 ) ) ;
#126036=DIRECTION ( 'NONE',  ( -1.000000000000000000, 0.000000000000000000, 0.000000000000000000 ) ) ;
#126052=CARTESIAN_POINT ( 'NONE',  ( -37.99626262588765968, 12.34573411038917179, -5.847842220587804896 ) ) ;
#126071=EDGE_LOOP ( 'NONE', ( #122451, #137054, #132805, #60628 ) ) ;
#126082=CARTESIAN_POINT ( 'NONE',  ( 8.906447517083050158, 27.41122689804195645, 145.4000000000000057 ) ) ;
#126105=CARTESIAN_POINT ( 'NONE',  ( -8.906447517083053711, -27.41122689804191026, 140.4000000000000057 ) ) ;
#126106=CARTESIAN_POINT ( 'NONE',  ( -17.81289503416611097, -24.51734667627696496, 142.5500000054623513 ) ) ;
#126123=CARTESIAN_POINT ( 'NONE',  ( 28.82186960331498327, 2.781578969918950771E-14, 147.0000000000000000 ) ) ;
#126196=CARTESIAN_POINT ( 'NONE',  ( 17.14385361876520264, 23.59649016807275856, 142.1750000027311671 ) ) ;
#126225=EDGE_CURVE ( 'NONE', #58436, #9032, #145542, .T. ) ;
#126316=CARTESIAN_POINT ( 'NONE',  ( -29.86685920354755197, -21.69954338932560134, -4.424999997268812990 ) ) ;
#126317=CARTESIAN_POINT ( 'NONE',  ( -33.82491520367208437, 1.773434586730183060, 100.2093774297293862 ) ) ;
#126369=CARTESIAN_POINT ( 'NONE',  ( 31.99999999999968736, 4.791014396527177230E-13, 45.00000000000022027 ) ) ;
#126558=DIRECTION ( 'NONE',  ( -6.982962677686266711E-15, 0.000000000000000000, 1.000000000000000000 ) ) ;
#126586=CARTESIAN_POINT ( 'NONE',  ( 27.73933785331498569, 2.768321779492822058E-14, 148.3750000027311842 ) ) ;
#126590=CARTESIAN_POINT ( 'NONE',  ( 22.44159573604009594, -16.30477369853687364, 139.6750000027311955 ) ) ;
#126656=CARTESIAN_POINT ( 'NONE',  ( 27.73933785331498569, 9.013057229001093518, 148.4750000027311785 ) ) ;
#126675=DIRECTION ( 'NONE',  ( -1.000000000000000000, 0.000000000000000000, 0.000000000000000000 ) ) ;
#126817=CARTESIAN_POINT ( 'NONE',  ( -22.81625015709510507, 31.40387420917330275, -4.924999997268813878 ) ) ;
#126834=VERTEX_POINT ( 'NONE', #41300 ) ;
#126862=DIRECTION ( 'NONE',  ( 0.000000000000000000, 0.000000000000000000, -1.000000000000000000 ) ) ;
#126873=AXIS2_PLACEMENT_3D ( 'NONE', #198008, #76637, #199996 ) ;
#126894=FACE_OUTER_BOUND ( 'NONE', #135389, .T. ) ;
#126905=CARTESIAN_POINT ( 'NONE',  ( 33.76764775315835010, -5.498935319396520249, 94.62547034095169352 ) ) ;
#126938=CARTESIAN_POINT ( 'NONE',  ( -29.86685920354755552, 21.69954338932564397, -6.824999997268814234 ) ) ;
#126968=AXIS2_PLACEMENT_3D ( 'NONE', #158055, #33717, #174232 ) ;
#126982=ORIENTED_EDGE ( 'NONE', *, *, #23933, .F. ) ;
#127048=AXIS2_PLACEMENT_3D ( 'NONE', #6301, #157014, #18512 ) ;
#127059=CARTESIAN_POINT ( 'NONE',  ( 8.571926809382597767, 26.38167802310806209, 140.7750000027311899 ) ) ;
#127080=CARTESIAN_POINT ( 'NONE',  ( 1.993301997531345686E-15, -30.30510711980685556, 140.5000000000000000 ) ) ;
#127081=CARTESIAN_POINT ( 'NONE',  ( -23.31738231874055245, -16.94106989632524574, 140.4500000054623854 ) ) ;
#127126=ORIENTED_EDGE ( 'NONE', *, *, #94442, .F. ) ;
#127173=CARTESIAN_POINT ( 'NONE',  ( -17.14385361876520975, 23.59649016807275856, 142.5750000027311728 ) ) ;
#127191=DIRECTION ( 'NONE',  ( 0.000000000000000000, 0.000000000000000000, 1.000000000000000000 ) ) ;
#127271=DIRECTION ( 'NONE',  ( 0.000000000000000000, 0.000000000000000000, 1.000000000000000000 ) ) ;
#127283=ORIENTED_EDGE ( 'NONE', *, *, #79968, .T. ) ;
#127296=CARTESIAN_POINT ( 'NONE',  ( -29.86685920354755197, -21.69954338932560134, -6.424999997268812990 ) ) ;
#127354=CARTESIAN_POINT ( 'NONE',  ( 34.38690502837283702, -7.455999864800775256, 45.95008414374197514 ) ) ;
#127378=DIRECTION ( 'NONE',  ( 1.000000000000000000, 0.000000000000000000, 0.000000000000000000 ) ) ;
#127434=EDGE_CURVE ( 'NONE', #177652, #57298, #196847, .T. ) ;
#127456=DIRECTION ( 'NONE',  ( 0.000000000000000000, 0.000000000000000000, -1.000000000000000000 ) ) ;
#127522=VECTOR ( 'NONE', #101756, 1000.000000000000000 ) ;
#127524=DIRECTION ( 'NONE',  ( 0.000000000000000000, 0.000000000000000000, -1.000000000000000000 ) ) ;
#127529=EDGE_CURVE ( 'NONE', #163891, #70870, #143025, .T. ) ;
#127541=AXIS2_PLACEMENT_3D ( 'NONE', #150211, #182532, #27873 ) ;
#127549=CARTESIAN_POINT ( 'NONE',  ( -33.74160284725413561, -3.639722220971261191, 99.13931652913684900 ) ) ;
#127550=CARTESIAN_POINT ( 'NONE',  ( 3.887666669675321707, -36.87873209731345270, -7.999999999999996447 ) ) ;
#127586=CARTESIAN_POINT ( 'NONE',  ( 27.73933785331498925, -9.013057229001033122, 148.2750000027311330 ) ) ;
#127657=CARTESIAN_POINT ( 'NONE',  ( 22.44159573604009594, -16.30477369853687364, 146.1750000027311671 ) ) ;
#127732=CARTESIAN_POINT ( 'NONE',  ( 11.74264578624799427, 36.14014761921585972, -4.349999994537626868 ) ) ;
#127781=CARTESIAN_POINT ( 'NONE',  ( 37.36578165719732425, 3.357000025855910064, 40.62839678089417816 ) ) ;
#127813=CARTESIAN_POINT ( 'NONE',  ( 36.91746824999999887, -11.99521256947793546, -5.724999997268813701 ) ) ;
#127882=FACE_OUTER_BOUND ( 'NONE', #146277, .T. ) ;
#127896=CARTESIAN_POINT ( 'NONE',  ( -30.00000000000000000, -40.00099999999999767, 37.49999999999999289 ) ) ;
#127901=CARTESIAN_POINT ( 'NONE',  ( 33.70211957050086937, -4.378872343537608458, 98.34732289368842828 ) ) ;
#127934=CARTESIAN_POINT ( 'NONE',  ( -11.74264578624800670, 36.14014761921585972, -0.3999999999999999112 ) ) ;
#128009=CARTESIAN_POINT ( 'NONE',  ( -30.00000000000000000, -5.510910596163089556E-15, 47.64999999999999147 ) ) ;
#128020=CARTESIAN_POINT ( 'NONE',  ( -30.00000000000000000, -5.510910596163089556E-15, 37.50000000000000000 ) ) ;
#128026=CARTESIAN_POINT ( 'NONE',  ( 32.42844225013696757, -3.321486864536503880, 88.27111922316778703 ) ) ;
#128035=DIRECTION ( 'NONE',  ( 1.000000000000000000, 0.000000000000000000, 0.000000000000000000 ) ) ;
#128057=CARTESIAN_POINT ( 'NONE',  ( 23.31738231874054890, -16.94106989632523508, 148.7999999999999829 ) ) ;
#128078=CARTESIAN_POINT ( 'NONE',  ( 28.82186960331498327, 2.781578969918950771E-14, 143.2500000054623683 ) ) ;
#128104=CARTESIAN_POINT ( 'NONE',  ( 17.81289503416611453, -24.51734667627695785, 146.9500000054623854 ) ) ;
#128112=VERTEX_POINT ( 'NONE', #130901 ) ;
#128171=CARTESIAN_POINT ( 'NONE',  ( 17.14385361876520264, -23.59649016807270883, 139.5750000027311444 ) ) ;
#128192=CARTESIAN_POINT ( 'NONE',  ( 36.87149605698873245, -2.274342727564266475, 50.01098105774816105 ) ) ;
#128292=CARTESIAN_POINT ( 'NONE',  ( -11.40812507854755609, 35.11059874428196537, -3.024999997268813523 ) ) ;
#128347=CARTESIAN_POINT ( 'NONE',  ( 35.68964480816959650, -0.9792624367684675812, 37.54765762180189625 ) ) ;
#128367=CARTESIAN_POINT ( 'NONE',  ( -28.28060372831499336, 2.428612866367529932E-14, 149.6875000013656063 ) ) ;
#128408=CARTESIAN_POINT ( 'NONE',  ( -28.82186960331499037, 2.428612866367529932E-14, 140.2500000054623683 ) ) ;
#128488=EDGE_CURVE ( 'NONE', #68886, #44815, #174150, .T. ) ;
#128502=EDGE_LOOP ( 'NONE', ( #55905, #115409, #17451, #145742 ) ) ;
#128514=CYLINDRICAL_SURFACE ( 'NONE', #22085, 37.99626262588765968 ) ;
#128575=CARTESIAN_POINT ( 'NONE',  ( 1.784210473542230573E-15, -29.16686587814331588, 147.8750000027311273 ) ) ;
#128580=CARTESIAN_POINT ( 'NONE',  ( -11.74149087413294623, -36.13659316521243881, -5.347842220587803119 ) ) ;
#128646=CARTESIAN_POINT ( 'NONE',  ( -8.571926809382608425, 26.38167802310805854, 142.9750000027312069 ) ) ;
#128723=CARTESIAN_POINT ( 'NONE',  ( -23.48529157249600985, 32.32473071737754111, -2.049999994537626158 ) ) ;
#128764=CARTESIAN_POINT ( 'NONE',  ( 31.99999999999966604, 4.791014396527177230E-13, 47.70000000000022311 ) ) ;
#128774=CARTESIAN_POINT ( 'NONE',  ( -11.40812507854755609, 35.11059874428196537, -1.524999997268813301 ) ) ;
#128806=CARTESIAN_POINT ( 'NONE',  ( 3.556970738554034288E-15, -38.81732327939057114, -2.124999997268813168 ) ) ;
#128924=CARTESIAN_POINT ( 'NONE',  ( 22.81625015709510151, -31.40387420917324590, -7.924999997268812990 ) ) ;
#128978=VECTOR ( 'NONE', #46392, 1000.000000000000114 ) ;
#128988=EDGE_LOOP ( 'NONE', ( #72322, #103270, #160575, #54448 ) ) ;
#129044=CARTESIAN_POINT ( 'NONE',  ( -17.81289503416611097, -24.51734667627696496, 148.2999999999999545 ) ) ;
#129065=CARTESIAN_POINT ( 'NONE',  ( 17.81289503416611453, -24.51734667627695785, 140.9500000054623285 ) ) ;
#129177=CARTESIAN_POINT ( 'NONE',  ( -32.00000000000000000, -1.163414459189985801E-14, 95.00000000000000000 ) ) ;
#129276=CARTESIAN_POINT ( 'NONE',  ( 37.99626262588765258, 2.893932880411085066E-14, -2.747842220587803475 ) ) ;
#129283=CARTESIAN_POINT ( 'NONE',  ( 22.81625015709510151, -31.40387420917324590, -7.924999997268812990 ) ) ;
#129284=CARTESIAN_POINT ( 'NONE',  ( -33.84955102792977755, 0.7177882281432041989, 100.4649514046632248 ) ) ;
#129324=ADVANCED_FACE ( 'NONE', ( #143826 ), #194357, .T. ) ;
#129528=CARTESIAN_POINT ( 'NONE',  ( 67.00000000000000000, -5.510910596163089556E-15, 45.00000000000000000 ) ) ;
#129546=ORIENTED_EDGE ( 'NONE', *, *, #69017, .F. ) ;
#129564=CARTESIAN_POINT ( 'NONE',  ( 1.784210473542230573E-15, -29.16686587814331588, 145.8750000027311273 ) ) ;
#129635=CARTESIAN_POINT ( 'NONE',  ( -8.571926809382601320, -26.38167802310801591, 143.7750000027311899 ) ) ;
#129712=CARTESIAN_POINT ( 'NONE',  ( -11.74264578624799782, -36.14014761921581709, -5.349999994537626868 ) ) ;
#129720=ORIENTED_EDGE ( 'NONE', *, *, #192515, .F. ) ;
#129761=CARTESIAN_POINT ( 'NONE',  ( 29.86685920354754842, -21.69954338932559068, -4.324999997268814234 ) ) ;
#129791=CARTESIAN_POINT ( 'NONE',  ( 29.86685920354754842, -21.69954338932559068, -5.824999997268813345 ) ) ;
#129912=CARTESIAN_POINT ( 'NONE',  ( 11.40812507854755253, -35.11059874428192273, -6.024999997268814411 ) ) ;
#129957=VERTEX_POINT ( 'NONE', #84142 ) ;
#130010=VERTEX_POINT ( 'NONE', #98297 ) ;
#130033=CARTESIAN_POINT ( 'NONE',  ( 8.906447517083050158, 27.41122689804195645, 143.4000000000000057 ) ) ;
#130056=CARTESIAN_POINT ( 'NONE',  ( 23.31738231874054890, -16.94106989632523508, 141.0500000054623513 ) ) ;
#130067=( LENGTH_UNIT ( ) NAMED_UNIT ( * ) SI_UNIT ( .MILLI., .METRE. ) );
#130090=LINE ( 'NONE', #160455, #78895 ) ;
#130095=EDGE_LOOP ( 'NONE', ( #2899, #6875 ) ) ;
#130121=EDGE_CURVE ( 'NONE', #26617, #134298, #48306, .T. ) ;
#130197=( BOUNDED_CURVE ( )  B_SPLINE_CURVE ( 2, ( #110339, #33509, #53656, #68819, #23326, #193177, #160836, #144657, #69823, #8146, #163846 ),
 .UNSPECIFIED., .F., .F. ) 
 B_SPLINE_CURVE_WITH_KNOTS ( ( 3, 2, 2, 2, 2, 3 ),
 ( 0.4000000000000001332, 0.4200000000000001510, 0.4400000000000000022, 0.4600000000000000200, 0.4799999999999999822, 0.5000000000000000000 ),
 .UNSPECIFIED. ) 
 CURVE ( )  GEOMETRIC_REPRESENTATION_ITEM ( )  RATIONAL_B_SPLINE_CURVE ( ( 0.9999999999999997780, 0.9510565162951537532, 1.000000000000000000, 0.9510565162951535312, 1.000000000000000000, 0.9510565162951535312, 1.000000000000000000, 0.9510565162951535312, 1.000000000000000000, 0.9510565162951535312, 1.000000000000000000 ) ) 
 REPRESENTATION_ITEM ( '' )  );
#130261=ORIENTED_EDGE ( 'NONE', *, *, #56324, .T. ) ;
#130274=CARTESIAN_POINT ( 'NONE',  ( -27.73933785331498925, 2.428612866367529932E-14, 149.3750000027311842 ) ) ;
#130275=CARTESIAN_POINT ( 'NONE',  ( -33.67954790872092730, 5.223285087354250678, 96.76001495611576786 ) ) ;
#130350=LINE ( 'NONE', #161713, #124883 ) ;
#130354=FACE_OUTER_BOUND ( 'NONE', #82412, .T. ) ;
#130455=ORIENTED_EDGE ( 'NONE', *, *, #1987, .T. ) ;
#130485=CARTESIAN_POINT ( 'NONE',  ( 36.91803858635991986, 1.187467863258684586, -8.000000000000005329 ) ) ;
#130533=CARTESIAN_POINT ( 'NONE',  ( -33.70061762759714696, -5.431516297171048890, 95.88384366041692886 ) ) ;
#130534=CARTESIAN_POINT ( 'NONE',  ( 8.398485719538898664, -36.04929410000102052, -7.999999999999994671 ) ) ;
#130575=CARTESIAN_POINT ( 'NONE',  ( 22.44159573604009594, -16.30477369853687364, 142.1750000027311671 ) ) ;
#130611=ORIENTED_EDGE ( 'NONE', *, *, #18566, .T. ) ;
#130647=VERTEX_POINT ( 'NONE', #75959 ) ;
#130650=CARTESIAN_POINT ( 'NONE',  ( 27.73933785331498569, 2.768321779492822058E-14, 140.3750000027311842 ) ) ;
#130721=CIRCLE ( 'NONE', #121057, 7.500000000000000000 ) ;
#130729=CARTESIAN_POINT ( 'NONE',  ( 38.00000000000000000, 12.34694845685046616, -6.649999994537624914 ) ) ;
#130763=DIRECTION ( 'NONE',  ( 0.000000000000000000, 0.000000000000000000, -1.000000000000000000 ) ) ;
#130777=LINE ( 'NONE', #113605, #198340 ) ;
#130778=CARTESIAN_POINT ( 'NONE',  ( -11.40812507854755609, 35.11059874428196537, -5.524999997268813523 ) ) ;
#130795=UNCERTAINTY_MEASURE_WITH_UNIT (LENGTH_MEASURE( 1.000000000000000082E-05 ), #151754, 'distance_accuracy_value', 'NONE');
#130810=CARTESIAN_POINT ( 'NONE',  ( -29.86685920354755197, -21.69954338932560134, -6.424999997268812990 ) ) ;
#130901=CARTESIAN_POINT ( 'NONE',  ( 28.82186960331498327, 2.781578969918950771E-14, 143.2500000054623683 ) ) ;
#130933=CARTESIAN_POINT ( 'NONE',  ( -11.40812507854755609, 35.11059874428196537, -7.024999997268813523 ) ) ;
#131038=VECTOR ( 'NONE', #83261, 1000.000000000000114 ) ;
#131055=CARTESIAN_POINT ( 'NONE',  ( -28.82186960331499392, -9.364793116373526516, 142.0999999999999659 ) ) ;
#131294=CARTESIAN_POINT ( 'NONE',  ( 1.784210473542230573E-15, -29.16686587814331588, 147.8750000027311273 ) ) ;
#131316=CARTESIAN_POINT ( 'NONE',  ( -34.40392893854400569, 6.519971432731296979, 48.73974290947565891 ) ) ;
#131322=CARTESIAN_POINT ( 'NONE',  ( -3.573655867282028392E-15, 2.428612866367529932E-14, 139.9999999999999716 ) ) ;
#131549=CARTESIAN_POINT ( 'NONE',  ( -11.74149087413294623, -36.13659316521243881, -1.602157773949822950 ) ) ;
#131569=VERTEX_POINT ( 'NONE', #122116 ) ;
#131587=CARTESIAN_POINT ( 'NONE',  ( -5.359611314223446995E-15, 29.16686587814335496, 146.8750000027311273 ) ) ;
#131611=CIRCLE ( 'NONE', #8944, 2.649999999999992806 ) ;
#131662=FACE_OUTER_BOUND ( 'NONE', #3002, .T. ) ;
#131664=CARTESIAN_POINT ( 'NONE',  ( -27.73933785331498925, 2.428612866367529932E-14, 141.3750000027311842 ) ) ;
#131707=LINE ( 'NONE', #114522, #121652 ) ;
#131740=CARTESIAN_POINT ( 'NONE',  ( -38.00000000000001421, 12.34694845685046438, -5.849999994537627757 ) ) ;
#131776=CARTESIAN_POINT ( 'NONE',  ( 31.72709406046301339, 0.4964181571218307387, 102.5000000000000284 ) ) ;
#131791=CARTESIAN_POINT ( 'NONE',  ( 37.24189295061466964, 4.138848244557342682, 41.36027101465354150 ) ) ;
#131823=CARTESIAN_POINT ( 'NONE',  ( 36.91746824999999887, -11.99521256947793546, -7.724999997268813701 ) ) ;
#131835=ORIENTED_EDGE ( 'NONE', *, *, #153999, .T. ) ;
#131932=FACE_OUTER_BOUND ( 'NONE', #181273, .T. ) ;
#131946=CARTESIAN_POINT ( 'NONE',  ( 30.74264578624799782, 22.33583958711400541, -4.800000000000000711 ) ) ;
#131993=DIRECTION ( 'NONE',  ( 1.000000000000000000, 0.000000000000000000, 3.709348145883536076E-20 ) ) ;
#132031=EDGE_CURVE ( 'NONE', #60180, #167889, #144744, .T. ) ;
#132054=CARTESIAN_POINT ( 'NONE',  ( -37.45873412500000654, 2.428612866367529932E-14, -1.437499995903219974 ) ) ;
#132064=CARTESIAN_POINT ( 'NONE',  ( 17.81289503416611453, -24.51734667627695785, 140.6999999999999602 ) ) ;
#132066=CARTESIAN_POINT ( 'NONE',  ( -17.81289503416611097, -24.51734667627696496, 138.5500000054623229 ) ) ;
#132126=ORIENTED_EDGE ( 'NONE', *, *, #192515, .T. ) ;
#132196=CARTESIAN_POINT ( 'NONE',  ( 36.91128768240056246, 2.428612879436746321E-14, 50.50000000000002842 ) ) ;
#132255=CARTESIAN_POINT ( 'NONE',  ( -28.82186960331489445, 9.364793116373697046, 145.8999999999999773 ) ) ;
#132270=CARTESIAN_POINT ( 'NONE',  ( 30.62874253898671384, 20.86932501997322476, -8.000000000000003553 ) ) ;
#132301=CARTESIAN_POINT ( 'NONE',  ( -36.91746825000000598, 2.428612866367529932E-14, -10.62499999726881406 ) ) ;
#132324=CARTESIAN_POINT ( 'NONE',  ( -34.67272174748971736, 7.108278434163710635, 42.55803597338269384 ) ) ;
#132346=CARTESIAN_POINT ( 'NONE',  ( -40.00200000000003087, -1.163414459189985801E-14, 95.00000000000000000 ) ) ;
#132355=DIRECTION ( 'NONE',  ( 1.000000000000000000, 0.000000000000000000, 3.709348145883536076E-20 ) ) ;
#132437=AXIS2_PLACEMENT_3D ( 'NONE', #44639, #140606, #107278 ) ;
#132590=CARTESIAN_POINT ( 'NONE',  ( 17.14385361876520264, -23.59649016807271238, 144.0750000027311444 ) ) ;
#132665=CARTESIAN_POINT ( 'NONE',  ( 8.571926809382603096, -26.38167802310801235, 147.4750000027311785 ) ) ;
#132737=CARTESIAN_POINT ( 'NONE',  ( 11.74264578624799427, 36.14014761921585972, -8.349999994537625980 ) ) ;
#132773=CARTESIAN_POINT ( 'NONE',  ( 32.42786921226272767, 3.325810949901237379, 88.27324663263311777 ) ) ;
#132787=CARTESIAN_POINT ( 'NONE',  ( 36.77234560139675779, 5.215770478161304347, 46.75454185840154508 ) ) ;
#132790=DIRECTION ( 'NONE',  ( 1.000000000000000000, 0.000000000000000000, 0.000000000000000000 ) ) ;
#132805=ORIENTED_EDGE ( 'NONE', *, *, #184390, .F. ) ;
#132806=ADVANCED_FACE ( 'NONE', ( #130354 ), #107880, .T. ) ;
#132819=DIRECTION ( 'NONE',  ( 0.06104853953485701173, 0.000000000000000000, -0.9981347984218670311 ) ) ;
#132900=CARTESIAN_POINT ( 'NONE',  ( -31.25711108810729755, 6.845500155895384076, 98.07395821223767030 ) ) ;
#132943=CARTESIAN_POINT ( 'NONE',  ( -23.48529157249599919, -32.32473071737750558, -1.699999999999999734 ) ) ;
#133060=CARTESIAN_POINT ( 'NONE',  ( -28.82186960331499392, 9.364793116373565596, 143.9000000000000057 ) ) ;
#133092=DIRECTION ( 'NONE',  ( -7.855351589328939542E-15, 0.000000000000000000, 1.000000000000000000 ) ) ;
#133190=CARTESIAN_POINT ( 'NONE',  ( 37.47059448506524149, -2.437326220201137872, 40.06626038917661958 ) ) ;
#133247=CARTESIAN_POINT ( 'NONE',  ( 28.82186960331511827, 9.364793116373395065, 145.0999999999999943 ) ) ;
#133265=CARTESIAN_POINT ( 'NONE',  ( -37.99626262588766679, 2.428612866367529932E-14, 6.432029388270255055E-14 ) ) ;
#133281=AXIS2_PLACEMENT_3D ( 'NONE', #90127, #197333, #107274 ) ;
#133317=CARTESIAN_POINT ( 'NONE',  ( -34.37178856895487655, 7.314363934749350094, 46.67665261413968381 ) ) ;
#133395=AXIS2_PLACEMENT_3D ( 'NONE', #70388, #101712, #116882 ) ;
#133499=FACE_OUTER_BOUND ( 'NONE', #144288, .T. ) ;
#133548=CARTESIAN_POINT ( 'NONE',  ( -30.34862450090452057, -22.29628711642643779, -7.999999999999994671 ) ) ;
#133583=CARTESIAN_POINT ( 'NONE',  ( -31.24012740013092326, -7.112679799535561287, 97.39185870086456021 ) ) ;
#133587=CARTESIAN_POINT ( 'NONE',  ( -22.44159573604010305, 16.30477369853692338, 141.1750000027311671 ) ) ;
#133714=ADVANCED_FACE ( 'NONE', ( #127882 ), #108327, .T. ) ;
#133736=CARTESIAN_POINT ( 'NONE',  ( -38.00000000000001421, -12.34694845685042708, -7.649999994537626691 ) ) ;
#133776=CARTESIAN_POINT ( 'NONE',  ( 32.33351994418282516, 3.967450966133691193, 88.63067128610951784 ) ) ;
#133824=CARTESIAN_POINT ( 'NONE',  ( -37.58407650405590061, 0.3600258186295099971, 39.49999999999997868 ) ) ;
#133835=CARTESIAN_POINT ( 'NONE',  ( 27.73933785331498569, 2.768321779492822058E-14, 145.8750000027311842 ) ) ;
#133924=AXIS2_PLACEMENT_3D ( 'NONE', #12807, #151318, #163495 ) ;
#133947=EDGE_LOOP ( 'NONE', ( #85536, #98649, #22489, #10532 ) ) ;
#133952=CARTESIAN_POINT ( 'NONE',  ( -11.74264578624800670, 36.14014761921585972, -4.400000000000000355 ) ) ;
#134060=ORIENTED_EDGE ( 'NONE', *, *, #78948, .T. ) ;
#134072=CARTESIAN_POINT ( 'NONE',  ( -8.906447517083053711, -27.41122689804191026, 140.4000000000000057 ) ) ;
#134214=VECTOR ( 'NONE', #154731, 1000.000000000000000 ) ;
#134280=CARTESIAN_POINT ( 'NONE',  ( 8.704215515294519534, 36.44267296588056837, -7.999999999999996447 ) ) ;
#134283=CARTESIAN_POINT ( 'NONE',  ( -32.00000000000000000, -5.510910596163089556E-15, 45.00000000000000000 ) ) ;
#134298=VERTEX_POINT ( 'NONE', #86053 ) ;
#134346=CYLINDRICAL_SURFACE ( 'NONE', #169059, 37.99626262588765968 ) ;
#134370=DIRECTION ( 'NONE',  ( -1.000000000000000000, 0.000000000000000000, 0.000000000000000000 ) ) ;
#134371=ORIENTED_EDGE ( 'NONE', *, *, #29683, .F. ) ;
#134390=AXIS2_PLACEMENT_3D ( 'NONE', #162621, #115121, #54451 ) ;
#134415=CARTESIAN_POINT ( 'NONE',  ( -37.99626262588762415, -12.34573411038919311, -3.902157773949822772 ) ) ;
#134527=EDGE_LOOP ( 'NONE', ( #98698, #166739, #152372, #9796 ) ) ;
#134557=CARTESIAN_POINT ( 'NONE',  ( 29.86685920354754842, -21.69954338932559068, -2.324999997268813345 ) ) ;
#134564=CARTESIAN_POINT ( 'NONE',  ( -5.271334918318021145, -36.86995875308960535, -7.999999999999994671 ) ) ;
#134577=CARTESIAN_POINT ( 'NONE',  ( -36.91746825000000598, 11.99521256947798520, -3.224999997268813257 ) ) ;
#134719=CARTESIAN_POINT ( 'NONE',  ( 17.81289503416610742, 24.51734667627700404, 147.2999999999999545 ) ) ;
#134751=CARTESIAN_POINT ( 'NONE',  ( 30.74264578624799782, 22.33583958711400541, -8.549999994537627046 ) ) ;
#134808=CARTESIAN_POINT ( 'NONE',  ( -34.75592306271660448, -1.707766843171850679, 52.30709029423474021 ) ) ;
#134837=CARTESIAN_POINT ( 'NONE',  ( 14.18669005401828187, -34.08280046153741694, -8.000000000000001776 ) ) ;
#134850=CARTESIAN_POINT ( 'NONE',  ( 17.14385361876520264, 23.59649016807275856, 146.1750000027311387 ) ) ;
#134855=DIRECTION ( 'NONE',  ( 1.000000000000000000, 0.000000000000000000, 0.000000000000000000 ) ) ;
#134960=CARTESIAN_POINT ( 'NONE',  ( 37.99999999999999289, 2.893978650043524126E-14, -3.000000000000000000 ) ) ;
#135020=EDGE_CURVE ( 'NONE', #108375, #136724, #42559, .T. ) ;
#135052=DIRECTION ( 'NONE',  ( -0.8660254037844391517, 0.000000000000000000, 0.4999999999999989453 ) ) ;
#135068=EDGE_LOOP ( 'NONE', ( #44209, #161081, #5242 ) ) ;
#135079=CARTESIAN_POINT ( 'NONE',  ( -8.906447517083060816, 27.41122689804195645, 147.8500000054623627 ) ) ;
#135081=CARTESIAN_POINT ( 'NONE',  ( -28.82186960331499037, 2.428612866367529932E-14, 138.2500000054623683 ) ) ;
#135116=EDGE_CURVE ( 'NONE', #163891, #54169, #164910, .T. ) ;
#135134=CARTESIAN_POINT ( 'NONE',  ( -30.73962218707678673, 22.33364281372846705, -0.2021577739498228998 ) ) ;
#135283=DIRECTION ( 'NONE',  ( 1.000000000000000000, -0.000000000000000000, -0.000000000000000000 ) ) ;
#135298=CARTESIAN_POINT ( 'NONE',  ( -30.00000000000000000, 40.00100000000004741, 37.49999999999999289 ) ) ;
#135309=CARTESIAN_POINT ( 'NONE',  ( -17.14385361876520264, -23.59649016807271593, 143.6750000027311671 ) ) ;
#135316=CARTESIAN_POINT ( 'NONE',  ( 31.79999999999968807, 4.791014396527177230E-13, 45.00000000000022027 ) ) ;
#135389=EDGE_LOOP ( 'NONE', ( #90331, #68836, #102269, #58711 ) ) ;
#135528=CYLINDRICAL_SURFACE ( 'NONE', #153839, 7.500000000000000000 ) ;
#135552=CARTESIAN_POINT ( 'NONE',  ( -11.40812507854754720, -35.11059874428192273, -4.724999997268812812 ) ) ;
#135570=CARTESIAN_POINT ( 'NONE',  ( -22.81625015709510507, 31.40387420917330275, -1.424999997268813212 ) ) ;
#135601=FILL_AREA_STYLE_COLOUR ( '', #136953 ) ;
#135633=CIRCLE ( 'NONE', #132437, 2.700000000000001066 ) ;
#135641=CARTESIAN_POINT ( 'NONE',  ( 1.993301997531345686E-15, -30.30510711980685556, 142.7500000054623683 ) ) ;
#135698=ADVANCED_FACE ( 'NONE', ( #98377 ), #165095, .T. ) ;
#135740=CARTESIAN_POINT ( 'NONE',  ( 36.91746825000000598, -11.99521256947793546, -2.224999997268813701 ) ) ;
#135829=ADVANCED_FACE ( 'NONE', ( #112335 ), #35496, .F. ) ;
#135831=CARTESIAN_POINT ( 'NONE',  ( -27.73933785331498925, 2.428612866367529932E-14, 148.8750000027311842 ) ) ;
#135836=CARTESIAN_POINT ( 'NONE',  ( -17.14385361876520619, 23.59649016807275856, 146.5750000027311444 ) ) ;
#135902=CYLINDRICAL_SURFACE ( 'NONE', #85051, 7.500000000000007105 ) ;
#135944=CARTESIAN_POINT ( 'NONE',  ( 30.74264578624799782, 22.33583958711400541, -6.800000000000000711 ) ) ;
#136242=PLANE ( 'NONE',  #27248 ) ;
#136256=CARTESIAN_POINT ( 'NONE',  ( 12.34766581223309245, 35.29190279822739740, -8.000000000000007105 ) ) ;
#136286=CARTESIAN_POINT ( 'NONE',  ( -22.44159573604009950, -16.30477369853688430, 141.5750000027311728 ) ) ;
#136311=CARTESIAN_POINT ( 'NONE',  ( -23.31738231874055245, -16.94106989632524574, 144.4500000054623854 ) ) ;
#136387=CARTESIAN_POINT ( 'NONE',  ( -11.74149087413294623, -36.13659316521243881, -3.602157773949823394 ) ) ;
#136523=CARTESIAN_POINT ( 'NONE',  ( -36.91746825000001309, 11.99521256947798342, -0.7249999972688133676 ) ) ;
#136632=VERTEX_POINT ( 'NONE', #14124 ) ;
#136710=CARTESIAN_POINT ( 'NONE',  ( 23.48529157249600630, -32.32473071737749137, -9.049999994537627046 ) ) ;
#136724=VERTEX_POINT ( 'NONE', #89980 ) ;
#136793=CARTESIAN_POINT ( 'NONE',  ( -36.81592377195798349, 3.639597414954541144, 49.13916779353752418 ) ) ;
#136806=CARTESIAN_POINT ( 'NONE',  ( 8.571926809382603096, -26.38167802310801235, 141.4750000027312069 ) ) ;
#136879=CARTESIAN_POINT ( 'NONE',  ( -22.44159573604010305, 16.30477369853692338, 149.1750000027311671 ) ) ;
#136920=CARTESIAN_POINT ( 'NONE',  ( -28.28060372831499336, 2.428612866367529932E-14, 139.6875000013656063 ) ) ;
#136953=COLOUR_RGB ( '', 0.66274510, 0.83137255, 0.94901961) ;
#136969=CARTESIAN_POINT ( 'NONE',  ( 34.61352925372422362, 7.251504142776767026, 43.02394063628852194 ) ) ;
#137023=ORIENTED_EDGE ( 'NONE', *, *, #66474, .T. ) ;
#137048=EDGE_CURVE ( 'NONE', #176832, #106856, #97891, .T. ) ;
#137054=ORIENTED_EDGE ( 'NONE', *, *, #79191, .T. ) ;
#137199=ORIENTED_EDGE ( 'NONE', *, *, #79032, .T. ) ;
#137258=ADVANCED_FACE ( 'NONE', ( #35258 ), #34272, .F. ) ;
#137275=CARTESIAN_POINT ( 'NONE',  ( -8.571926809382601320, -26.38167802310801591, 143.7750000027311899 ) ) ;
#137299=CARTESIAN_POINT ( 'NONE',  ( -23.31738231874055600, 16.94106989632528837, 144.0500000054623513 ) ) ;
#137317=DIRECTION ( 'NONE',  ( 0.000000000000000000, -1.000000000000000000, 0.000000000000000000 ) ) ;
#137333=ORIENTED_EDGE ( 'NONE', *, *, #176321, .T. ) ;
#137373=CARTESIAN_POINT ( 'NONE',  ( 30.00000000000000711, -5.510910596163089556E-15, 45.00000000000000000 ) ) ;
#137514=CARTESIAN_POINT ( 'NONE',  ( -36.91746825000001309, -11.99521256947794789, -2.524999997268813523 ) ) ;
#137520=CARTESIAN_POINT ( 'NONE',  ( 34.25194412823101686, 3.632597792548375448, 90.85486465461555383 ) ) ;
#137596=VERTEX_POINT ( 'NONE', #171792 ) ;
#137618=CARTESIAN_POINT ( 'NONE',  ( -32.53418548917481701, 2.421649558188280427, 87.88477275112326481 ) ) ;
#137640=DIRECTION ( 'NONE',  ( 0.000000000000000000, 0.000000000000000000, -1.000000000000000000 ) ) ;
#137703=CARTESIAN_POINT ( 'NONE',  ( 3.556970738554033499E-15, -38.81732327939057825, -8.624999997268814056 ) ) ;
#137752=CARTESIAN_POINT ( 'NONE',  ( -23.31738231874055600, 16.94106989632528837, 143.7999999999999829 ) ) ;
#137780=EDGE_CURVE ( 'NONE', #38003, #59237, #163075, .T. ) ;
#137793=CARTESIAN_POINT ( 'NONE',  ( -22.44159573604009950, -16.30477369853688430, 145.0750000027311728 ) ) ;
#137799=CARTESIAN_POINT ( 'NONE',  ( 17.14385361876520264, -23.59649016807271238, 141.5750000027312012 ) ) ;
#137822=AXIS2_PLACEMENT_3D ( 'NONE', #43605, #13270, #192553 ) ;
#137868=AXIS2_PLACEMENT_3D ( 'NONE', #128367, #190063, #175892 ) ;
#137890=CARTESIAN_POINT ( 'NONE',  ( 17.81289503416611453, -24.51734667627695785, 144.9500000054623854 ) ) ;
#137910=CARTESIAN_POINT ( 'NONE',  ( -38.00000000000000711, 2.428612866367529932E-14, -10.00000000000000000 ) ) ;
#137961=PLANE ( 'NONE',  #108269 ) ;
#138032=CARTESIAN_POINT ( 'NONE',  ( -40.00200000000003087, -4.592425496802575156E-15, 52.50000000000000000 ) ) ;
#138138=AXIS2_PLACEMENT_3D ( 'NONE', #42307, #43293, #197969 ) ;
#138155=CARTESIAN_POINT ( 'NONE',  ( -36.91746825000000598, 2.428612866367529932E-14, -4.624999997268814056 ) ) ;
#138270=CARTESIAN_POINT ( 'NONE',  ( 17.14385361876520264, 23.59649016807275856, 144.6750000027311671 ) ) ;
#138295=CARTESIAN_POINT ( 'NONE',  ( 8.906447517083050158, 27.41122689804195645, 145.6500000054623740 ) ) ;
#138316=CARTESIAN_POINT ( 'NONE',  ( -23.48298174826589602, -32.32155151706771790, -7.447842220587802764 ) ) ;
#138382=CARTESIAN_POINT ( 'NONE',  ( -27.73933785331498925, 2.428612866367529932E-14, 140.8750000027311842 ) ) ;
#138390=ADVANCED_FACE ( 'NONE', ( #77540, #105895 ), #136242, .T. ) ;
#138397=CARTESIAN_POINT ( 'NONE',  ( 17.81289503416610742, 24.51734667627700404, 141.5500000054623513 ) ) ;
#138435=CARTESIAN_POINT ( 'NONE',  ( -17.81289503416611808, 24.51734667627700404, 149.6999999999999602 ) ) ;
#138503=CARTESIAN_POINT ( 'NONE',  ( -36.91746825000001309, 11.99521256947798342, -9.224999997268813701 ) ) ;
#138508=CARTESIAN_POINT ( 'NONE',  ( 33.78659134798514430, 2.758747016945830133, 99.77194732211482631 ) ) ;
#138519=CARTESIAN_POINT ( 'NONE',  ( 36.91746824999999887, -11.99521256947793546, -6.224999997268814589 ) ) ;
#138604=CARTESIAN_POINT ( 'NONE',  ( -31.24009710442677701, 7.113574878955727598, 97.38907943302068304 ) ) ;
#138691=CARTESIAN_POINT ( 'NONE',  ( -5.950531402560715689E-15, 38.81732327939063509, -5.624999997268812280 ) ) ;
#138770=CARTESIAN_POINT ( 'NONE',  ( -28.82186960331499037, 2.428612866367529932E-14, 139.9999999999999716 ) ) ;
#138776=CARTESIAN_POINT ( 'NONE',  ( -36.77035430826401097, 5.154579508995667858, 46.92692430510570034 ) ) ;
#138944=ORIENTED_EDGE ( 'NONE', *, *, #166279, .F. ) ;
#138945=CARTESIAN_POINT ( 'NONE',  ( 34.74703179323498148, 1.946018278951714198, 52.24735473369668171 ) ) ;
#139003=VERTEX_POINT ( 'NONE', #128009 ) ;
#139087=( BOUNDED_CURVE ( )  B_SPLINE_CURVE ( 2, ( #176636, #144273, #163460, #128104, #145272, #193804, #115949, #5760, #24958, #66443, #4754 ),
 .UNSPECIFIED., .F., .F. ) 
 B_SPLINE_CURVE_WITH_KNOTS ( ( 3, 2, 2, 2, 2, 3 ),
 ( 0.1000000000000000888, 0.1200000000000000927, 0.1400000000000001243, 0.1600000000000001421, 0.1800000000000001321, 0.2000000000000001776 ),
 .UNSPECIFIED. ) 
 CURVE ( )  GEOMETRIC_REPRESENTATION_ITEM ( )  RATIONAL_B_SPLINE_CURVE ( ( 0.9999999999999997780, 0.9510565162951537532, 1.000000000000000000, 0.9510565162951535312, 1.000000000000000000, 0.9510565162951535312, 1.000000000000000000, 0.9510565162951535312, 1.000000000000000000, 0.9510565162951530871, 1.000000000000000444 ) ) 
 REPRESENTATION_ITEM ( '' )  );
#139173=ADVANCED_FACE ( 'NONE', ( #80516 ), #113830, .T. ) ;
#139182=EDGE_CURVE ( 'NONE', #45563, #89527, #66023, .T. ) ;
#139214=CARTESIAN_POINT ( 'NONE',  ( -3.573655867282028392E-15, 2.428612866367529932E-14, 139.9999999999999716 ) ) ;
#139229=CARTESIAN_POINT ( 'NONE',  ( -36.89003987753539349, -5.463308683677073674, 44.27017301194418764 ) ) ;
#139238=DIRECTION ( 'NONE',  ( 0.000000000000000000, 0.000000000000000000, 1.000000000000000000 ) ) ;
#139259=CARTESIAN_POINT ( 'NONE',  ( 8.571926809382597767, 26.38167802310806209, 142.7750000027311899 ) ) ;
#139283=CARTESIAN_POINT ( 'NONE',  ( 8.906447517083057264, -27.41122689804191026, 146.8500000054623627 ) ) ;
#139303=CARTESIAN_POINT ( 'NONE',  ( 17.81289503416611453, -24.51734667627695785, 142.6999999999999886 ) ) ;
#139324=ADVANCED_FACE ( 'NONE', ( #48212 ), #49203, .F. ) ;
#139369=CARTESIAN_POINT ( 'NONE',  ( -17.14385361876520975, 23.59649016807275856, 144.5750000027311728 ) ) ;
#139422=CARTESIAN_POINT ( 'NONE',  ( -5.429308488886486681E-15, 30.30510711980690175, 149.5000000000000000 ) ) ;
#139480=EDGE_LOOP ( 'NONE', ( #131835, #176527, #187889, #23584, #103180, #120554, #70384, #11133, #189269, #106205, #61946, #164015 ) ) ;
#139491=CARTESIAN_POINT ( 'NONE',  ( 36.91746825000000598, -11.99521256947793546, -1.724999997268813479 ) ) ;
#139508=CARTESIAN_POINT ( 'NONE',  ( -36.91746825000000598, 2.428612866367529932E-14, -7.124999997268813168 ) ) ;
#139531=CARTESIAN_POINT ( 'NONE',  ( -31.43434485161624536, -5.140865793513094140, 100.4663950908259409 ) ) ;
#139592=CARTESIAN_POINT ( 'NONE',  ( -31.76179951907201371, 6.484602924383671585, 91.22381659560100786 ) ) ;
#139675=CARTESIAN_POINT ( 'NONE',  ( 36.91746824999999177, 2.880721459617395097E-14, -6.124999997268813168 ) ) ;
#139684=EDGE_CURVE ( 'NONE', #46374, #189055, #54417, .T. ) ;
#139690=ORIENTED_EDGE ( 'NONE', *, *, #158172, .T. ) ;
#139725=CARTESIAN_POINT ( 'NONE',  ( -17.81289503416611808, 24.51734667627700404, 143.6999999999999886 ) ) ;
#139726=CARTESIAN_POINT ( 'NONE',  ( 28.82186960331498327, 2.781578969918950771E-14, 145.2500000054623683 ) ) ;
#139765=CARTESIAN_POINT ( 'NONE',  ( -17.14385361876520264, -23.59649016807271593, 143.1750000027311671 ) ) ;
#139837=CARTESIAN_POINT ( 'NONE',  ( -28.82186960331499037, 2.428612866367529932E-14, 146.0000000000000000 ) ) ;
#139914=ORIENTED_EDGE ( 'NONE', *, *, #68656, .T. ) ;
#139931=FACE_BOUND ( 'NONE', #52667, .T. ) ;
#140091=CARTESIAN_POINT ( 'NONE',  ( 33.70061762759713986, -5.431516297171046226, 95.88384366041691464 ) ) ;
#140094=EDGE_CURVE ( 'NONE', #120101, #162507, #178442, .T. ) ;
#140110=CARTESIAN_POINT ( 'NONE',  ( -31.80000000000000782, -5.180255960393304182E-15, 47.70000000000000284 ) ) ;
#140137=VECTOR ( 'NONE', #66527, 1000.000000000000114 ) ;
#140216=CARTESIAN_POINT ( 'NONE',  ( -37.11169547541891234, -4.770708601134445281, 42.23953901806350331 ) ) ;
#140247=CARTESIAN_POINT ( 'NONE',  ( 17.81289503416611453, -24.51734667627695785, 146.6999999999999886 ) ) ;
#140271=CARTESIAN_POINT ( 'NONE',  ( 28.82186960331499392, -9.364793116373510529, 147.1500000054623456 ) ) ;
#140274=AXIS2_PLACEMENT_3D ( 'NONE', #148530, #83828, #159680 ) ;
#140285=EDGE_LOOP ( 'NONE', ( #108700, #63538, #154121, #197481 ) ) ;
#140295=ORIENTED_EDGE ( 'NONE', *, *, #37951, .F. ) ;
#140317=EDGE_LOOP ( 'NONE', ( #37741, #65951 ) ) ;
#140340=AXIS2_PLACEMENT_3D ( 'NONE', #137373, #13057, #166742 ) ;
#140366=CARTESIAN_POINT ( 'NONE',  ( -22.44159573604009950, -16.30477369853688430, 143.0750000027311728 ) ) ;
#140384=VECTOR ( 'NONE', #71506, 1000.000000000000000 ) ;
#140422=CARTESIAN_POINT ( 'NONE',  ( 17.81289503416610742, 24.51734667627700404, 149.2999999999999261 ) ) ;
#140456=EDGE_CURVE ( 'NONE', #172412, #116580, #199091, .T. ) ;
#140494=CARTESIAN_POINT ( 'NONE',  ( 36.91746825000000598, -11.99521256947793546, -10.22499999726881548 ) ) ;
#140499=CARTESIAN_POINT ( 'NONE',  ( 33.84581411518096417, 5.355620490906737530, 93.73536670833321693 ) ) ;
#140510=CARTESIAN_POINT ( 'NONE',  ( 36.91746824999999887, -11.99521256947793546, -4.224999997268813701 ) ) ;
#140606=DIRECTION ( 'NONE',  ( -1.000000000000000000, -0.000000000000000000, -0.000000000000000000 ) ) ;
#140679=CARTESIAN_POINT ( 'NONE',  ( -36.91746825000001309, 11.99521256947798342, -7.224999997268814589 ) ) ;
#140732=CARTESIAN_POINT ( 'NONE',  ( 23.31738231874054534, 16.94106989632529192, 145.4500000054623854 ) ) ;
#140742=AXIS2_PLACEMENT_3D ( 'NONE', #131322, #24168, #117155 ) ;
#140744=CARTESIAN_POINT ( 'NONE',  ( -30.73962218707678318, -22.33364281372842441, -7.802157773949823572 ) ) ;
#140767=CARTESIAN_POINT ( 'NONE',  ( -27.73933785331498925, 9.013057229001089965, 140.7750000027311899 ) ) ;
#140772=CARTESIAN_POINT ( 'NONE',  ( 8.571926809382597767, 26.38167802310806209, 140.2750000027311899 ) ) ;
#140803=ORIENTED_EDGE ( 'NONE', *, *, #128488, .F. ) ;
#140842=CARTESIAN_POINT ( 'NONE',  ( -27.73933785331498925, 2.428612866367529932E-14, 147.3750000027311842 ) ) ;
#140881=CARTESIAN_POINT ( 'NONE',  ( -38.00000000000000711, 2.428612866367529932E-14, -8.000000000000000000 ) ) ;
#140921=EDGE_LOOP ( 'NONE', ( #191272, #5402, #84598, #157706 ) ) ;
#140986=CIRCLE ( 'NONE', #21628, 2.649999999999999467 ) ;
#141095=CARTESIAN_POINT ( 'NONE',  ( 33.71409597518591283, -4.151718627496498115, 98.62556914322648538 ) ) ;
#141128=CARTESIAN_POINT ( 'NONE',  ( -22.81625015709510507, 31.40387420917330275, -2.924999997268813434 ) ) ;
#141149=AXIS2_PLACEMENT_3D ( 'NONE', #139214, #31052, #186743 ) ;
#141203=DIRECTION ( 'NONE',  ( 0.000000000000000000, 0.000000000000000000, 1.000000000000000000 ) ) ;
#141217=CARTESIAN_POINT ( 'NONE',  ( -36.76875311564131721, -5.017346702420296900, 47.26027925686760511 ) ) ;
#141232=ORIENTED_EDGE ( 'NONE', *, *, #80827, .F. ) ;
#141247=CARTESIAN_POINT ( 'NONE',  ( 1.993301997531345292E-15, -30.30510711980685912, 148.5000000000000000 ) ) ;
#141270=CARTESIAN_POINT ( 'NONE',  ( 28.82186960331499392, -9.364793116373510529, 139.1500000054623456 ) ) ;
#141291=CARTESIAN_POINT ( 'NONE',  ( -23.31738231874055245, -16.94106989632524574, 142.1999999999999886 ) ) ;
#141313=CARTESIAN_POINT ( 'NONE',  ( 32.00000000000000000, -5.510910596163089556E-15, 39.49999999999996447 ) ) ;
#141364=CARTESIAN_POINT ( 'NONE',  ( -22.44159573604010305, 16.30477369853692338, 144.6750000027311671 ) ) ;
#141418=AXIS2_PLACEMENT_3D ( 'NONE', #33375, #187084, #21183 ) ;
#141444=DIRECTION ( 'NONE',  ( -0.000000000000000000, -0.000000000000000000, -1.000000000000000000 ) ) ;
#141446=CIRCLE ( 'NONE', #15454, 5.500000000001017852 ) ;
#141459=( BOUNDED_CURVE ( )  B_SPLINE_CURVE ( 2, ( #30433, #61745, #198292, #41639, #121437, #135641, #168927, #59769, #92080, #14262, #180170 ),
 .UNSPECIFIED., .F., .F. ) 
 B_SPLINE_CURVE_WITH_KNOTS ( ( 3, 2, 2, 2, 2, 3 ),
 ( 0.5000000000000004441, 0.5200000000000004619, 0.5400000000000004796, 0.5600000000000006084, 0.5800000000000005151, 0.6000000000000005329 ),
 .UNSPECIFIED. ) 
 CURVE ( )  GEOMETRIC_REPRESENTATION_ITEM ( )  RATIONAL_B_SPLINE_CURVE ( ( 0.9999999999999988898, 0.9510565162951546414, 1.000000000000000000, 0.9510565162951535312, 1.000000000000000000, 0.9510565162951535312, 1.000000000000000000, 0.9510565162951535312, 1.000000000000000000, 0.9510565162951521989, 1.000000000000001332 ) ) 
 REPRESENTATION_ITEM ( '' )  );
#141481=EDGE_CURVE ( 'NONE', #175318, #11483, #156570, .T. ) ;
#141491=CARTESIAN_POINT ( 'NONE',  ( 36.91746824999999177, 2.880721459617395097E-14, -3.624999997268813168 ) ) ;
#141508=CARTESIAN_POINT ( 'NONE',  ( 36.91746824999999177, 2.880721459617395097E-14, -6.124999997268813168 ) ) ;
#141537=CARTESIAN_POINT ( 'NONE',  ( -37.87393738558670009, 1.964790904463869577E-14, 2.000000000000000000 ) ) ;
#141547=CYLINDRICAL_SURFACE ( 'NONE', #92173, 37.99626262588765968 ) ;
#141678=CARTESIAN_POINT ( 'NONE',  ( 29.86685920354754842, -21.69954338932559068, -10.32499999726881335 ) ) ;
#141761=CARTESIAN_POINT ( 'NONE',  ( 8.571926809382597767, 26.38167802310806209, 148.7750000027311899 ) ) ;
#141765=CARTESIAN_POINT ( 'NONE',  ( -22.44159573604009950, -16.30477369853688430, 141.0750000027311728 ) ) ;
#141788=EDGE_CURVE ( 'NONE', #108375, #103711, #95743, .T. ) ;
#141815=EDGE_CURVE ( 'NONE', #147006, #199732, #150379, .T. ) ;
#141830=VECTOR ( 'NONE', #69525, 1000.000000000000000 ) ;
#141833=CARTESIAN_POINT ( 'NONE',  ( 8.571926809382597767, 26.38167802310806209, 142.7750000027311899 ) ) ;
#141853=CARTESIAN_POINT ( 'NONE',  ( 8.906447517083057264, -27.41122689804191026, 144.8500000054623911 ) ) ;
#141973=AXIS2_PLACEMENT_3D ( 'NONE', #101320, #163009, #137640 ) ;
#141993=CARTESIAN_POINT ( 'NONE',  ( 29.86685920354754842, -21.69954338932559068, -1.824999997268813345 ) ) ;
#142081=CARTESIAN_POINT ( 'NONE',  ( 33.75684350552030821, -3.359699206722003062, 99.36933870599243335 ) ) ;
#142160=ORIENTED_EDGE ( 'NONE', *, *, #111650, .T. ) ;
#142236=CARTESIAN_POINT ( 'NONE',  ( -8.906447517083053711, -27.41122689804191026, 148.4000000000000057 ) ) ;
#142259=CARTESIAN_POINT ( 'NONE',  ( 27.73933785331498214, 9.013057229001095294, 147.9750000027311501 ) ) ;
#142353=CARTESIAN_POINT ( 'NONE',  ( -27.73933785331498925, -9.013057229001049109, 144.9750000027312069 ) ) ;
#142366=EDGE_CURVE ( 'NONE', #108481, #26617, #166228, .T. ) ;
#142374=CARTESIAN_POINT ( 'NONE',  ( -11.74149087413295511, 36.13659316521247433, -6.402157773949824104 ) ) ;
#142403=EDGE_LOOP ( 'NONE', ( #52806, #6646 ) ) ;
#142462=EDGE_CURVE ( 'NONE', #57160, #155489, #194782, .T. ) ;
#142479=CARTESIAN_POINT ( 'NONE',  ( -22.81625015709510507, 31.40387420917330275, -6.924999997268812990 ) ) ;
#142480=CARTESIAN_POINT ( 'NONE',  ( -33.68482864984028424, 4.779698632210292786, 97.74495643025990432 ) ) ;
#142504=VERTEX_POINT ( 'NONE', #147269 ) ;
#142532=CARTESIAN_POINT ( 'NONE',  ( 34.51183469268315207, -7.447092774749549449, 43.98515247788456151 ) ) ;
#142561=LINE ( 'NONE', #6033, #198462 ) ;
#142591=DIRECTION ( 'NONE',  ( 0.000000000000000000, 0.000000000000000000, -1.000000000000000000 ) ) ;
#142600=EDGE_CURVE ( 'NONE', #97477, #26617, #22926, .T. ) ;
#142668=CARTESIAN_POINT ( 'NONE',  ( -11.40812507854754720, -35.11059874428192273, -10.72499999726881548 ) ) ;
#142681=ORIENTED_EDGE ( 'NONE', *, *, #32687, .T. ) ;
#142724=FACE_OUTER_BOUND ( 'NONE', #59642, .T. ) ;
#142731=MANIFOLD_SOLID_BREP ( 'Cavity2', #4555 ) ;
#142754=CARTESIAN_POINT ( 'NONE',  ( 8.571926809382603096, -26.38167802310801235, 141.4750000027312069 ) ) ;
#142825=CARTESIAN_POINT ( 'NONE',  ( 17.14385361876520264, 23.59649016807275856, 144.6750000027311671 ) ) ;
#142899=CARTESIAN_POINT ( 'NONE',  ( -6.020228577223754586E-15, 39.95556452105416412, -2.249999994537625891 ) ) ;
#142950=ADVANCED_FACE ( 'NONE', ( #45490 ), #69607, .T. ) ;
#142983=CARTESIAN_POINT ( 'NONE',  ( -11.40812507854754720, -35.11059874428192273, -4.224999997268813701 ) ) ;
#143019=DIRECTION ( 'NONE',  ( -1.000000000000000000, -0.000000000000000000, -3.709348145883536076E-20 ) ) ;
#143025=B_SPLINE_CURVE_WITH_KNOTS ( 'NONE', 3,
 ( #112737, #143069, #109762, #63258, #144073, #172436, #159233, #155278, #96565, #142081, #78415, #141095, #127901, #81384, #82385, #5554, #3567, #140091, #94588, #186635, #67233, #126905, #174430, #188611, #171446, #20728, #1583, #4548, #32933, #111752, #49097, #17768, #2582, #64262, #125928, #158253, #187627, #170447, #66241, #110754 ),
 .UNSPECIFIED., .F., .F.,
 ( 4, 2, 2, 2, 2, 2, 2, 2, 2, 2, 2, 2, 2, 2, 2, 2, 2, 2, 2, 4 ),
 ( 0.02158449572284441148, 0.02266158837400314083, 0.02373868102516187018, 0.02427722735074124005, 0.02481577367632061340, 0.02589286632747935663, 0.02696995897863810332, 0.02804705162979684654, 0.02912414428095558977, 0.02966269060653496312, 0.03020123693211433646, 0.03127832958327311785, 0.03235542223443189924, 0.03343251488559068757, 0.03450960753674947590, 0.03558670018790825729, 0.03612524651348765492, 0.03666379283906703868, 0.03774088549022582006, 0.03881797814138458758 ),
 .UNSPECIFIED. ) ;
#143069=CARTESIAN_POINT ( 'NONE',  ( 33.85315667487628843, -0.3599896029658087859, 100.5000000000010374 ) ) ;
#143103=CARTESIAN_POINT ( 'NONE',  ( -11.40812507854754720, -35.11059874428192273, -6.224999997268812812 ) ) ;
#143194=CARTESIAN_POINT ( 'NONE',  ( 32.58888545195122077, -1.708444646721647420, 87.69298048441147841 ) ) ;
#143223=CARTESIAN_POINT ( 'NONE',  ( -8.906447517083060816, 27.41122689804195645, 149.5999999999999943 ) ) ;
#143244=CARTESIAN_POINT ( 'NONE',  ( 27.73933785331498925, -9.013057229001033122, 147.7750000027311899 ) ) ;
#143264=CARTESIAN_POINT ( 'NONE',  ( -32.64453336272028139, 2.028832619897439204E-14, 87.50000000000000000 ) ) ;
#143352=DIRECTION ( 'NONE',  ( 0.000000000000000000, 0.000000000000000000, -1.000000000000000000 ) ) ;
#143376=VECTOR ( 'NONE', #72906, 1000.000000000000000 ) ;
#143459=CARTESIAN_POINT ( 'NONE',  ( 29.86685920354754487, 21.69954338932564752, -7.424999997268813878 ) ) ;
#143460=CARTESIAN_POINT ( 'NONE',  ( -33.68458106784984096, 5.328653173427194467, 96.40873914273848300 ) ) ;
#143514=CARTESIAN_POINT ( 'NONE',  ( 34.46950536905809059, -7.498137530812974738, 44.48224578455059941 ) ) ;
#143533=FACE_OUTER_BOUND ( 'NONE', #37503, .T. ) ;
#143675=ORIENTED_EDGE ( 'NONE', *, *, #32497, .F. ) ;
#143712=CARTESIAN_POINT ( 'NONE',  ( -33.68444218968560477, -5.327119193238887718, 96.41491933019771920 ) ) ;
#143718=DIRECTION ( 'NONE',  ( 1.000000000000000000, 0.000000000000000000, 0.000000000000000000 ) ) ;
#143745=LINE ( 'NONE', #187300, #69897 ) ;
#143750=CARTESIAN_POINT ( 'NONE',  ( 27.73933785331498925, -9.013057229001033122, 139.7750000027311899 ) ) ;
#143783=EDGE_LOOP ( 'NONE', ( #151113, #41837, #164104, #7104 ) ) ;
#143822=CARTESIAN_POINT ( 'NONE',  ( -27.73933785331498925, 2.428612866367529932E-14, 145.3750000027311842 ) ) ;
#143826=FACE_OUTER_BOUND ( 'NONE', #41664, .T. ) ;
#143900=CARTESIAN_POINT ( 'NONE',  ( -38.00000000000000711, 2.428612866367529932E-14, -5.749999994537626336 ) ) ;
#143952=CARTESIAN_POINT ( 'NONE',  ( -5.950531402560715689E-15, 38.81732327939063509, -5.624999997268812280 ) ) ;
#143970=ORIENTED_EDGE ( 'NONE', *, *, #6551, .F. ) ;
#143985=CARTESIAN_POINT ( 'NONE',  ( 22.81625015709510151, -31.40387420917324590, -1.924999997268813212 ) ) ;
#144048=ORIENTED_EDGE ( 'NONE', *, *, #189746, .F. ) ;
#144073=CARTESIAN_POINT ( 'NONE',  ( 33.82551795724113930, -1.774401534882015241, 100.2184796937738582 ) ) ;
#144106=CARTESIAN_POINT ( 'NONE',  ( -36.91746825000001309, 11.99521256947798342, -8.724999997268813701 ) ) ;
#144226=CARTESIAN_POINT ( 'NONE',  ( -28.82186960331499392, -9.364793116373526516, 148.0999999999999943 ) ) ;
#144247=CARTESIAN_POINT ( 'NONE',  ( 8.906447517083050158, 27.41122689804195645, 141.6500000054623740 ) ) ;
#144273=CARTESIAN_POINT ( 'NONE',  ( 28.82186960331496905, -9.364793116373544279, 147.1500000054623456 ) ) ;
#144288=EDGE_LOOP ( 'NONE', ( #158516, #90549, #84783, #144048 ) ) ;
#144300=CIRCLE ( 'NONE', #137822, 35.99626262588765258 ) ;
#144339=CARTESIAN_POINT ( 'NONE',  ( -17.14385361876520975, 23.59649016807275856, 140.5750000027311444 ) ) ;
#144461=CARTESIAN_POINT ( 'NONE',  ( 36.91746824999999177, 2.880721459617395097E-14, -5.624999997268813168 ) ) ;
#144517=CARTESIAN_POINT ( 'NONE',  ( 34.72618186072386948, -2.417897188208078418, 52.10384489098236571 ) ) ;
#144541=CARTESIAN_POINT ( 'NONE',  ( -23.48298174826590667, 32.32155151706776053, -4.302157773949822683 ) ) ;
#144602=AXIS2_PLACEMENT_3D ( 'NONE', #135316, #180829, #101970 ) ;
#144657=CARTESIAN_POINT ( 'NONE',  ( 23.48298174826590667, -32.32155151706770368, -5.302157773949822683 ) ) ;
#144660=CARTESIAN_POINT ( 'NONE',  ( 36.91746824999999177, 2.880721459617395097E-14, -10.12499999726881583 ) ) ;
#144706=EDGE_CURVE ( 'NONE', #56681, #153137, #150228, .T. ) ;
#144713=DIRECTION ( 'NONE',  ( 0.000000000000000000, 0.000000000000000000, 1.000000000000000000 ) ) ;
#144744=( BOUNDED_CURVE ( )  B_SPLINE_CURVE ( 2, ( #111224, #160716, #19230, #113207, #82863, #172916, #36361, #144541, #6026, #53535, #158714 ),
 .UNSPECIFIED., .F., .T. ) 
 B_SPLINE_CURVE_WITH_KNOTS ( ( 3, 2, 2, 2, 2, 3 ),
 ( 0.5000000000000000000, 0.5200000000000000178, 0.5400000000000000355, 0.5600000000000001643, 0.5800000000000001821, 0.6000000000000000888 ),
 .UNSPECIFIED. ) 
 CURVE ( )  GEOMETRIC_REPRESENTATION_ITEM ( )  RATIONAL_B_SPLINE_CURVE ( ( 1.000000000000000000, 0.9510565162951535312, 1.000000000000000000, 0.9510565162951535312, 1.000000000000000000, 0.9510565162951535312, 1.000000000000000000, 0.9510565162951535312, 1.000000000000000000, 0.9510565162951533091, 1.000000000000000222 ) ) 
 REPRESENTATION_ITEM ( '' )  );
#144747=CARTESIAN_POINT ( 'NONE',  ( -27.73933785331498925, 2.428612866367529932E-14, 143.3750000027311842 ) ) ;
#144819=CARTESIAN_POINT ( 'NONE',  ( 17.14385361876520264, 23.59649016807275856, 146.6750000027311671 ) ) ;
#144896=CARTESIAN_POINT ( 'NONE',  ( -11.74264578624800670, 36.14014761921585972, -6.149999994537627579 ) ) ;
#144931=CARTESIAN_POINT ( 'NONE',  ( 31.24420449012917089, 7.031618440654747282, 97.62038805904606420 ) ) ;
#144936=LINE ( 'NONE', #189473, #131038 ) ;
#144946=CARTESIAN_POINT ( 'NONE',  ( -11.40812507854754720, -35.11059874428192273, -6.724999997268813701 ) ) ;
#144979=CARTESIAN_POINT ( 'NONE',  ( -11.40812507854754720, -35.11059874428192273, -6.224999997268812812 ) ) ;
#144993=DIRECTION ( 'NONE',  ( 0.000000000000000000, 0.000000000000000000, -1.000000000000000000 ) ) ;
#145099=CARTESIAN_POINT ( 'NONE',  ( 29.86685920354754487, 21.69954338932564752, -9.424999997268814766 ) ) ;
#145184=CARTESIAN_POINT ( 'NONE',  ( -32.00000000000000711, -1.163414459189985801E-14, 95.00000000000000000 ) ) ;
#145190=CARTESIAN_POINT ( 'NONE',  ( 32.15403441185031141, -4.954129643790904147, 89.34785441345067625 ) ) ;
#145193=DIRECTION ( 'NONE',  ( 0.000000000000000000, -1.000000000000000000, 0.000000000000000000 ) ) ;
#145245=CARTESIAN_POINT ( 'NONE',  ( 1.993301997531345292E-15, -30.30510711980685912, 142.7500000054623683 ) ) ;
#145255=DIRECTION ( 'NONE',  ( -1.000000000000000000, 0.000000000000000000, -6.982962677686266711E-15 ) ) ;
#145272=CARTESIAN_POINT ( 'NONE',  ( 8.906447517083057264, -27.41122689804191026, 146.8500000054623627 ) ) ;
#145338=CARTESIAN_POINT ( 'NONE',  ( -22.44159573604009950, -16.30477369853688430, 139.0750000027311728 ) ) ;
#145457=CARTESIAN_POINT ( 'NONE',  ( -36.91746825000000598, 2.428612866367529932E-14, -4.624999997268814056 ) ) ;
#145458=CARTESIAN_POINT ( 'NONE',  ( -33.83483822987809475, 1.427510505796699025, 100.3145928531379241 ) ) ;
#145509=DIRECTION ( 'NONE',  ( 1.000000000000000000, 0.000000000000000000, 0.000000000000000000 ) ) ;
#145542=B_SPLINE_CURVE_WITH_KNOTS ( 'NONE', 3,
 ( #170843, #44524, #974, #78816, #29363, #169843, #167863, #90993, #75837, #122337, #45510, #31337, #30341, #91982, #153676, #15173, #5947, #19153, #64655, #51466, #188014, #83779, #36282, #143460, #130275, #94985, #142480, #97937, #159630, #67624, #80802, #157663, #160637, #4945, #126317, #145458, #3958, #129284, #49484, #111147 ),
 .UNSPECIFIED., .F., .F.,
 ( 4, 2, 2, 2, 2, 2, 2, 2, 2, 2, 2, 2, 2, 2, 2, 2, 2, 2, 2, 4 ),
 ( 0.004339806180219608206, 0.005417599276633671204, 0.006495392373047733335, 0.007034288921254771773, 0.007573185469461809344, 0.008650978565875887955, 0.009728771662289966565, 0.01080656475870404344, 0.01134546130691106366, 0.01188435785511808215, 0.01296215095153212260, 0.01403994404794616131, 0.01511773714436020176, 0.01619553024077424047, 0.01727332333718828092, 0.01835111643360232137, 0.01942890953001635834, 0.01996780607822337336, 0.02050670262643038491, 0.02158449572284441495 ),
 .UNSPECIFIED. ) ;
#145569=( BOUNDED_CURVE ( )  B_SPLINE_CURVE ( 2, ( #154912, #76076, #137752, #139725, #121584, #15413, #186268, #94224, #125572, #172075, #155905 ),
 .UNSPECIFIED., .F., .F. ) 
 B_SPLINE_CURVE_WITH_KNOTS ( ( 3, 2, 2, 2, 2, 3 ),
 ( 0.6000000000000005329, 0.6200000000000005507, 0.6400000000000005684, 0.6600000000000006972, 0.6800000000000007150, 0.7000000000000006217 ),
 .UNSPECIFIED. ) 
 CURVE ( )  GEOMETRIC_REPRESENTATION_ITEM ( )  RATIONAL_B_SPLINE_CURVE ( ( 0.9999999999999986677, 0.9510565162951548634, 1.000000000000000000, 0.9510565162951535312, 1.000000000000000000, 0.9510565162951535312, 1.000000000000000000, 0.9510565162951535312, 1.000000000000000000, 0.9510565162951518658, 1.000000000000001554 ) ) 
 REPRESENTATION_ITEM ( '' )  );
#145619=DIRECTION ( 'NONE',  ( 1.000000000000000000, 0.000000000000000000, 0.000000000000000000 ) ) ;
#145658=CARTESIAN_POINT ( 'NONE',  ( 29.86685920354754487, 21.69954338932564752, -9.924999997268812990 ) ) ;
#145662=CARTESIAN_POINT ( 'NONE',  ( 35.04522399272636335, 11.85564638482192557, -8.000000000000001776 ) ) ;
#145675=ORIENTED_EDGE ( 'NONE', *, *, #93145, .T. ) ;
#145709=CARTESIAN_POINT ( 'NONE',  ( 14.18669005401828187, -34.08280046153741694, -8.000000000000001776 ) ) ;
#145725=CARTESIAN_POINT ( 'NONE',  ( -27.73933785331498925, 2.428612866367529932E-14, 138.8750000027311842 ) ) ;
#145742=ORIENTED_EDGE ( 'NONE', *, *, #68093, .T. ) ;
#145747=CARTESIAN_POINT ( 'NONE',  ( 17.14385361876520264, 23.59649016807275856, 142.6750000027311103 ) ) ;
#145754=LINE ( 'NONE', #4242, #67083 ) ;
#145778=LINE ( 'NONE', #114437, #120903 ) ;
#145818=CARTESIAN_POINT ( 'NONE',  ( 17.14385361876520264, 23.59649016807275856, 140.6750000027311387 ) ) ;
#145894=CARTESIAN_POINT ( 'NONE',  ( 11.74264578624800315, -36.14014761921581709, -5.149999994537626691 ) ) ;
#145916=EDGE_CURVE ( 'NONE', #2296, #36039, #169531, .T. ) ;
#145931=CARTESIAN_POINT ( 'NONE',  ( 31.27056374934903715, 7.502136971886772976, 95.45648825569141138 ) ) ;
#145947=CARTESIAN_POINT ( 'NONE',  ( 29.86685920354754487, 21.69954338932564752, -3.924999997268812990 ) ) ;
#145949=CARTESIAN_POINT ( 'NONE',  ( -31.99364916731038022, -5.510910596163089556E-15, 45.00000000000000000 ) ) ;
#145977=CARTESIAN_POINT ( 'NONE',  ( 3.556970738554034288E-15, -38.81732327939057114, -4.124999997268813168 ) ) ;
#145989=ORIENTED_EDGE ( 'NONE', *, *, #105310, .F. ) ;
#146097=CARTESIAN_POINT ( 'NONE',  ( 11.40812507854754365, 35.11059874428196537, -7.224999997268813701 ) ) ;
#146215=CARTESIAN_POINT ( 'NONE',  ( -28.82186960331499392, 9.364793116373565596, 141.9000000000000057 ) ) ;
#146223=CIRCLE ( 'NONE', #55897, 2.699999999999993960 ) ;
#146239=CARTESIAN_POINT ( 'NONE',  ( -22.44159573604009950, -16.30477369853688430, 147.0750000027312012 ) ) ;
#146277=EDGE_LOOP ( 'NONE', ( #50691, #105254, #117831, #41605 ) ) ;
#146342=EDGE_CURVE ( 'NONE', #139003, #83841, #69603, .T. ) ;
#146388=CYLINDRICAL_SURFACE ( 'NONE', #62987, 35.99626262588765258 ) ;
#146452=CARTESIAN_POINT ( 'NONE',  ( 11.40812507854755253, -35.11059874428192273, -10.02499999726881441 ) ) ;
#146512=CARTESIAN_POINT ( 'NONE',  ( -31.99364916731038022, -5.186379194389042044E-15, 42.35000000000000853 ) ) ;
#146659=CARTESIAN_POINT ( 'NONE',  ( 30.03989666729983199, -21.49319168150500303, -7.999999999999994671 ) ) ;
#146744=CARTESIAN_POINT ( 'NONE',  ( -32.36699822888682831, -3.753862658156239096, 88.50241378327223174 ) ) ;
#146748=CARTESIAN_POINT ( 'NONE',  ( -5.359611314223446995E-15, 29.16686587814335496, 144.8750000027311557 ) ) ;
#146754=CARTESIAN_POINT ( 'NONE',  ( 37.99626262588760994, -12.34573411038917357, -4.847842220587804007 ) ) ;
#146761=( BOUNDED_CURVE ( )  B_SPLINE_CURVE ( 2, ( #68918, #146754, #53756, #54751, #86085, #178113, #128580, #52741, #98226, #8248, #115430 ),
 .UNSPECIFIED., .F., .F. ) 
 B_SPLINE_CURVE_WITH_KNOTS ( ( 3, 2, 2, 2, 2, 3 ),
 ( 0.3000000000000000999, 0.3200000000000001177, 0.3400000000000000799, 0.3600000000000000422, 0.3800000000000000044, 0.4000000000000000222 ),
 .UNSPECIFIED. ) 
 CURVE ( )  GEOMETRIC_REPRESENTATION_ITEM ( )  RATIONAL_B_SPLINE_CURVE ( ( 0.9999999999999997780, 0.9510565162951537532, 1.000000000000000000, 0.9510565162951535312, 1.000000000000000000, 0.9510565162951535312, 1.000000000000000000, 0.9510565162951535312, 1.000000000000000000, 0.9510565162951535312, 1.000000000000000000 ) ) 
 REPRESENTATION_ITEM ( '' )  );
#146822=ORIENTED_EDGE ( 'NONE', *, *, #53035, .T. ) ;
#146871=CARTESIAN_POINT ( 'NONE',  ( 28.82186960331498327, 2.781578969918950771E-14, 147.0000000000000000 ) ) ;
#146899=AXIS2_PLACEMENT_3D ( 'NONE', #129528, #191228, #114365 ) ;
#146923=LINE ( 'NONE', #26593, #69462 ) ;
#146946=CARTESIAN_POINT ( 'NONE',  ( 31.26591117326540115, 6.741338443544413472, 98.29621977100282493 ) ) ;
#146962=CARTESIAN_POINT ( 'NONE',  ( 30.00000000000000711, -4.592425496802575156E-15, 52.50000000000000000 ) ) ;
#146977=UNCERTAINTY_MEASURE_WITH_UNIT (LENGTH_MEASURE( 1.000000000000000082E-05 ), #89080, 'distance_accuracy_value', 'NONE');
#146991=CARTESIAN_POINT ( 'NONE',  ( 29.86685920354754842, -21.69954338932559068, -7.824999997268813345 ) ) ;
#146997=ADVANCED_FACE ( 'NONE', ( #13582 ), #196641, .T. ) ;
#147006=VERTEX_POINT ( 'NONE', #41953 ) ;
#147075=CARTESIAN_POINT ( 'NONE',  ( 31.99364916731003916, -5.186379194429593439E-15, 47.65000000000021885 ) ) ;
#147080=DIRECTION ( 'NONE',  ( -1.000000000000000000, 0.000000000000000000, -3.709348145883536076E-20 ) ) ;
#147083=CARTESIAN_POINT ( 'NONE',  ( 37.99626262588765258, 2.893932880411085066E-14, 2.000000000000000000 ) ) ;
#147118=CARTESIAN_POINT ( 'NONE',  ( 30.74264578624799782, 22.33583958711400541, -2.799999999999999822 ) ) ;
#147235=CARTESIAN_POINT ( 'NONE',  ( -5.429308488886486681E-15, 30.30510711980690175, 143.4999999999999432 ) ) ;
#147237=CARTESIAN_POINT ( 'NONE',  ( -8.906447517083060816, 27.41122689804195645, 143.8500000054623911 ) ) ;
#147269=CARTESIAN_POINT ( 'NONE',  ( -28.82186960331499037, 2.428612866367529932E-14, 138.2500000054623683 ) ) ;
#147354=CARTESIAN_POINT ( 'NONE',  ( -8.571926809382601320, -26.38167802310801591, 139.2750000027311899 ) ) ;
#147407=AXIS2_PLACEMENT_3D ( 'NONE', #47780, #185289, #46781 ) ;
#147446=CARTESIAN_POINT ( 'NONE',  ( -12.36037464099328176, 35.70181166999180533, -7.999999999999996447 ) ) ;
#147544=ORIENTED_EDGE ( 'NONE', *, *, #79191, .F. ) ;
#147696=VERTEX_POINT ( 'NONE', #182448 ) ;
#147719=CARTESIAN_POINT ( 'NONE',  ( -30.00000000000000000, -1.163414459189985801E-14, 95.00000000000000000 ) ) ;
#147732=FACE_OUTER_BOUND ( 'NONE', #62943, .T. ) ;
#147744=CARTESIAN_POINT ( 'NONE',  ( -11.40812507854755609, 35.11059874428196537, -1.524999997268813301 ) ) ;
#147770=CARTESIAN_POINT ( 'NONE',  ( -8.571926809382608425, 26.38167802310805854, 142.9750000027312069 ) ) ;
#147821=VECTOR ( 'NONE', #198093, 1000.000000000000000 ) ;
#147846=CARTESIAN_POINT ( 'NONE',  ( 27.73933785331498925, -9.013057229001034898, 147.7750000027311899 ) ) ;
#147885=DIRECTION ( 'NONE',  ( 0.000000000000000000, 1.224646799147330774E-16, 1.000000000000000000 ) ) ;
#147919=CARTESIAN_POINT ( 'NONE',  ( -38.00000000000001421, -12.34694845685042708, -9.649999994537626691 ) ) ;
#147929=DIRECTION ( 'NONE',  ( -0.000000000000000000, -1.000000000000000000, 0.000000000000000000 ) ) ;
#147955=CARTESIAN_POINT ( 'NONE',  ( 31.65987002919143478, 2.420393710425480904, 102.1029948765363713 ) ) ;
#148076=DIRECTION ( 'NONE',  ( 0.000000000000000000, 0.000000000000000000, 1.000000000000000000 ) ) ;
#148081=FACE_OUTER_BOUND ( 'NONE', #185131, .T. ) ;
#148122=CARTESIAN_POINT ( 'NONE',  ( 30.74264578624800137, -22.33583958711395212, -7.200000000000001066 ) ) ;
#148238=CARTESIAN_POINT ( 'NONE',  ( 1.993301997531345292E-15, -30.30510711980685912, 144.4999999999999432 ) ) ;
#148442=DIRECTION ( 'NONE',  ( 1.000000000000000000, 0.000000000000000000, -0.000000000000000000 ) ) ;
#148476=CARTESIAN_POINT ( 'NONE',  ( -27.73933785331498925, 9.013057229001089965, 149.2750000027311330 ) ) ;
#148499=CARTESIAN_POINT ( 'NONE',  ( -34.78522506798723413, -4.592425496937305498E-15, 52.50000000000000000 ) ) ;
#148530=CARTESIAN_POINT ( 'NONE',  ( -3.573655867282028392E-15, 2.428612866367529932E-14, 139.9999999999999716 ) ) ;
#148608=CARTESIAN_POINT ( 'NONE',  ( 30.73962218707677607, 22.33364281372847060, -2.802157773949823127 ) ) ;
#148652=EDGE_CURVE ( 'NONE', #199732, #89527, #40606, .T. ) ;
#148728=CARTESIAN_POINT ( 'NONE',  ( -34.35275354914907098, -2.907972467998146016, 90.32821402270536737 ) ) ;
#148730=CARTESIAN_POINT ( 'NONE',  ( -14.13632694027962167, -34.57669575970837883, -7.999999999999994671 ) ) ;
#148742=CARTESIAN_POINT ( 'NONE',  ( -36.91746825000000598, 2.428612866367529932E-14, -3.124999997268813168 ) ) ;
#148763=CARTESIAN_POINT ( 'NONE',  ( -32.64453336272028849, -0.4913453444576352802, 87.50000000000004263 ) ) ;
#148767=CARTESIAN_POINT ( 'NONE',  ( -17.14385361876520264, -23.59649016807271593, 141.6750000027311103 ) ) ;
#148772=PRESENTATION_STYLE_ASSIGNMENT (( #104255 ) ) ;
#148773=CARTESIAN_POINT ( 'NONE',  ( 23.48298174826590667, -32.32155151706770368, -7.047842220587802409 ) ) ;
#148800=CARTESIAN_POINT ( 'NONE',  ( -3.573655867282028392E-15, 2.428612866367529932E-14, 150.0000000000000000 ) ) ;
#148916=CARTESIAN_POINT ( 'NONE',  ( 36.91746824999999887, 11.99521256947799053, -2.024999997268813523 ) ) ;
#148953=CARTESIAN_POINT ( 'NONE',  ( 32.23033374730683676, 4.573250637950146746, 89.03582022910541127 ) ) ;
#148958=DIRECTION ( 'NONE',  ( -7.855351589328939542E-15, 0.000000000000000000, 1.000000000000000000 ) ) ;
#148970=CARTESIAN_POINT ( 'NONE',  ( -34.45224964297660364, -5.970420695714335757, 49.56603145559585499 ) ) ;
#148980=FACE_OUTER_BOUND ( 'NONE', #153973, .T. ) ;
#148999=CARTESIAN_POINT ( 'NONE',  ( 36.91746824999999177, 2.880721459617395097E-14, -7.624999997268813168 ) ) ;
#149012=ORIENTED_EDGE ( 'NONE', *, *, #177696, .F. ) ;
#149082=CARTESIAN_POINT ( 'NONE',  ( -31.56642711641982757, 3.769985069464013350, 101.5021612967808409 ) ) ;
#149083=CARTESIAN_POINT ( 'NONE',  ( 28.82186960331491221, -9.364793116373624215, 146.8999999999999773 ) ) ;
#149123=CARTESIAN_POINT ( 'NONE',  ( 3.766062262543149401E-15, -39.95556452105413570, -5.500000000000000000 ) ) ;
#149178=EDGE_CURVE ( 'NONE', #14250, #15991, #63242, .T. ) ;
#149241=CARTESIAN_POINT ( 'NONE',  ( 23.31738231874054890, -16.94106989632523508, 140.7999999999999829 ) ) ;
#149243=CARTESIAN_POINT ( 'NONE',  ( -28.82186960331489445, 9.364793116373697046, 144.1500000054623456 ) ) ;
#149437=FACE_BOUND ( 'NONE', #167555, .T. ) ;
#149456=AXIS2_PLACEMENT_3D ( 'NONE', #171946, #80914, #173949 ) ;
#149457=FACE_OUTER_BOUND ( 'NONE', #21407, .T. ) ;
#149467=CARTESIAN_POINT ( 'NONE',  ( 29.86685920354754487, 21.69954338932564752, -9.424999997268814766 ) ) ;
#149473=CYLINDRICAL_SURFACE ( 'NONE', #138138, 7.500000000000007105 ) ;
#149523=EDGE_CURVE ( 'NONE', #168659, #137596, #57868, .T. ) ;
#149570=CARTESIAN_POINT ( 'NONE',  ( 30.73962218707677962, -22.33364281372841376, -3.202157773949823039 ) ) ;
#149591=EDGE_CURVE ( 'NONE', #97477, #77271, #108419, .T. ) ;
#149638=ORIENTED_EDGE ( 'NONE', *, *, #179710, .F. ) ;
#149706=ORIENTED_EDGE ( 'NONE', *, *, #151158, .T. ) ;
#149714=CARTESIAN_POINT ( 'NONE',  ( 36.91746825000000598, -11.99521256947793546, -2.224999997268813701 ) ) ;
#149721=CARTESIAN_POINT ( 'NONE',  ( -26.85942494856799101, -26.31850930613038742, -8.000000000000003553 ) ) ;
#149758=CARTESIAN_POINT ( 'NONE',  ( -5.359611314223446995E-15, 29.16686587814335496, 140.8750000027311842 ) ) ;
#149764=( NAMED_UNIT ( * ) SI_UNIT ( $, .STERADIAN. ) SOLID_ANGLE_UNIT ( ) );
#149903=CARTESIAN_POINT ( 'NONE',  ( 22.81625015709510151, -31.40387420917324590, -2.424999997268812546 ) ) ;
#149940=AXIS2_PLACEMENT_3D ( 'NONE', #171088, #187277, #126558 ) ;
#149985=DIRECTION ( 'NONE',  ( -1.000000000000000000, -0.000000000000000000, -3.709348145883536076E-20 ) ) ;
#149990=CARTESIAN_POINT ( 'NONE',  ( -37.19778934971984796, 4.370295695334256436, 41.64163531972152299 ) ) ;
#150002=CARTESIAN_POINT ( 'NONE',  ( -17.14385361876520264, -23.59649016807271593, 147.1750000027311671 ) ) ;
#150037=AXIS2_PLACEMENT_3D ( 'NONE', #82881, #160734, #55558 ) ;
#150072=CARTESIAN_POINT ( 'NONE',  ( 28.82186960331498327, 2.428612866367529932E-14, 139.9999999999999716 ) ) ;
#150121=CARTESIAN_POINT ( 'NONE',  ( 37.99999999999999289, 2.893978650043524126E-14, -5.000000000000000000 ) ) ;
#150127=DIRECTION ( 'NONE',  ( 0.000000000000000000, 0.000000000000000000, 1.000000000000000000 ) ) ;
#150133=VECTOR ( 'NONE', #23131, 1000.000000000000114 ) ;
#150211=CARTESIAN_POINT ( 'NONE',  ( -32.00000000000000000, -1.163414459189985801E-14, 95.00000000000000000 ) ) ;
#150228=CIRCLE ( 'NONE', #153367, 28.82186960331498682 ) ;
#150246=CARTESIAN_POINT ( 'NONE',  ( 23.31738231874054534, 16.94106989632529192, 147.4500000054623854 ) ) ;
#150248=VECTOR ( 'NONE', #71878, 1000.000000000000000 ) ;
#150379=LINE ( 'NONE', #11876, #53183 ) ;
#150436=CARTESIAN_POINT ( 'NONE',  ( -23.31738231874055600, 16.94106989632528837, 145.7999999999999829 ) ) ;
#150449=CARTESIAN_POINT ( 'NONE',  ( 14.47172084996136121, 34.43943601750907391, -7.999999999999994671 ) ) ;
#150454=AXIS2_PLACEMENT_3D ( 'NONE', #6343, #99354, #147885 ) ;
#150464=ORIENTED_EDGE ( 'NONE', *, *, #19233, .F. ) ;
#150505=VECTOR ( 'NONE', #16273, 1000.000000000000000 ) ;
#150593=VERTEX_POINT ( 'NONE', #170993 ) ;
#150612=CARTESIAN_POINT ( 'NONE',  ( -23.48298174826590667, 32.32155151706776053, -4.047842220587802409 ) ) ;
#150693=ORIENTED_EDGE ( 'NONE', *, *, #65800, .F. ) ;
#150712=ORIENTED_EDGE ( 'NONE', *, *, #89344, .F. ) ;
#150720=CARTESIAN_POINT ( 'NONE',  ( -29.86685920354755552, 21.69954338932564397, -1.324999997268813345 ) ) ;
#150726=CARTESIAN_POINT ( 'NONE',  ( -37.99626262588765968, -12.34573411038913626, -1.902157773949822772 ) ) ;
#150742=CONICAL_SURFACE ( 'NONE', #176569, 38.00373040315628259, 0.06108652381980166773 ) ;
#150836=CARTESIAN_POINT ( 'NONE',  ( -3.573655867282028392E-15, 2.428612866367529932E-14, 139.9999999999999716 ) ) ;
#150851=B_SPLINE_CURVE_WITH_KNOTS ( 'NONE', 3,
 ( #148499, #196019, #10987, #119164, #25171, #179852, #197007, #162656, #195006, #178844, #9990, #70658, #86813, #41323, #193006, #131316, #71650, #180847, #103985, #181831, #133317, #166665, #8990, #54483, #56484, #118162, #132324, #43310, #102983, #100971, #165664, #26164, #28166, #194016, #55479, #117149, #33110, #46284, #108946, #168624, #77612, #169627, #45299, #182824, #14957, #75619, #44306, #61441 ),
 .UNSPECIFIED., .F., .F.,
 ( 4, 2, 2, 2, 2, 2, 2, 2, 2, 2, 2, 2, 2, 2, 2, 2, 2, 2, 2, 2, 2, 2, 2, 4 ),
 ( 0.01768515071410573999, 0.01915622216236231162, 0.01989175788649060264, 0.02062729361061889019, 0.02209836505887546876, 0.02283390078300375631, 0.02356943650713204733, 0.02504050795538863977, 0.02651157940364523569, 0.02724711512777353017, 0.02798265085190182813, 0.02945372230015839976, 0.03092479374841497486, 0.03239586519667154996, 0.03313140092079983057, 0.03386693664492811118, 0.03460247236905639873, 0.03533800809318467934, 0.03680907954144126137, 0.03754461526556955586, 0.03828015098969785035, 0.03975122243795443933, 0.04048675816208274075, 0.04122229388621103524 ),
 .UNSPECIFIED. ) ;
#150856=EDGE_CURVE ( 'NONE', #49688, #189055, #99110, .T. ) ;
#150913=CARTESIAN_POINT ( 'NONE',  ( -5.950531402560715689E-15, 38.81732327939063509, -1.624999997268813612 ) ) ;
#150926=( BOUNDED_SURFACE ( )  B_SPLINE_SURFACE ( 1, 2, ( 
 ( #130274, #148476, #164645, #7945, #26140, #87782, #10962, #57470, #192983, #84774, #177820, #191969, #88785, #68618, #69628, #131294, #54461, #24138, #39290, #100947, #166640, #62407, #45275, #106928, #46261, #90760, #198957, #123089, #107916, #168601, #44282, #30101, #91741, #735, #74620, #76594, #29122, #77588, #31099, #154435, #93749, #152443, #181807, #92747, #60424, #13929, #153436, #138270, #105940, #89782, #14934, #199953, #108922, #61418, #15929, #75596, #137275, #135309, #184775, #196982, #122097, #120116, #183788, #169601, #151467, #43285, #139259, #58448, #124077, #185778, #47265, #170602, #104954, #32092, #11973, #73638, #28142, #12956, #136286, #197962, #59432, #121105, #182799, #167625, #20886, #37050, #127059, #66395, #34078, #172592, #188766, #96718, #49248, #82544, #52219, #18916, #189759, #111906, #173594, #187778, #155430 ),
 ( #1739, #80561, #5710, #63417, #143223, #190745, #110906, #95736, #171598, #158406, #94742, #2736, #128057, #67387, #48261, #141247, #142236, #129044, #79578, #144226, #3721, #113876, #78573, #175573, #51231, #16920, #112892, #65398, #157422, #174586, #50250, #109914, #35063, #140247, #19895, #81536, #36051, #125092, #186790, #4705, #33086, #97700, #156422, #159391, #17923, #64413, #126082, #21892, #57236, #115898, #71396, #163411, #191732, #38060, #24907, #148238, #6703, #101721, #86554, #176586, #68381, #133060, #9732, #41065, #164417, #147235, #130033, #194750, #116890, #56222, #53214, #117904, #114892, #69386, #162393, #118910, #179593, #98709, #180594, #131055, #40047, #146215, #23896, #161400, #102728, #70396, #25910, #87554, #99716, #72396, #22892, #160403, #149241, #132064, #10732, #84538, #134072, #83542, #195762, #55221, #7703 ) ),
 .UNSPECIFIED., .F., .F., .T. ) 
 B_SPLINE_SURFACE_WITH_KNOTS ( ( 2, 2 ),
 ( 3, 2, 2, 2, 2, 2, 2, 2, 2, 2, 2, 2, 2, 2, 2, 2, 2, 2, 2, 2, 2, 2, 2, 2, 2, 2, 2, 2, 2, 2, 2, 2, 2, 2, 2, 2, 2, 2, 2, 2, 2, 2, 2, 2, 2, 2, 2, 2, 2, 2, 3 ),
 ( 0.000000000000000000, 1.000000000000000000 ),
 ( 0.000000000000000000, 0.02000000000000000042, 0.04000000000000000083, 0.05999999999999999778, 0.08000000000000000167, 0.1000000000000000056, 0.1199999999999999956, 0.1400000000000000133, 0.1600000000000000033, 0.1799999999999999933, 0.2000000000000000111, 0.2200000000000000011, 0.2399999999999999911, 0.2600000000000000089, 0.2800000000000000266, 0.2999999999999999889, 0.3200000000000000067, 0.3400000000000000244, 0.3599999999999999867, 0.3800000000000000044, 0.4000000000000000222, 0.4199999999999999845, 0.4400000000000000022, 0.4600000000000000200, 0.4799999999999999822, 0.5000000000000000000, 0.5200000000000000178, 0.5400000000000000355, 0.5600000000000000533, 0.5799999999999999600, 0.5999999999999999778, 0.6199999999999999956, 0.6400000000000000133, 0.6600000000000000311, 0.6800000000000000488, 0.6999999999999999556, 0.7199999999999999734, 0.7399999999999999911, 0.7600000000000000089, 0.7800000000000000266, 0.8000000000000000444, 0.8199999999999999512, 0.8399999999999999689, 0.8599999999999999867, 0.8800000000000000044, 0.9000000000000000222, 0.9200000000000000400, 0.9399999999999999467, 0.9599999999999999645, 0.9799999999999999822, 1.000000000000000000 ),
 .UNSPECIFIED. ) 
 GEOMETRIC_REPRESENTATION_ITEM ( )  RATIONAL_B_SPLINE_SURFACE ( (
 ( 1.000000000000000000, 0.9510565162951535312, 1.000000000000000000, 0.9510565162951535312, 1.000000000000000000, 0.9510565162951535312, 1.000000000000000000, 0.9510565162951535312, 1.000000000000000000, 0.9510565162951535312, 1.000000000000000000, 0.9510565162951535312, 1.000000000000000000, 0.9510565162951535312, 1.000000000000000000, 0.9510565162951535312, 1.000000000000000000, 0.9510565162951535312, 1.000000000000000000, 0.9510565162951535312, 1.000000000000000000, 0.9510565162951535312, 1.000000000000000000, 0.9510565162951535312, 1.000000000000000000, 0.9510565162951535312, 1.000000000000000000, 0.9510565162951535312, 1.000000000000000000, 0.9510565162951535312, 1.000000000000000000, 0.9510565162951535312, 1.000000000000000000, 0.9510565162951535312, 1.000000000000000000, 0.9510565162951535312, 1.000000000000000000, 0.9510565162951535312, 1.000000000000000000, 0.9510565162951535312, 1.000000000000000000, 0.9510565162951535312, 1.000000000000000000, 0.9510565162951535312, 1.000000000000000000, 0.9510565162951535312, 1.000000000000000000, 0.9510565162951535312, 1.000000000000000000, 0.9510565162951535312, 1.000000000000000000, 0.9510565162951535312, 1.000000000000000000, 0.9510565162951535312, 1.000000000000000000, 0.9510565162951535312, 1.000000000000000000, 0.9510565162951535312, 1.000000000000000000, 0.9510565162951535312, 1.000000000000000000, 0.9510565162951535312, 1.000000000000000000, 0.9510565162951535312, 1.000000000000000000, 0.9510565162951535312, 1.000000000000000000, 0.9510565162951535312, 1.000000000000000000, 0.9510565162951535312, 1.000000000000000000, 0.9510565162951535312, 1.000000000000000000, 0.9510565162951535312, 1.000000000000000000, 0.9510565162951535312, 1.000000000000000000, 0.9510565162951535312, 1.000000000000000000, 0.9510565162951535312, 1.000000000000000000, 0.9510565162951535312, 1.000000000000000000, 0.9510565162951535312, 1.000000000000000000, 0.9510565162951535312, 1.000000000000000000, 0.9510565162951535312, 1.000000000000000000, 0.9510565162951535312, 1.000000000000000000, 0.9510565162951535312, 1.000000000000000000, 0.9510565162951535312, 1.000000000000000000, 0.9510565162951535312, 1.000000000000000000, 0.9510565162951535312, 1.000000000000000000, 0.9510565162951535312, 1.000000000000000000),
 ( 1.000000000000000000, 0.9510565162951535312, 1.000000000000000000, 0.9510565162951535312, 1.000000000000000000, 0.9510565162951535312, 1.000000000000000000, 0.9510565162951535312, 1.000000000000000000, 0.9510565162951535312, 1.000000000000000000, 0.9510565162951535312, 1.000000000000000000, 0.9510565162951535312, 1.000000000000000000, 0.9510565162951535312, 1.000000000000000000, 0.9510565162951535312, 1.000000000000000000, 0.9510565162951535312, 1.000000000000000000, 0.9510565162951535312, 1.000000000000000000, 0.9510565162951535312, 1.000000000000000000, 0.9510565162951535312, 1.000000000000000000, 0.9510565162951535312, 1.000000000000000000, 0.9510565162951535312, 1.000000000000000000, 0.9510565162951535312, 1.000000000000000000, 0.9510565162951535312, 1.000000000000000000, 0.9510565162951535312, 1.000000000000000000, 0.9510565162951535312, 1.000000000000000000, 0.9510565162951535312, 1.000000000000000000, 0.9510565162951535312, 1.000000000000000000, 0.9510565162951535312, 1.000000000000000000, 0.9510565162951535312, 1.000000000000000000, 0.9510565162951535312, 1.000000000000000000, 0.9510565162951535312, 1.000000000000000000, 0.9510565162951535312, 1.000000000000000000, 0.9510565162951535312, 1.000000000000000000, 0.9510565162951535312, 1.000000000000000000, 0.9510565162951535312, 1.000000000000000000, 0.9510565162951535312, 1.000000000000000000, 0.9510565162951535312, 1.000000000000000000, 0.9510565162951535312, 1.000000000000000000, 0.9510565162951535312, 1.000000000000000000, 0.9510565162951535312, 1.000000000000000000, 0.9510565162951535312, 1.000000000000000000, 0.9510565162951535312, 1.000000000000000000, 0.9510565162951535312, 1.000000000000000000, 0.9510565162951535312, 1.000000000000000000, 0.9510565162951535312, 1.000000000000000000, 0.9510565162951535312, 1.000000000000000000, 0.9510565162951535312, 1.000000000000000000, 0.9510565162951535312, 1.000000000000000000, 0.9510565162951535312, 1.000000000000000000, 0.9510565162951535312, 1.000000000000000000, 0.9510565162951535312, 1.000000000000000000, 0.9510565162951535312, 1.000000000000000000, 0.9510565162951535312, 1.000000000000000000, 0.9510565162951535312, 1.000000000000000000, 0.9510565162951535312, 1.000000000000000000, 0.9510565162951535312, 1.000000000000000000) ) ) 
 REPRESENTATION_ITEM ( '' )  SURFACE ( )  );
#150930=ORIENTED_EDGE ( 'NONE', *, *, #12591, .T. ) ;
#151006=CARTESIAN_POINT ( 'NONE',  ( -17.14385361876520264, -23.59649016807271593, 147.1750000027311671 ) ) ;
#151011=CARTESIAN_POINT ( 'NONE',  ( -22.44159573604009950, -16.30477369853688430, 143.0750000027311728 ) ) ;
#151103=DIRECTION ( 'NONE',  ( -1.000000000000000000, 0.000000000000000000, -6.982962677686266711E-15 ) ) ;
#151113=ORIENTED_EDGE ( 'NONE', *, *, #51286, .F. ) ;
#151118=CARTESIAN_POINT ( 'NONE',  ( 23.48529157249600630, -32.32473071737749137, -1.299999999999999822 ) ) ;
#151128=CIRCLE ( 'NONE', #63916, 37.99626262588765968 ) ;
#151158=EDGE_CURVE ( 'NONE', #166090, #128112, #168186, .T. ) ;
#151171=CARTESIAN_POINT ( 'NONE',  ( 34.40392893854398437, 6.519971432731299643, 48.73974290947561627 ) ) ;
#151179=ADVANCED_FACE ( 'NONE', ( #75181 ), #76167, .F. ) ;
#151227=CARTESIAN_POINT ( 'NONE',  ( 35.99626262588764547, 2.869439944428138037E-14, -8.000000000000000000 ) ) ;
#151253=ORIENTED_EDGE ( 'NONE', *, *, #12591, .F. ) ;
#151318=DIRECTION ( 'NONE',  ( 1.000000000000000000, -0.000000000000000000, -0.000000000000000000 ) ) ;
#151367=DIRECTION ( 'NONE',  ( -1.000000000000000000, -0.000000000000000000, -0.000000000000000000 ) ) ;
#151378=APPLICATION_CONTEXT ( 'automotive_design' ) ;
#151437=LINE ( 'NONE', #186759, #89675 ) ;
#151467=CARTESIAN_POINT ( 'NONE',  ( -8.571926809382608425, 26.38167802310805854, 142.9750000027312069 ) ) ;
#151490=CARTESIAN_POINT ( 'NONE',  ( -23.31738231874055600, 16.94106989632528837, 146.0500000054623797 ) ) ;
#151597=CARTESIAN_POINT ( 'NONE',  ( 37.99626262588765258, 2.893932880411085066E-14, -3.002157773949822861 ) ) ;
#151617=CARTESIAN_POINT ( 'NONE',  ( 33.85315667487628133, 2.428612866512670557E-14, 100.5000000000010232 ) ) ;
#151705=CARTESIAN_POINT ( 'NONE',  ( 36.91746824999999887, 11.99521256947799053, -10.02499999726881086 ) ) ;
#151711=CARTESIAN_POINT ( 'NONE',  ( 23.48298174826590667, -32.32155151706770368, -1.302157773949822683 ) ) ;
#151749=LINE ( 'NONE', #182093, #182155 ) ;
#151754=( LENGTH_UNIT ( ) NAMED_UNIT ( * ) SI_UNIT ( .MILLI., .METRE. ) );
#151890=CARTESIAN_POINT ( 'NONE',  ( -11.40812507854755609, 35.11059874428196537, -1.524999997268813301 ) ) ;
#151903=EDGE_CURVE ( 'NONE', #118975, #31542, #158160, .T. ) ;
#151941=CARTESIAN_POINT ( 'NONE',  ( 36.90816834587730710, 0.7173862878750157934, 50.46507289210756397 ) ) ;
#151979=CARTESIAN_POINT ( 'NONE',  ( -17.14385361876520619, 23.59649016807275856, 148.5750000027311444 ) ) ;
#151985=CARTESIAN_POINT ( 'NONE',  ( 27.73933785331498925, -9.013057229001033122, 141.7750000027311899 ) ) ;
#152095=CARTESIAN_POINT ( 'NONE',  ( -23.48529157249600985, 32.32473071737754111, -8.300000000000000711 ) ) ;
#152332=CARTESIAN_POINT ( 'NONE',  ( -31.80000000000000782, -1.163414459189985801E-14, 95.00000000000000000 ) ) ;
#152340=EDGE_CURVE ( 'NONE', #115964, #81412, #18090, .T. ) ;
#152372=ORIENTED_EDGE ( 'NONE', *, *, #28811, .F. ) ;
#152398=DIRECTION ( 'NONE',  ( -1.000000000000000000, 0.000000000000000000, -0.000000000000000000 ) ) ;
#152412=CARTESIAN_POINT ( 'NONE',  ( -36.89607807516672722, -1.430951785632631701, 50.32279621992264396 ) ) ;
#152443=CARTESIAN_POINT ( 'NONE',  ( -27.73933785331498925, 9.013057229001089965, 145.2750000027311899 ) ) ;
#152467=CARTESIAN_POINT ( 'NONE',  ( 17.81289503416610742, 24.51734667627700404, 145.5500000054623513 ) ) ;
#152494=CARTESIAN_POINT ( 'NONE',  ( -31.80000000000000782, -1.163414459189985801E-14, 95.00000000000000000 ) ) ;
#152521=CARTESIAN_POINT ( 'NONE',  ( -31.80000000000000782, -5.510910596163089556E-15, 45.00000000000000000 ) ) ;
#152525=ADVANCED_FACE ( 'NONE', ( #38813 ), #166161, .F. ) ;
#152553=CARTESIAN_POINT ( 'NONE',  ( 1.784210473542230573E-15, -29.16686587814331588, 141.8750000027311842 ) ) ;
#152679=CARTESIAN_POINT ( 'NONE',  ( -29.86685920354755197, -21.69954338932560134, -2.424999997268813434 ) ) ;
#152697=CARTESIAN_POINT ( 'NONE',  ( -22.81625015709509441, -31.40387420917324590, -4.824999997268813345 ) ) ;
#152719=CARTESIAN_POINT ( 'NONE',  ( -31.69386653422660061, -1.706804019390318006, 102.3073255780427075 ) ) ;
#152725=CARTESIAN_POINT ( 'NONE',  ( -22.44159573604009950, -16.30477369853688430, 139.5750000027311728 ) ) ;
#152737=EDGE_LOOP ( 'NONE', ( #108845, #164934 ) ) ;
#152783=CARTESIAN_POINT ( 'NONE',  ( -31.72709406046301339, 2.040068635034919209E-14, 102.5000000000000142 ) ) ;
#152795=CARTESIAN_POINT ( 'NONE',  ( -21.96747269023789428, 18.79906110326631463, 140.0254762022684645 ) ) ;
#152868=CARTESIAN_POINT ( 'NONE',  ( 36.91746825000000598, -11.99521256947793546, -4.224999997268812812 ) ) ;
#152948=CARTESIAN_POINT ( 'NONE',  ( -36.86581981986046230, 2.436233122106819415, 49.93429970834160514 ) ) ;
#152955=CARTESIAN_POINT ( 'NONE',  ( 1.784210473542230573E-15, -29.16686587814331588, 147.3750000027311842 ) ) ;
#152960=CARTESIAN_POINT ( 'NONE',  ( 1.784210473542230573E-15, -29.16686587814331588, 143.3750000027311557 ) ) ;
#152997=ORIENTED_EDGE ( 'NONE', *, *, #76080, .T. ) ;
#153070=CARTESIAN_POINT ( 'NONE',  ( -30.74264578624800492, -22.33583958711396278, -7.800000000000000711 ) ) ;
#153137=VERTEX_POINT ( 'NONE', #138770 ) ;
#153301=DIRECTION ( 'NONE',  ( 0.000000000000000000, 1.000000000000000000, -1.224646799147353207E-16 ) ) ;
#153316=CARTESIAN_POINT ( 'NONE',  ( -36.91746825000001309, 11.99521256947798342, -0.7249999972688133676 ) ) ;
#153367=AXIS2_PLACEMENT_3D ( 'NONE', #47243, #139238, #122076 ) ;
#153405=CARTESIAN_POINT ( 'NONE',  ( -36.90807327575559071, -0.7244114042849736368, 50.46397389534120492 ) ) ;
#153427=PLANE ( 'NONE',  #62457 ) ;
#153436=CARTESIAN_POINT ( 'NONE',  ( 8.571926809382597767, 26.38167802310806209, 144.7750000027311899 ) ) ;
#153460=CARTESIAN_POINT ( 'NONE',  ( -8.906447517083053711, -27.41122689804191026, 144.6500000054623740 ) ) ;
#153548=CARTESIAN_POINT ( 'NONE',  ( 1.784210473542230573E-15, -29.16686587814331588, 143.3750000027311557 ) ) ;
#153550=ORIENTED_EDGE ( 'NONE', *, *, #132031, .T. ) ;
#153562=DIRECTION ( 'NONE',  ( 0.000000000000000000, 0.000000000000000000, -1.000000000000000000 ) ) ;
#153564=CARTESIAN_POINT ( 'NONE',  ( -17.81289503416611808, 24.51734667627700404, 141.9500000054623570 ) ) ;
#153566=CARTESIAN_POINT ( 'NONE',  ( 38.00373040315627549, 2.428612866367529932E-14, -0.1220970790697140096 ) ) ;
#153664=ORIENTED_EDGE ( 'NONE', *, *, #53439, .T. ) ;
#153675=CARTESIAN_POINT ( 'NONE',  ( 36.91746824999999177, 2.880721459617395097E-14, -8.124999997268814056 ) ) ;
#153676=CARTESIAN_POINT ( 'NONE',  ( -33.98302989258739615, 4.936846515367097510, 92.54907045995909698 ) ) ;
#153693=CARTESIAN_POINT ( 'NONE',  ( 3.556970738554034288E-15, -38.81732327939057114, -4.624999997268814056 ) ) ;
#153717=CARTESIAN_POINT ( 'NONE',  ( -31.49170352461663214, -4.578070284816035951, 100.9457761758980325 ) ) ;
#153722=CARTESIAN_POINT ( 'NONE',  ( 27.73933785331498214, 9.013057229001095294, 140.4750000027311785 ) ) ;
#153780=CARTESIAN_POINT ( 'NONE',  ( -31.30058771566195830, 6.382914491190407880, 98.94581565101640308 ) ) ;
#153787=DIRECTION ( 'NONE',  ( -1.000000000000000000, 0.000000000000000000, 0.000000000000000000 ) ) ;
#153803=DIRECTION ( 'NONE',  ( 0.000000000000000000, 0.000000000000000000, -1.000000000000000000 ) ) ;
#153839=AXIS2_PLACEMENT_3D ( 'NONE', #58662, #28360, #198178 ) ;
#153865=CARTESIAN_POINT ( 'NONE',  ( -29.86685920354755197, -21.69954338932560134, -6.924999997268813878 ) ) ;
#153883=ORIENTED_EDGE ( 'NONE', *, *, #43390, .T. ) ;
#153958=CARTESIAN_POINT ( 'NONE',  ( -22.44159573604010305, 16.30477369853692338, 146.6750000027311671 ) ) ;
#153973=EDGE_LOOP ( 'NONE', ( #122841, #114332, #184837, #198023 ) ) ;
#153999=EDGE_CURVE ( 'NONE', #96409, #118975, #53723, .T. ) ;
#154002=ORIENTED_EDGE ( 'NONE', *, *, #116795, .F. ) ;
#154069=VERTEX_POINT ( 'NONE', #8996 ) ;
#154074=CARTESIAN_POINT ( 'NONE',  ( 3.766062262543149401E-15, -39.95556452105413570, -7.500000000000000888 ) ) ;
#154121=ORIENTED_EDGE ( 'NONE', *, *, #50509, .F. ) ;
#154125=CARTESIAN_POINT ( 'NONE',  ( 35.59978325014670730, 2.421353778481764252, 37.88472941744216627 ) ) ;
#154180=AXIS2_PLACEMENT_3D ( 'NONE', #43259, #87755, #88759 ) ;
#154405=CARTESIAN_POINT ( 'NONE',  ( -36.82872320124401710, -3.359544971329626595, 49.36946820683673565 ) ) ;
#154435=CARTESIAN_POINT ( 'NONE',  ( -27.73933785331498925, -9.013057229001049109, 145.4750000027311501 ) ) ;
#154461=CARTESIAN_POINT ( 'NONE',  ( -17.81289503416611808, 24.51734667627700404, 145.9500000054623854 ) ) ;
#154548=CARTESIAN_POINT ( 'NONE',  ( -22.44159573604009950, -16.30477369853688430, 147.0750000027312012 ) ) ;
#154561=LINE ( 'NONE', #76719, #183473 ) ;
#154563=CARTESIAN_POINT ( 'NONE',  ( 28.82186960331498327, 2.781578969918950771E-14, 141.2500000054623683 ) ) ;
#154624=CARTESIAN_POINT ( 'NONE',  ( 30.00000000000000000, -5.510910596163089556E-15, 42.35000000000000142 ) ) ;
#154673=CARTESIAN_POINT ( 'NONE',  ( -29.86685920354755197, -21.69954338932560134, -10.92499999726881299 ) ) ;
#154679=CARTESIAN_POINT ( 'NONE',  ( 33.84955102792976334, 0.7177882281432049760, 100.4649514046631680 ) ) ;
#154691=CARTESIAN_POINT ( 'NONE',  ( -36.91746825000000598, -11.99521256947794789, -7.024999997268812635 ) ) ;
#154716=CARTESIAN_POINT ( 'NONE',  ( -31.64627301717024821, -2.653341670344202097, 102.0192792579183276 ) ) ;
#154731=DIRECTION ( 'NONE',  ( 0.000000000000000000, 0.000000000000000000, 1.000000000000000000 ) ) ;
#154776=CARTESIAN_POINT ( 'NONE',  ( -32.64453336272028139, 2.028832619897439204E-14, 87.50000000000000000 ) ) ;
#154798=DIRECTION ( 'NONE',  ( 1.000000000000000000, -0.000000000000000000, -0.000000000000000000 ) ) ;
#154862=CARTESIAN_POINT ( 'NONE',  ( -11.40812507854755609, 35.11059874428196537, -5.524999997268813523 ) ) ;
#154912=CARTESIAN_POINT ( 'NONE',  ( -28.82186960331499037, 2.428612866367530248E-14, 144.0000000000000000 ) ) ;
#154931=ORIENTED_EDGE ( 'NONE', *, *, #137048, .T. ) ;
#154932=EDGE_CURVE ( 'NONE', #65515, #122026, #155460, .T. ) ;
#154951=CARTESIAN_POINT ( 'NONE',  ( 22.44159573604009594, -16.30477369853687364, 143.6750000027311671 ) ) ;
#154978=CIRCLE ( 'NONE', #9665, 28.82186960331498682 ) ;
#155004=DIRECTION ( 'NONE',  ( 1.000000000000000000, -0.000000000000000000, -0.000000000000000000 ) ) ;
#155078=CARTESIAN_POINT ( 'NONE',  ( 37.99626262588765258, 2.893932880411085066E-14, -3.002157773949822861 ) ) ;
#155268=EDGE_CURVE ( 'NONE', #99233, #24708, #161429, .T. ) ;
#155278=CARTESIAN_POINT ( 'NONE',  ( 33.78625674316657523, -2.758724085166796236, 99.76151011743465347 ) ) ;
#155296=DIRECTION ( 'NONE',  ( 0.000000000000000000, 1.224646799147373422E-16, 1.000000000000000000 ) ) ;
#155430=CARTESIAN_POINT ( 'NONE',  ( -27.73933785331498925, 2.428612866367529932E-14, 139.3750000027311842 ) ) ;
#155454=CARTESIAN_POINT ( 'NONE',  ( -23.31738231874055600, 16.94106989632528837, 148.0500000054623797 ) ) ;
#155460=LINE ( 'NONE', #80591, #95712 ) ;
#155489=VERTEX_POINT ( 'NONE', #84567 ) ;
#155538=EDGE_LOOP ( 'NONE', ( #85257, #156713 ) ) ;
#155541=CARTESIAN_POINT ( 'NONE',  ( -22.44159573604009950, -16.30477369853688430, 145.0750000027311728 ) ) ;
#155666=CARTESIAN_POINT ( 'NONE',  ( -22.81625015709510507, 31.40387420917330275, -7.424999997268812990 ) ) ;
#155672=CARTESIAN_POINT ( 'NONE',  ( 33.76801240946110028, 5.498839508946048227, 94.61983786177952993 ) ) ;
#155683=CARTESIAN_POINT ( 'NONE',  ( -29.86685920354755197, -21.69954338932560134, -4.924999997268813878 ) ) ;
#155715=CARTESIAN_POINT ( 'NONE',  ( 34.78522506798721992, 2.428612866353961525E-14, 52.50000000000000000 ) ) ;
#155743=CARTESIAN_POINT ( 'NONE',  ( 32.00000000000000000, -5.510910596163089556E-15, 45.00000000000000000 ) ) ;
#155767=CARTESIAN_POINT ( 'NONE',  ( -31.24420449012919931, 7.031618440654747282, 97.62038805904604999 ) ) ;
#155779=CARTESIAN_POINT ( 'NONE',  ( -23.31738231874055600, 16.94106989632528837, 140.0500000054623513 ) ) ;
#155852=CARTESIAN_POINT ( 'NONE',  ( 3.556970738554033499E-15, -38.81732327939057825, -6.624999997268814056 ) ) ;
#155905=CARTESIAN_POINT ( 'NONE',  ( 28.82186960331498327, 2.781578969918950771E-14, 143.0000000000000000 ) ) ;
#155942=CARTESIAN_POINT ( 'NONE',  ( 8.571926809382603096, -26.38167802310801235, 147.9750000027311785 ) ) ;
#156055=CARTESIAN_POINT ( 'NONE',  ( -30.74264578624800492, 22.33583958711400186, -8.200000000000001066 ) ) ;
#156102=ORIENTED_EDGE ( 'NONE', *, *, #119343, .F. ) ;
#156136=CIRCLE ( 'NONE', #182006, 2.649999999999999467 ) ;
#156164=EDGE_CURVE ( 'NONE', #108481, #186418, #185801, .T. ) ;
#156274=ADVANCED_FACE ( 'NONE', ( #114570, #38747 ), #82219, .F. ) ;
#156393=CARTESIAN_POINT ( 'NONE',  ( -23.31738231874055245, -16.94106989632524574, 144.1999999999999886 ) ) ;
#156422=CARTESIAN_POINT ( 'NONE',  ( -23.31738231874055600, 16.94106989632528837, 145.7999999999999829 ) ) ;
#156429=MECHANICAL_DESIGN_GEOMETRIC_PRESENTATION_REPRESENTATION('',(#117611),#49762);
#156448=CARTESIAN_POINT ( 'NONE',  ( -8.906447517083053711, -27.41122689804191026, 140.6500000054623740 ) ) ;
#156490=ORIENTED_EDGE ( 'NONE', *, *, #58712, .T. ) ;
#156518=EDGE_CURVE ( 'NONE', #139003, #26356, #105395, .T. ) ;
#156541=CARTESIAN_POINT ( 'NONE',  ( -5.359611314223446995E-15, 29.16686587814335851, 142.3750000027311557 ) ) ;
#156560=AXIS2_PLACEMENT_3D ( 'NONE', #152332, #27024, #88669 ) ;
#156562=CARTESIAN_POINT ( 'NONE',  ( 37.99626262588763126, 12.34573411038920732, -6.902157773949824104 ) ) ;
#156570=( BOUNDED_CURVE ( )  B_SPLINE_CURVE ( 2, ( #36178, #21015, #6834, #68513, #50381, #82671, #23024, #189886, #20025, #100841, #67518 ),
 .UNSPECIFIED., .F., .T. ) 
 B_SPLINE_CURVE_WITH_KNOTS ( ( 3, 2, 2, 2, 2, 3 ),
 ( 0.1000000000000000888, 0.1200000000000000927, 0.1400000000000001243, 0.1600000000000001421, 0.1800000000000001321, 0.2000000000000001776 ),
 .UNSPECIFIED. ) 
 CURVE ( )  GEOMETRIC_REPRESENTATION_ITEM ( )  RATIONAL_B_SPLINE_CURVE ( ( 0.9999999999999997780, 0.9510565162951537532, 1.000000000000000000, 0.9510565162951535312, 1.000000000000000000, 0.9510565162951535312, 1.000000000000000000, 0.9510565162951535312, 1.000000000000000000, 0.9510565162951530871, 1.000000000000000444 ) ) 
 REPRESENTATION_ITEM ( '' )  );
#156669=CARTESIAN_POINT ( 'NONE',  ( 22.81625015709509441, 31.40387420917330275, -3.324999997268812901 ) ) ;
#156687=CARTESIAN_POINT ( 'NONE',  ( 11.40812507854754365, 35.11059874428196537, -7.724999997268813701 ) ) ;
#156713=ORIENTED_EDGE ( 'NONE', *, *, #145916, .F. ) ;
#156859=CARTESIAN_POINT ( 'NONE',  ( 3.556970738554033499E-15, -38.81732327939057825, -4.624999997268814056 ) ) ;
#156945=CARTESIAN_POINT ( 'NONE',  ( 22.44159573604009594, -16.30477369853687364, 139.6750000027311955 ) ) ;
#157014=DIRECTION ( 'NONE',  ( -1.000000000000000000, -0.000000000000000000, -0.000000000000000000 ) ) ;
#157016=CARTESIAN_POINT ( 'NONE',  ( 22.44159573604009239, 16.30477369853692693, 144.5750000027311728 ) ) ;
#157062=CARTESIAN_POINT ( 'NONE',  ( -8.906447517083060816, 27.41122689804195645, 147.5999999999999943 ) ) ;
#157136=DIRECTION ( 'NONE',  ( 0.000000000000000000, 0.000000000000000000, 1.000000000000000000 ) ) ;
#157159=CARTESIAN_POINT ( 'NONE',  ( 67.00000000000000000, -5.510910596163089556E-15, 45.00000000000000000 ) ) ;
#157166=ORIENTED_EDGE ( 'NONE', *, *, #118105, .T. ) ;
#157174=DIRECTION ( 'NONE',  ( -0.06104853953485701173, -7.476289853398329258E-18, -0.9981347984218670311 ) ) ;
#157180=CARTESIAN_POINT ( 'NONE',  ( -36.91746825000000598, 11.99521256947798520, -6.724999997268813701 ) ) ;
#157224=ADVANCED_FACE ( 'NONE', ( #139931, #16611 ), #137961, .F. ) ;
#157283=EDGE_CURVE ( 'NONE', #60925, #168659, #39351, .T. ) ;
#157322=CIRCLE ( 'NONE', #105658, 2.649999999999999467 ) ;
#157394=CARTESIAN_POINT ( 'NONE',  ( 32.22964258392465808, -4.577260022299252107, 89.03854312871816035 ) ) ;
#157422=CARTESIAN_POINT ( 'NONE',  ( 23.31738231874054534, 16.94106989632529192, 147.1999999999999886 ) ) ;
#157445=CARTESIAN_POINT ( 'NONE',  ( 17.81289503416611453, -24.51734667627695785, 138.9500000054623570 ) ) ;
#157448=CIRCLE ( 'NONE', #141418, 7.500000000000000000 ) ;
#157510=CARTESIAN_POINT ( 'NONE',  ( 37.99626262588765258, 2.893932880411085066E-14, -2.747842220587803475 ) ) ;
#157537=CARTESIAN_POINT ( 'NONE',  ( -27.73933785331498925, 2.428612866367529932E-14, 146.8750000027311842 ) ) ;
#157591=AXIS2_PLACEMENT_3D ( 'NONE', #165847, #104165, #60619 ) ;
#157629=ORIENTED_EDGE ( 'NONE', *, *, #145916, .T. ) ;
#157662=CARTESIAN_POINT ( 'NONE',  ( 3.556970738554033499E-15, -38.81732327939057825, -8.124999997268814056 ) ) ;
#157663=CARTESIAN_POINT ( 'NONE',  ( -33.78659134798514430, 2.758747016945830133, 99.77194732211482631 ) ) ;
#157665=CARTESIAN_POINT ( 'NONE',  ( -37.99626262588766679, 2.428612866367529932E-14, -3.747842220587803475 ) ) ;
#157706=ORIENTED_EDGE ( 'NONE', *, *, #63840, .T. ) ;
#157717=CARTESIAN_POINT ( 'NONE',  ( 35.59965464630456466, -2.422542088861788567, 37.88523239209962412 ) ) ;
#157854=CARTESIAN_POINT ( 'NONE',  ( -3.573655867282028392E-15, 2.428612866367529932E-14, 139.9999999999999716 ) ) ;
#157904=CARTESIAN_POINT ( 'NONE',  ( 4.645199820668773683, -36.77942965383466145, -8.000000000000001776 ) ) ;
#157920=VERTEX_POINT ( 'NONE', #189447 ) ;
#157937=CARTESIAN_POINT ( 'NONE',  ( 17.14385361876520264, 23.59649016807275856, 140.1750000027311955 ) ) ;
#158008=CARTESIAN_POINT ( 'NONE',  ( 8.571926809382603096, -26.38167802310801235, 147.9750000027311785 ) ) ;
#158055=CARTESIAN_POINT ( 'NONE',  ( 30.00000000000000000, -40.00099999999999767, 37.49999999999999289 ) ) ;
#158083=CARTESIAN_POINT ( 'NONE',  ( 11.74264578624800315, -36.14014761921581709, -3.149999994537626247 ) ) ;
#158132=CARTESIAN_POINT ( 'NONE',  ( -30.00000000000000000, -4.592425496802575156E-15, 52.50000000000000000 ) ) ;
#158152=ORIENTED_EDGE ( 'NONE', *, *, #151158, .F. ) ;
#158160=LINE ( 'NONE', #37808, #182774 ) ;
#158166=CARTESIAN_POINT ( 'NONE',  ( -29.86685920354755552, 21.69954338932564397, -0.8249999972688133454 ) ) ;
#158172=EDGE_CURVE ( 'NONE', #153137, #176832, #146923, .T. ) ;
#158253=CARTESIAN_POINT ( 'NONE',  ( 34.46475727851696291, -1.773375775694352674, 89.78131888620558243 ) ) ;
#158287=CARTESIAN_POINT ( 'NONE',  ( 3.556970738554033499E-15, -38.81732327939057825, -6.124999997268812280 ) ) ;
#158300=AXIS2_PLACEMENT_3D ( 'NONE', #95601, #18782, #80428 ) ;
#158377=CARTESIAN_POINT ( 'NONE',  ( 31.23717829866982498, -7.254840157072012907, 96.91794063280339344 ) ) ;
#158380=CARTESIAN_POINT ( 'NONE',  ( -31.80000000000000782, -1.163414459189985801E-14, 92.30000000000001137 ) ) ;
#158406=CARTESIAN_POINT ( 'NONE',  ( 28.82186960331498327, 9.364793116373570925, 149.0999999999999943 ) ) ;
#158428=CARTESIAN_POINT ( 'NONE',  ( -23.31738231874055245, -16.94106989632524574, 138.4500000054623570 ) ) ;
#158516=ORIENTED_EDGE ( 'NONE', *, *, #69017, .T. ) ;
#158539=CARTESIAN_POINT ( 'NONE',  ( 36.95458794302616212, -5.320992724678918151, 43.56214547691708816 ) ) ;
#158637=CARTESIAN_POINT ( 'NONE',  ( 11.40812507854755253, -35.11059874428192273, -4.024999997268814411 ) ) ;
#158692=CARTESIAN_POINT ( 'NONE',  ( 34.74703293042576746, -1.945922946419409216, 52.24735972161444408 ) ) ;
#158714=CARTESIAN_POINT ( 'NONE',  ( -37.99626262588766679, 2.428612866367529932E-14, -4.002157773949823749 ) ) ;
#158766=EDGE_CURVE ( 'NONE', #175318, #175994, #170053, .T. ) ;
#158879=CARTESIAN_POINT ( 'NONE',  ( -33.82551795724113930, -1.774401534882018350, 100.2184796937738724 ) ) ;
#158917=CARTESIAN_POINT ( 'NONE',  ( -22.44159573604009950, -16.30477369853688430, 141.0750000027311728 ) ) ;
#158987=CARTESIAN_POINT ( 'NONE',  ( 17.14385361876520264, -23.59649016807270883, 144.0750000027311444 ) ) ;
#159064=CARTESIAN_POINT ( 'NONE',  ( -6.020228577223754586E-15, 39.95556452105416412, -6.249999994537626336 ) ) ;
#159104=DIRECTION ( 'NONE',  ( 0.000000000000000000, 0.000000000000000000, 1.000000000000000000 ) ) ;
#159113=CARTESIAN_POINT ( 'NONE',  ( -31.80000000000000782, -5.510910596163089556E-15, 45.00000000000000000 ) ) ;
#159114=CARTESIAN_POINT ( 'NONE',  ( -36.91746825000001309, 11.99521256947798342, -5.224999997268811924 ) ) ;
#159116=CARTESIAN_POINT ( 'NONE',  ( -35.70266437024448436, -0.4905633046376467465, 37.50000000000000000 ) ) ;
#159145=CARTESIAN_POINT ( 'NONE',  ( -5.950531402560715689E-15, 38.81732327939063509, -5.124999997268813168 ) ) ;
#159182=CARTESIAN_POINT ( 'NONE',  ( 30.82560697742735201, 2.428612866367529932E-14, 150.0000000000000000 ) ) ;
#159233=CARTESIAN_POINT ( 'NONE',  ( 33.80025371042794546, -2.440809870420986183, 99.93203653199846315 ) ) ;
#159266=CARTESIAN_POINT ( 'NONE',  ( -5.950531402560715689E-15, 38.81732327939063509, -7.124999997268814944 ) ) ;
#159357=CARTESIAN_POINT ( 'NONE',  ( -29.43349580481984162, 2.016473703290251599E-14, 139.9999999999999716 ) ) ;
#159358=CARTESIAN_POINT ( 'NONE',  ( 31.49170352461661793, -4.578070284816052826, 100.9457761758980325 ) ) ;
#159391=CARTESIAN_POINT ( 'NONE',  ( -17.81289503416611808, 24.51734667627700404, 145.6999999999999886 ) ) ;
#159412=CARTESIAN_POINT ( 'NONE',  ( 1.993301997531345292E-15, -30.30510711980685912, 140.7500000054623683 ) ) ;
#159501=EDGE_LOOP ( 'NONE', ( #127126, #109977, #109954, #96263 ) ) ;
#159504=CARTESIAN_POINT ( 'NONE',  ( -27.73933785331498925, -9.013057229001049109, 138.9750000027311785 ) ) ;
#159523=CARTESIAN_POINT ( 'NONE',  ( 36.78376627615639194, -4.378768456387976293, 48.34741972342520455 ) ) ;
#159574=TOROIDAL_SURFACE ( 'NONE', #149940, 2.700000000000000622, 0.2000000000000000111 ) ;
#159629=CARTESIAN_POINT ( 'NONE',  ( 22.81625015709509441, 31.40387420917330275, -5.324999997268812457 ) ) ;
#159630=CARTESIAN_POINT ( 'NONE',  ( -33.71430530369729439, 4.147805181855619416, 98.62971388258593208 ) ) ;
#159680=DIRECTION ( 'NONE',  ( 1.000000000000000000, 0.000000000000000000, 0.000000000000000000 ) ) ;
#159685=CARTESIAN_POINT ( 'NONE',  ( 34.36947210329395119, -7.112397586384675563, 47.39260519897412394 ) ) ;
#159700=CARTESIAN_POINT ( 'NONE',  ( 28.82186960331498327, 2.781578969918950771E-14, 141.0000000000000000 ) ) ;
#159704=DIRECTION ( 'NONE',  ( 0.000000000000000000, 0.000000000000000000, -1.000000000000000000 ) ) ;
#159721=VECTOR ( 'NONE', #86041, 1000.000000000000114 ) ;
#159741=( BOUNDED_CURVE ( )  B_SPLINE_CURVE ( 2, ( #61507, #32179, #34164, #79666, #93835, #112979, #189844, #17010, #51317, #823, #157510 ),
 .UNSPECIFIED., .F., .F. ) 
 B_SPLINE_CURVE_WITH_KNOTS ( ( 3, 2, 2, 2, 2, 3 ),
 ( 0.000000000000000000, 0.01999999999999999348, 0.03999999999999998695, 0.05999999999999998390, 0.07999999999999997391, 0.09999999999999997780 ),
 .UNSPECIFIED. ) 
 CURVE ( )  GEOMETRIC_REPRESENTATION_ITEM ( )  RATIONAL_B_SPLINE_CURVE ( ( 1.000000000000000000, 0.9510565162951535312, 1.000000000000000000, 0.9510565162951535312, 1.000000000000000000, 0.9510565162951535312, 1.000000000000000000, 0.9510565162951535312, 1.000000000000000000, 0.9510565162951536422, 0.9999999999999998890 ) ) 
 REPRESENTATION_ITEM ( '' )  );
#159751=PLANE ( 'NONE',  #149456 ) ;
#159880=LINE ( 'NONE', #3210, #57843 ) ;
#159886=CARTESIAN_POINT ( 'NONE',  ( -33.68492599513093211, -4.777136547582186310, 97.74919260172214308 ) ) ;
#159924=CARTESIAN_POINT ( 'NONE',  ( -27.73933785331498925, -9.013057229001049109, 147.4750000027311785 ) ) ;
#159996=CARTESIAN_POINT ( 'NONE',  ( -27.73933785331498925, 9.013057229001088189, 143.2750000027311899 ) ) ;
#160074=CARTESIAN_POINT ( 'NONE',  ( -11.74264578624800670, 36.14014761921585972, -2.149999994537626691 ) ) ;
#160126=CARTESIAN_POINT ( 'NONE',  ( -29.86685920354755197, -21.69954338932560134, -2.924999997268813878 ) ) ;
#160128=CYLINDRICAL_SURFACE ( 'NONE', #59745, 2.649999999999999467 ) ;
#160158=CARTESIAN_POINT ( 'NONE',  ( 29.86685920354754487, 21.69954338932564752, -5.424999997268813878 ) ) ;
#160280=CARTESIAN_POINT ( 'NONE',  ( -38.00000000000000711, 2.428612866367529932E-14, 1.084202172485504434E-16 ) ) ;
#160355=DIRECTION ( 'NONE',  ( -1.000000000000000000, -0.000000000000000000, -0.000000000000000000 ) ) ;
#160392=EDGE_LOOP ( 'NONE', ( #107222, #79135, #197098, #71411 ) ) ;
#160403=CARTESIAN_POINT ( 'NONE',  ( 28.82186960331499392, -9.364793116373510529, 140.9000000000000057 ) ) ;
#160425=CARTESIAN_POINT ( 'NONE',  ( 1.993301997531345292E-15, -30.30510711980685912, 138.7500000054623683 ) ) ;
#160455=CARTESIAN_POINT ( 'NONE',  ( -35.99626262588765968, 2.428612866367529932E-14, 2.000000000000000000 ) ) ;
#160514=ORIENTED_EDGE ( 'NONE', *, *, #40971, .F. ) ;
#160517=CARTESIAN_POINT ( 'NONE',  ( 22.44159573604009594, -16.30477369853687364, 139.6750000027311955 ) ) ;
#160575=ORIENTED_EDGE ( 'NONE', *, *, #49370, .T. ) ;
#160636=CARTESIAN_POINT ( 'NONE',  ( 22.81625015709510151, -31.40387420917324590, -3.924999997268811658 ) ) ;
#160637=CARTESIAN_POINT ( 'NONE',  ( -33.80093248007431583, 2.440252113607738416, 99.94207534358628209 ) ) ;
#160660=VECTOR ( 'NONE', #135283, 1000.000000000000000 ) ;
#160716=CARTESIAN_POINT ( 'NONE',  ( 37.99626262588764547, 12.34573411038917357, -4.902157773949822328 ) ) ;
#160734=DIRECTION ( 'NONE',  ( 1.000000000000000000, 0.000000000000000000, 0.000000000000000000 ) ) ;
#160773=CARTESIAN_POINT ( 'NONE',  ( -32.00000000000000000, -1.163414459189985801E-14, 95.00000000000000000 ) ) ;
#160815=ORIENTED_EDGE ( 'NONE', *, *, #197168, .T. ) ;
#160836=CARTESIAN_POINT ( 'NONE',  ( 11.74149087413295156, -36.13659316521243881, -5.402157773949823216 ) ) ;
#160868=CARTESIAN_POINT ( 'NONE',  ( 31.99364916730969455, -1.130961319020620804E-14, 97.65000000000020464 ) ) ;
#160926=CARTESIAN_POINT ( 'NONE',  ( -27.73933785331498925, 9.013057229001089965, 143.2750000027311899 ) ) ;
#160937=EDGE_LOOP ( 'NONE', ( #88614, #193976 ) ) ;
#160997=CARTESIAN_POINT ( 'NONE',  ( 27.73933785331498925, -9.013057229001034898, 148.2750000027311614 ) ) ;
#161073=CARTESIAN_POINT ( 'NONE',  ( 30.74264578624799782, 22.33583958711400541, -4.549999994537627046 ) ) ;
#161081=ORIENTED_EDGE ( 'NONE', *, *, #158766, .T. ) ;
#161094=ORIENTED_EDGE ( 'NONE', *, *, #99422, .F. ) ;
#161108=CARTESIAN_POINT ( 'NONE',  ( 31.25082632804103255, 7.456723613865053224, 95.94516017006306186 ) ) ;
#161123=CARTESIAN_POINT ( 'NONE',  ( -36.91746825000001309, -11.99521256947794789, -5.024999997268813523 ) ) ;
#161125=CARTESIAN_POINT ( 'NONE',  ( -34.91229673954799040, -6.363315211036966623, 41.02293916657588824 ) ) ;
#161127=CARTESIAN_POINT ( 'NONE',  ( -31.99364916731038022, -1.130961319012580892E-14, 92.35000000000000853 ) ) ;
#161140=ORIENTED_EDGE ( 'NONE', *, *, #186365, .T. ) ;
#161155=CARTESIAN_POINT ( 'NONE',  ( -22.81625015709509441, -31.40387420917324590, -6.324999997268814234 ) ) ;
#161198=ADVANCED_FACE ( 'NONE', ( #119359 ), #135528, .T. ) ;
#161277=CARTESIAN_POINT ( 'NONE',  ( 38.00000000000000000, 12.34694845685046616, -0.9000000000000000222 ) ) ;
#161380=DIRECTION ( 'NONE',  ( 0.000000000000000000, 0.000000000000000000, 1.000000000000000000 ) ) ;
#161400=CARTESIAN_POINT ( 'NONE',  ( -17.81289503416611808, 24.51734667627700404, 141.6999999999999602 ) ) ;
#161423=CARTESIAN_POINT ( 'NONE',  ( -27.73933785331498925, -9.013057229001049109, 146.9750000027311785 ) ) ;
#161429=LINE ( 'NONE', #37079, #192574 ) ;
#161434=SURFACE_STYLE_USAGE ( .BOTH. , #8760 ) ;
#161469=ORIENTED_EDGE ( 'NONE', *, *, #189746, .T. ) ;
#161533=CARTESIAN_POINT ( 'NONE',  ( -30.00000000000000000, -1.071565949253934124E-14, 102.5000000000000142 ) ) ;
#161626=CYLINDRICAL_SURFACE ( 'NONE', #134390, 37.99626262588765968 ) ;
#161678=FACE_OUTER_BOUND ( 'NONE', #143783, .T. ) ;
#161713=CARTESIAN_POINT ( 'NONE',  ( -37.99626262588766679, 2.428612866367529932E-14, 2.000000000000000000 ) ) ;
#161834=CARTESIAN_POINT ( 'NONE',  ( -22.81625015709509441, -31.40387420917324590, -10.82499999726881157 ) ) ;
#161873=EDGE_LOOP ( 'NONE', ( #180048, #26427, #49508, #88000 ) ) ;
#161885=CARTESIAN_POINT ( 'NONE',  ( -33.77897430376540910, -2.912663603757514874, 99.66889340242285300 ) ) ;
#161924=CARTESIAN_POINT ( 'NONE',  ( -8.571926809382608425, 26.38167802310805854, 140.9750000027312069 ) ) ;
#161955=DIRECTION ( 'NONE',  ( -1.000000000000000000, -0.000000000000000000, -3.709348145883536076E-20 ) ) ;
#162073=CARTESIAN_POINT ( 'NONE',  ( 23.48529157249600630, -32.32473071737749137, -5.049999994537627046 ) ) ;
#162075=B_SPLINE_CURVE_WITH_KNOTS ( 'NONE', 3,
 ( #65369, #187750, #110878, #143194, #117615, #113847, #50221, #172563, #128026, #83513, #20855, #157394, #145190, #18887, #67356, #81506, #71114, #40777, #111875, #52189, #190716, #174553, #173565, #179313, #9449, #98679, #35034, #96689, #158377, #175543, #97669, #4674, #164133, #5680, #189728, #51201, #112862, #159358, #102446, #82512, #195475, #105430, #73129, #43766, #167113, #44755, #89269, #90252 ),
 .UNSPECIFIED., .F., .F.,
 ( 4, 2, 2, 2, 2, 2, 2, 2, 2, 2, 2, 2, 2, 2, 2, 2, 2, 2, 2, 2, 2, 2, 2, 4 ),
 ( 0.04104976116627322147, 0.04252145193039932880, 0.04325729731246238247, 0.04399314269452542919, 0.04472898807658848286, 0.04546483345865153652, 0.04693652422277766467, 0.04840821498690379282, 0.04914406036896685342, 0.04987990575102992097, 0.05135159651515604912, 0.05208744189721910972, 0.05282328727928217726, 0.05429497804340830541, 0.05503082342547139377, 0.05576666880753447519, 0.05723835957166064498, 0.05871005033578681476, 0.05944589571784988230, 0.06018174109991294984, 0.06165343186403906411, 0.06238927724610211778, 0.06312512262816517838, 0.06459681339229128572 ),
 .UNSPECIFIED. ) ;
#162111=CARTESIAN_POINT ( 'NONE',  ( 31.54545164052520434, 7.106679946642015189, 92.55365670706888181 ) ) ;
#162155=CARTESIAN_POINT ( 'NONE',  ( -36.99206003604233217, 5.206627989871537743, 43.21856904651837539 ) ) ;
#162263=CARTESIAN_POINT ( 'NONE',  ( -32.00000000000000711, -1.130348995613007185E-14, 97.69999999999998863 ) ) ;
#162277=CARTESIAN_POINT ( 'NONE',  ( 29.86685920354754842, -21.69954338932559068, -9.824999997268813345 ) ) ;
#162322=ORIENTED_EDGE ( 'NONE', *, *, #65800, .T. ) ;
#162393=CARTESIAN_POINT ( 'NONE',  ( 8.906447517083057264, -27.41122689804191026, 142.5999999999999943 ) ) ;
#162395=CARTESIAN_POINT ( 'NONE',  ( 23.31738231874054890, -16.94106989632523508, 139.0500000054623513 ) ) ;
#162427=CARTESIAN_POINT ( 'NONE',  ( 32.00000000000000000, -5.510910596163089556E-15, 42.35000000000000142 ) ) ;
#162507=VERTEX_POINT ( 'NONE', #32476 ) ;
#162527=CARTESIAN_POINT ( 'NONE',  ( 36.84749596837620089, -2.912325675875791386, 49.66910675224615801 ) ) ;
#162562=CARTESIAN_POINT ( 'NONE',  ( -3.573655867282028392E-15, 2.428612866367529932E-14, 2.000000000000000000 ) ) ;
#162601=CARTESIAN_POINT ( 'NONE',  ( -4.945344302077486986, 37.34563040183822835, -8.000000000000000000 ) ) ;
#162621=CARTESIAN_POINT ( 'NONE',  ( -3.573655867282028392E-15, 2.428612866367529932E-14, 2.000000000000000000 ) ) ;
#162631=CARTESIAN_POINT ( 'NONE',  ( 22.81625015709510151, -31.40387420917324590, -9.924999997268814766 ) ) ;
#162656=CARTESIAN_POINT ( 'NONE',  ( -34.67490207739297148, 3.335485537672764345, 51.73549893453299120 ) ) ;
#162675=EDGE_CURVE ( 'NONE', #188321, #8281, #17306, .T. ) ;
#162834=CARTESIAN_POINT ( 'NONE',  ( 26.98314665059723083, -25.22428982341646275, -8.000000000000003553 ) ) ;
#162884=CARTESIAN_POINT ( 'NONE',  ( -34.16298174666833631, -4.140866818352566092, 91.36220571553955949 ) ) ;
#162897=CARTESIAN_POINT ( 'NONE',  ( -36.91746825000000598, 2.428612866367529932E-14, -1.124999997268813390 ) ) ;
#162906=AXIS2_PLACEMENT_3D ( 'NONE', #114274, #145619, #127456 ) ;
#162918=CARTESIAN_POINT ( 'NONE',  ( -31.64921935833423561, -6.825000981063952921, 91.88079052344197351 ) ) ;
#162923=CARTESIAN_POINT ( 'NONE',  ( 8.571926809382597767, 26.38167802310806209, 142.7750000027311899 ) ) ;
#162996=ORIENTED_EDGE ( 'NONE', *, *, #72915, .F. ) ;
#162999=CARTESIAN_POINT ( 'NONE',  ( -22.44159573604010305, 16.30477369853692338, 148.6750000027311671 ) ) ;
#163009=DIRECTION ( 'NONE',  ( 1.000000000000000000, -0.000000000000000000, -0.000000000000000000 ) ) ;
#163067=CIRCLE ( 'NONE', #127541, 5.500000000001017852 ) ;
#163075=( BOUNDED_CURVE ( )  B_SPLINE_CURVE ( 2, ( #55409, #132255, #150436, #194939, #102916, #54415, #117080, #24089, #40241, #133247, #176779 ),
 .UNSPECIFIED., .F., .T. ) 
 B_SPLINE_CURVE_WITH_KNOTS ( ( 3, 2, 2, 2, 2, 3 ),
 ( 0.4000000000000003553, 0.4200000000000003175, 0.4400000000000003908, 0.4600000000000004086, 0.4800000000000004263, 0.5000000000000004441 ),
 .UNSPECIFIED. ) 
 CURVE ( )  GEOMETRIC_REPRESENTATION_ITEM ( )  RATIONAL_B_SPLINE_CURVE ( ( 0.9999999999999992228, 0.9510565162951543083, 1.000000000000000000, 0.9510565162951535312, 1.000000000000000000, 0.9510565162951535312, 1.000000000000000000, 0.9510565162951535312, 1.000000000000000000, 0.9510565162951524210, 1.000000000000001110 ) ) 
 REPRESENTATION_ITEM ( '' )  );
#163077=CARTESIAN_POINT ( 'NONE',  ( -23.48529157249600985, 32.32473071737754111, -8.049999994537627046 ) ) ;
#163114=CARTESIAN_POINT ( 'NONE',  ( 31.76179951907201371, 6.484602924383669809, 91.22381659560102207 ) ) ;
#163119=DIRECTION ( 'NONE',  ( -1.000000000000000000, 0.000000000000000000, -6.982962677686266711E-15 ) ) ;
#163127=CARTESIAN_POINT ( 'NONE',  ( 36.81781682666242261, 5.501098665926424935, 45.34601664933739329 ) ) ;
#163146=ORIENTED_EDGE ( 'NONE', *, *, #144706, .F. ) ;
#163175=DIRECTION ( 'NONE',  ( 0.000000000000000000, 0.000000000000000000, -1.000000000000000000 ) ) ;
#163287=CARTESIAN_POINT ( 'NONE',  ( -38.00000000000001421, 12.34694845685046438, -6.099999999999999645 ) ) ;
#163294=DIRECTION ( 'NONE',  ( -1.000000000000000000, -0.000000000000000000, -3.709348145883536076E-20 ) ) ;
#163379=CARTESIAN_POINT ( 'NONE',  ( 37.99626262588765258, 2.893932880411085066E-14, -6.747842220587804363 ) ) ;
#163411=CARTESIAN_POINT ( 'NONE',  ( 28.82186960331499392, -9.364793116373510529, 144.9000000000000057 ) ) ;
#163427=ORIENTED_EDGE ( 'NONE', *, *, #177539, .T. ) ;
#163460=CARTESIAN_POINT ( 'NONE',  ( 23.31738231874054890, -16.94106989632523508, 147.0500000054623797 ) ) ;
#163495=DIRECTION ( 'NONE',  ( 0.000000000000000000, 0.000000000000000000, -1.000000000000000000 ) ) ;
#163538=CARTESIAN_POINT ( 'NONE',  ( -28.88419406831849301, 24.88742053112121511, -7.973410913627005492 ) ) ;
#163614=DIRECTION ( 'NONE',  ( 0.000000000000000000, 0.000000000000000000, 1.000000000000000000 ) ) ;
#163701=CYLINDRICAL_SURFACE ( 'NONE', #140274, 28.82186960331498682 ) ;
#163743=DIRECTION ( 'NONE',  ( -1.000000000000000000, 0.000000000000000000, -6.982962677686266711E-15 ) ) ;
#163838=ADVANCED_FACE ( 'NONE', ( #123235 ), #16080, .F. ) ;
#163846=CARTESIAN_POINT ( 'NONE',  ( 37.99626262588765258, 2.893932880411085066E-14, -5.002157773949823749 ) ) ;
#163865=EDGE_LOOP ( 'NONE', ( #100495, #175448, #93246, #15731, #44270, #156102, #141232, #118649, #35744, #65474 ) ) ;
#163891=VERTEX_POINT ( 'NONE', #151617 ) ;
#163907=CARTESIAN_POINT ( 'NONE',  ( -37.51207494968712552, -5.596088347520207229, -8.000000000000000000 ) ) ;
#163940=CARTESIAN_POINT ( 'NONE',  ( -31.27032343591157471, -7.501918430611450361, 95.46114142609054909 ) ) ;
#163944=CARTESIAN_POINT ( 'NONE',  ( 17.14385361876520264, -23.59649016807271238, 142.0750000027311444 ) ) ;
#163949=( NAMED_UNIT ( * ) SI_UNIT ( $, .STERADIAN. ) SOLID_ANGLE_UNIT ( ) );
#163957=ORIENTED_EDGE ( 'NONE', *, *, #37951, .T. ) ;
#164015=ORIENTED_EDGE ( 'NONE', *, *, #60978, .F. ) ;
#164018=CARTESIAN_POINT ( 'NONE',  ( -8.571926809382601320, -26.38167802310801591, 147.2750000027311899 ) ) ;
#164037=CYLINDRICAL_SURFACE ( 'NONE', #37154, 28.82186960331498682 ) ;
#164090=CARTESIAN_POINT ( 'NONE',  ( -38.00000000000000711, 2.428612866367529932E-14, -11.74999999453762634 ) ) ;
#164104=ORIENTED_EDGE ( 'NONE', *, *, #13961, .T. ) ;
#164126=CARTESIAN_POINT ( 'NONE',  ( 31.24009710442676280, 7.113574878955725822, 97.38907943302065462 ) ) ;
#164133=CARTESIAN_POINT ( 'NONE',  ( 31.28611164036840364, -6.519914617504974252, 98.73992561365416520 ) ) ;
#164144=CARTESIAN_POINT ( 'NONE',  ( -34.78522506798723413, -4.592425496937305498E-15, 52.50000000000000000 ) ) ;
#164225=CARTESIAN_POINT ( 'NONE',  ( -28.28060372831499336, 2.428612866367529932E-14, 149.6875000013656063 ) ) ;
#164256=LINE ( 'NONE', #93092, #150505 ) ;
#164294=ORIENTED_EDGE ( 'NONE', *, *, #89680, .F. ) ;
#164299=CARTESIAN_POINT ( 'NONE',  ( -30.74264578624800492, 22.33583958711400186, -2.200000000000000178 ) ) ;
#164388=CARTESIAN_POINT ( 'NONE',  ( 37.99626262588768810, 12.34573411038912027, -6.647842220587802942 ) ) ;
#164417=CARTESIAN_POINT ( 'NONE',  ( -8.906447517083060816, 27.41122689804195645, 143.5999999999999943 ) ) ;
#164472=ORIENTED_EDGE ( 'NONE', *, *, #60352, .T. ) ;
#164615=CARTESIAN_POINT ( 'NONE',  ( 5.714903183877464876, 37.05114278946271611, -8.000000000000000000 ) ) ;
#164618=CARTESIAN_POINT ( 'NONE',  ( -67.00000000000000000, -5.510910596163089556E-15, 39.49999999999996447 ) ) ;
#164631=ORIENTED_EDGE ( 'NONE', *, *, #135020, .T. ) ;
#164645=CARTESIAN_POINT ( 'NONE',  ( -22.44159573604010305, 16.30477369853692338, 149.1750000027311671 ) ) ;
#164887=DIRECTION ( 'NONE',  ( -1.000000000000000000, -0.000000000000000000, -3.709348145883536076E-20 ) ) ;
#164893=CARTESIAN_POINT ( 'NONE',  ( 36.91746824999999177, 2.880721459617395097E-14, -4.124999997268813168 ) ) ;
#164899=CARTESIAN_POINT ( 'NONE',  ( -34.46475727851697002, -1.773375775694353562, 89.78131888620559664 ) ) ;
#164910=LINE ( 'NONE', #26404, #143376 ) ;
#164920=ORIENTED_EDGE ( 'NONE', *, *, #169778, .F. ) ;
#164934=ORIENTED_EDGE ( 'NONE', *, *, #16286, .T. ) ;
#164935=CARTESIAN_POINT ( 'NONE',  ( -32.33375351741885595, -3.966103829525452262, 88.62974963220463565 ) ) ;
#164939=CARTESIAN_POINT ( 'NONE',  ( 1.784210473542230573E-15, -29.16686587814331588, 141.8750000027311842 ) ) ;
#165082=CARTESIAN_POINT ( 'NONE',  ( -22.81625015709509441, -31.40387420917324590, -2.824999997268812901 ) ) ;
#165095=( BOUNDED_SURFACE ( )  B_SPLINE_SURFACE ( 1, 2, ( 
 ( #177266, #93674, #36714, #128723, #160074, #142899, #192421, #35731, #4381, #21561, #82209, #193422, #114560, #112568, #158083, #66066, #7377, #115578, #37728, #100395, #19575, #22568, #97378, #99390, #51896, #189434, #127732, #81218, #161073, #50910, #174263, #38737, #84214, #162073, #145894, #190420, #129712, #68058, #69062, #113555, #143900, #131740, #83221, #108846, #144896, #159064, #20558, #70072, #6378, #130729, #53903, #32016, #191409, #5382, #67065, #52885, #23569, #85217, #8397, #133736, #72062, #9405, #101384, #163077, #120543, #24580, #132737, #102403, #134751, #167069, #42735, #43721, #73079, #136710, #71071, #26576, #194425, #74069, #166079, #147919, #58877, #89220, #57903, #27582, #54897, #86229, #116571, #55895, #117568, #75044, #87233, #196433, #103404, #11410, #39721, #179269, #40733, #90207, #119575, #104397, #164090 ),
 ( #181258, #13380, #195430, #10405, #151890, #150913, #12407, #25589, #56906, #148916, #118580, #135740, #178260, #149903, #180270, #197411, #41740, #165082, #28570, #88219, #182236, #105382, #106366, #169023, #17349, #109348, #172023, #33512, #31524, #44711, #184217, #152868, #95171, #45699, #171030, #156859, #93177, #78008, #107350, #80009, #91179, #62838, #61840, #18354, #154862, #138691, #123510, #198391, #32521, #94173, #139675, #79005, #16360, #59868, #14363, #155852, #30528, #76028, #153865, #63851, #1163, #140679, #124522, #186217, #172, #47698, #2171, #48689, #15363, #168049, #92181, #125522, #187219, #110342, #121535, #137703, #183230, #29546, #199388, #60852, #77019, #122527, #185203, #46694, #108355, #170034, #52654, #34507, #145658, #176019, #144660, #114317, #141678, #49674, #3169, #188202, #142668, #161834, #174025, #21326, #190182 ) ),
 .UNSPECIFIED., .F., .F., .F. ) 
 B_SPLINE_SURFACE_WITH_KNOTS ( ( 2, 2 ),
 ( 3, 2, 2, 2, 2, 2, 2, 2, 2, 2, 2, 2, 2, 2, 2, 2, 2, 2, 2, 2, 2, 2, 2, 2, 2, 2, 2, 2, 2, 2, 2, 2, 2, 2, 2, 2, 2, 2, 2, 2, 2, 2, 2, 2, 2, 2, 2, 2, 2, 2, 3 ),
 ( 0.000000000000000000, 1.000000000000000000 ),
 ( 0.000000000000000000, 0.02000000000000000042, 0.04000000000000000083, 0.05999999999999999778, 0.08000000000000000167, 0.1000000000000000056, 0.1199999999999999956, 0.1400000000000000133, 0.1600000000000000033, 0.1799999999999999933, 0.2000000000000000111, 0.2200000000000000011, 0.2399999999999999911, 0.2600000000000000089, 0.2800000000000000266, 0.2999999999999999889, 0.3200000000000000067, 0.3400000000000000244, 0.3599999999999999867, 0.3800000000000000044, 0.4000000000000000222, 0.4199999999999999845, 0.4400000000000000022, 0.4600000000000000200, 0.4799999999999999822, 0.5000000000000000000, 0.5200000000000000178, 0.5400000000000000355, 0.5600000000000000533, 0.5799999999999999600, 0.5999999999999999778, 0.6199999999999999956, 0.6400000000000000133, 0.6600000000000000311, 0.6800000000000000488, 0.6999999999999999556, 0.7199999999999999734, 0.7399999999999999911, 0.7600000000000000089, 0.7800000000000000266, 0.8000000000000000444, 0.8199999999999999512, 0.8399999999999999689, 0.8599999999999999867, 0.8800000000000000044, 0.9000000000000000222, 0.9200000000000000400, 0.9399999999999999467, 0.9599999999999999645, 0.9799999999999999822, 1.000000000000000000 ),
 .UNSPECIFIED. ) 
 GEOMETRIC_REPRESENTATION_ITEM ( )  RATIONAL_B_SPLINE_SURFACE ( (
 ( 1.000000000000000000, 0.9510565162951535312, 1.000000000000000000, 0.9510565162951535312, 1.000000000000000000, 0.9510565162951535312, 1.000000000000000000, 0.9510565162951535312, 1.000000000000000000, 0.9510565162951535312, 1.000000000000000000, 0.9510565162951535312, 1.000000000000000000, 0.9510565162951535312, 1.000000000000000000, 0.9510565162951535312, 1.000000000000000000, 0.9510565162951535312, 1.000000000000000000, 0.9510565162951535312, 1.000000000000000000, 0.9510565162951535312, 1.000000000000000000, 0.9510565162951535312, 1.000000000000000000, 0.9510565162951535312, 1.000000000000000000, 0.9510565162951535312, 1.000000000000000000, 0.9510565162951535312, 1.000000000000000000, 0.9510565162951535312, 1.000000000000000000, 0.9510565162951535312, 1.000000000000000000, 0.9510565162951535312, 1.000000000000000000, 0.9510565162951535312, 1.000000000000000000, 0.9510565162951535312, 1.000000000000000000, 0.9510565162951535312, 1.000000000000000000, 0.9510565162951535312, 1.000000000000000000, 0.9510565162951535312, 1.000000000000000000, 0.9510565162951535312, 1.000000000000000000, 0.9510565162951535312, 1.000000000000000000, 0.9510565162951535312, 1.000000000000000000, 0.9510565162951535312, 1.000000000000000000, 0.9510565162951535312, 1.000000000000000000, 0.9510565162951535312, 1.000000000000000000, 0.9510565162951535312, 1.000000000000000000, 0.9510565162951535312, 1.000000000000000000, 0.9510565162951535312, 1.000000000000000000, 0.9510565162951535312, 1.000000000000000000, 0.9510565162951535312, 1.000000000000000000, 0.9510565162951535312, 1.000000000000000000, 0.9510565162951535312, 1.000000000000000000, 0.9510565162951535312, 1.000000000000000000, 0.9510565162951535312, 1.000000000000000000, 0.9510565162951535312, 1.000000000000000000, 0.9510565162951535312, 1.000000000000000000, 0.9510565162951535312, 1.000000000000000000, 0.9510565162951535312, 1.000000000000000000, 0.9510565162951535312, 1.000000000000000000, 0.9510565162951535312, 1.000000000000000000, 0.9510565162951535312, 1.000000000000000000, 0.9510565162951535312, 1.000000000000000000, 0.9510565162951535312, 1.000000000000000000, 0.9510565162951535312, 1.000000000000000000, 0.9510565162951535312, 1.000000000000000000, 0.9510565162951535312, 1.000000000000000000),
 ( 1.000000000000000000, 0.9510565162951535312, 1.000000000000000000, 0.9510565162951535312, 1.000000000000000000, 0.9510565162951535312, 1.000000000000000000, 0.9510565162951535312, 1.000000000000000000, 0.9510565162951535312, 1.000000000000000000, 0.9510565162951535312, 1.000000000000000000, 0.9510565162951535312, 1.000000000000000000, 0.9510565162951535312, 1.000000000000000000, 0.9510565162951535312, 1.000000000000000000, 0.9510565162951535312, 1.000000000000000000, 0.9510565162951535312, 1.000000000000000000, 0.9510565162951535312, 1.000000000000000000, 0.9510565162951535312, 1.000000000000000000, 0.9510565162951535312, 1.000000000000000000, 0.9510565162951535312, 1.000000000000000000, 0.9510565162951535312, 1.000000000000000000, 0.9510565162951535312, 1.000000000000000000, 0.9510565162951535312, 1.000000000000000000, 0.9510565162951535312, 1.000000000000000000, 0.9510565162951535312, 1.000000000000000000, 0.9510565162951535312, 1.000000000000000000, 0.9510565162951535312, 1.000000000000000000, 0.9510565162951535312, 1.000000000000000000, 0.9510565162951535312, 1.000000000000000000, 0.9510565162951535312, 1.000000000000000000, 0.9510565162951535312, 1.000000000000000000, 0.9510565162951535312, 1.000000000000000000, 0.9510565162951535312, 1.000000000000000000, 0.9510565162951535312, 1.000000000000000000, 0.9510565162951535312, 1.000000000000000000, 0.9510565162951535312, 1.000000000000000000, 0.9510565162951535312, 1.000000000000000000, 0.9510565162951535312, 1.000000000000000000, 0.9510565162951535312, 1.000000000000000000, 0.9510565162951535312, 1.000000000000000000, 0.9510565162951535312, 1.000000000000000000, 0.9510565162951535312, 1.000000000000000000, 0.9510565162951535312, 1.000000000000000000, 0.9510565162951535312, 1.000000000000000000, 0.9510565162951535312, 1.000000000000000000, 0.9510565162951535312, 1.000000000000000000, 0.9510565162951535312, 1.000000000000000000, 0.9510565162951535312, 1.000000000000000000, 0.9510565162951535312, 1.000000000000000000, 0.9510565162951535312, 1.000000000000000000, 0.9510565162951535312, 1.000000000000000000, 0.9510565162951535312, 1.000000000000000000, 0.9510565162951535312, 1.000000000000000000, 0.9510565162951535312, 1.000000000000000000, 0.9510565162951535312, 1.000000000000000000) ) ) 
 REPRESENTATION_ITEM ( '' )  SURFACE ( )  );
#165139=CARTESIAN_POINT ( 'NONE',  ( -34.61318912441601015, -7.252276964307558416, 43.02678305251433244 ) ) ;
#165162=DIRECTION ( 'NONE',  ( 1.000000000000000000, -0.000000000000000000, -0.000000000000000000 ) ) ;
#165167=CARTESIAN_POINT ( 'NONE',  ( -37.24189295061466254, 4.138848244557342682, 41.36027101465353439 ) ) ;
#165178=CARTESIAN_POINT ( 'NONE',  ( -22.44159573604010305, 16.30477369853692338, 142.6750000027311671 ) ) ;
#165249=CARTESIAN_POINT ( 'NONE',  ( -32.45668260148361384, 3.101559039593200673, 88.16695215365973581 ) ) ;
#165279=ORIENTED_EDGE ( 'NONE', *, *, #64977, .F. ) ;
#165292=CARTESIAN_POINT ( 'NONE',  ( 23.48529157249600630, -32.32473071737749137, -3.300000000000000266 ) ) ;
#165381=ADVANCED_FACE ( 'NONE', ( #176393 ), #63641, .T. ) ;
#165465=CARTESIAN_POINT ( 'NONE',  ( -37.99626262588766679, 2.428612866367529932E-14, -0.002157773949821304490 ) ) ;
#165492=FACE_OUTER_BOUND ( 'NONE', #67683, .T. ) ;
#165528=FACE_OUTER_BOUND ( 'NONE', #81800, .T. ) ;
#165611=CARTESIAN_POINT ( 'NONE',  ( -25.52603992809234157, 28.15638454425511839, -8.000000000000001776 ) ) ;
#165640=CARTESIAN_POINT ( 'NONE',  ( -22.81625015709509441, -31.40387420917324590, -10.32499999726881157 ) ) ;
#165664=CARTESIAN_POINT ( 'NONE',  ( -34.91303292417841675, 6.360705039060875698, 41.01876028008880581 ) ) ;
#165777=CARTESIAN_POINT ( 'NONE',  ( -37.99626262588765968, 12.34573411038917179, -3.847842220587804007 ) ) ;
#165847=CARTESIAN_POINT ( 'NONE',  ( -32.00000000000000000, -5.510910596163089556E-15, 45.00000000000000000 ) ) ;
#165886=CARTESIAN_POINT ( 'NONE',  ( -22.81625015709509441, -31.40387420917324590, -4.824999997268813345 ) ) ;
#165892=CARTESIAN_POINT ( 'NONE',  ( -33.73406392173259150, -5.500497537618388222, 95.16330145977875077 ) ) ;
#165893=LINE ( 'NONE', #39536, #150248 ) ;
#165905=CARTESIAN_POINT ( 'NONE',  ( -5.950531402560715689E-15, 38.81732327939063509, -1.624999997268813390 ) ) ;
#165933=CARTESIAN_POINT ( 'NONE',  ( 17.14385361876520264, -23.59649016807271238, 140.0750000027311728 ) ) ;
#166044=DIRECTION ( 'NONE',  ( 0.06104853953485701173, 0.000000000000000000, -0.9981347984218670311 ) ) ;
#166079=CARTESIAN_POINT ( 'NONE',  ( -30.74264578624800492, -22.33583958711396278, -9.549999994537627046 ) ) ;
#166090=VERTEX_POINT ( 'NONE', #100526 ) ;
#166133=CARTESIAN_POINT ( 'NONE',  ( 36.81592377195799060, 3.639597414954547805, 49.13916779353751707 ) ) ;
#166161=CYLINDRICAL_SURFACE ( 'NONE', #43933, 2.649999999999999467 ) ;
#166166=CARTESIAN_POINT ( 'NONE',  ( -36.78335851983072047, 5.362873614019889601, 46.23361200806721882 ) ) ;
#166172=CARTESIAN_POINT ( 'NONE',  ( 22.44159573604009239, 16.30477369853692693, 148.0750000027312012 ) ) ;
#166177=CARTESIAN_POINT ( 'NONE',  ( 1.784210473542230573E-15, -29.16686587814331588, 147.3750000027311842 ) ) ;
#166207=EDGE_LOOP ( 'NONE', ( #39818, #94483, #132126, #107954 ) ) ;
#166228=CIRCLE ( 'NONE', #27393, 2.649999999999999467 ) ;
#166244=DIRECTION ( 'NONE',  ( 1.000000000000000000, 0.000000000000000000, 0.000000000000000000 ) ) ;
#166279=EDGE_CURVE ( 'NONE', #122084, #99233, #144300, .T. ) ;
#166291=CARTESIAN_POINT ( 'NONE',  ( -6.020228577223754586E-15, 39.95556452105416412, -6.500000000000000000 ) ) ;
#166394=MECHANICAL_DESIGN_GEOMETRIC_PRESENTATION_REPRESENTATION('',(#88862),#66184);
#166544=CARTESIAN_POINT ( 'NONE',  ( 37.24135263299451992, -4.142047767899329713, 41.36355589474229788 ) ) ;
#166630=CARTESIAN_POINT ( 'NONE',  ( -37.99626262588766679, 2.428612866367529932E-14, -2.002157773949823305 ) ) ;
#166640=CARTESIAN_POINT ( 'NONE',  ( -27.73933785331498925, 2.428612866367529932E-14, 147.3750000027311842 ) ) ;
#166665=CARTESIAN_POINT ( 'NONE',  ( -34.38695055765524700, 7.456135981908278865, 45.94887894546500462 ) ) ;
#166700=ORIENTED_EDGE ( 'NONE', *, *, #8154, .F. ) ;
#166739=ORIENTED_EDGE ( 'NONE', *, *, #29683, .T. ) ;
#166742=DIRECTION ( 'NONE',  ( 0.000000000000000000, 0.000000000000000000, -1.000000000000000000 ) ) ;
#166883=CARTESIAN_POINT ( 'NONE',  ( -22.81625015709510507, 31.40387420917330275, -0.9249999972688132122 ) ) ;
#166890=CARTESIAN_POINT ( 'NONE',  ( 11.74149087413295156, -36.13659316521243881, -1.402157773949822550 ) ) ;
#166911=EDGE_LOOP ( 'NONE', ( #19463, #110973, #42414, #194678 ) ) ;
#166959=DIRECTION ( 'NONE',  ( 0.000000000000000000, 0.000000000000000000, 1.000000000000000000 ) ) ;
#167008=CIRCLE ( 'NONE', #79812, 40.00000000000002132 ) ;
#167069=CARTESIAN_POINT ( 'NONE',  ( 38.00000000000000000, 12.34694845685046616, -8.649999994537624914 ) ) ;
#167113=CARTESIAN_POINT ( 'NONE',  ( 31.69386653422658640, -1.706804019390332661, 102.3073255780427360 ) ) ;
#167161=CARTESIAN_POINT ( 'NONE',  ( 17.14385361876520264, -23.59649016807271238, 145.5750000027312012 ) ) ;
#167166=CARTESIAN_POINT ( 'NONE',  ( 27.73933785331498214, 9.013057229001095294, 143.9750000027312069 ) ) ;
#167188=AXIS2_PLACEMENT_3D ( 'NONE', #11945, #25115, #148442 ) ;
#167198=ORIENTED_EDGE ( 'NONE', *, *, #82089, .F. ) ;
#167207=( BOUNDED_CURVE ( )  B_SPLINE_CURVE ( 2, ( #92248, #17413, #140744, #107416, #47760, #111405, #18419, #172087, #173091, #125584, #33574 ),
 .UNSPECIFIED., .F., .T. ) 
 B_SPLINE_CURVE_WITH_KNOTS ( ( 3, 2, 2, 2, 2, 3 ),
 ( 0.2002265011048941501, 0.2199999999999999734, 0.2400000000000000189, 0.2600000000000000089, 0.2800000000000000822, 0.3000000000000000999 ),
 .UNSPECIFIED. ) 
 CURVE ( )  GEOMETRIC_REPRESENTATION_ITEM ( )  RATIONAL_B_SPLINE_CURVE ( ( 0.9989039793630181130, 0.9516108039519795003, 1.000000000000000000, 0.9510565162951535312, 1.000000000000000000, 0.9510565162951535312, 1.000000000000000000, 0.9510565162951535312, 1.000000000000000000, 0.9510565162951534202, 1.000000000000000222 ) ) 
 REPRESENTATION_ITEM ( '' )  );
#167212=DIRECTION ( 'NONE',  ( 0.000000000000000000, 0.000000000000000000, 1.000000000000000000 ) ) ;
#167235=CARTESIAN_POINT ( 'NONE',  ( -40.00200000000003087, -1.163414459189985801E-14, 95.00000000000000000 ) ) ;
#167273=CARTESIAN_POINT ( 'NONE',  ( -38.00000000000001421, -12.34694845685042708, -1.899999999999999911 ) ) ;
#167328=CARTESIAN_POINT ( 'NONE',  ( 34.38695055765521857, 7.456135981908276200, 45.94887894546498330 ) ) ;
#167461=( BOUNDED_CURVE ( )  B_SPLINE_CURVE ( 2, ( #91788, #123135, #77634, #139303, #781, #114937, #19938, #81579, #141291, #50293, #95781 ),
 .UNSPECIFIED., .F., .T. ) 
 B_SPLINE_CURVE_WITH_KNOTS ( ( 3, 2, 2, 2, 2, 3 ),
 ( 0.7000000000000006217, 0.7200000000000006395, 0.7400000000000006573, 0.7600000000000006750, 0.7800000000000006928, 0.8000000000000007105 ),
 .UNSPECIFIED. ) 
 CURVE ( )  GEOMETRIC_REPRESENTATION_ITEM ( )  RATIONAL_B_SPLINE_CURVE ( ( 0.9999999999999983347, 0.9510565162951551965, 1.000000000000000000, 0.9510565162951535312, 1.000000000000000000, 0.9510565162951535312, 1.000000000000000000, 0.9510565162951535312, 1.000000000000000000, 0.9510565162951518658, 1.000000000000001554 ) ) 
 REPRESENTATION_ITEM ( '' )  );
#167555=EDGE_LOOP ( 'NONE', ( #109696, #187091, #91727 ) ) ;
#167595=CARTESIAN_POINT ( 'NONE',  ( -36.77739090780051612, -5.326908766905468440, 46.41547615974453578 ) ) ;
#167615=DIRECTION ( 'NONE',  ( 0.000000000000000000, 0.000000000000000000, 1.000000000000000000 ) ) ;
#167625=CARTESIAN_POINT ( 'NONE',  ( -17.14385361876520619, 23.59649016807275856, 141.0750000027311728 ) ) ;
#167650=CARTESIAN_POINT ( 'NONE',  ( -8.906447517083053711, -27.41122689804191026, 146.6500000054623740 ) ) ;
#167672=CARTESIAN_POINT ( 'NONE',  ( 11.74149087413295156, -36.13659316521243881, -7.147842220587802942 ) ) ;
#167737=CARTESIAN_POINT ( 'NONE',  ( -27.73933785331498925, 2.428612866367529932E-14, 139.3750000027311842 ) ) ;
#167862=CARTESIAN_POINT ( 'NONE',  ( 11.40812507854755253, -35.11059874428192273, -2.024999997268813079 ) ) ;
#167863=CARTESIAN_POINT ( 'NONE',  ( -34.40575365382724016, 2.434396366613705176, 90.06480789948632548 ) ) ;
#167868=CARTESIAN_POINT ( 'NONE',  ( 34.29436769411893948, 3.356737774573909316, 90.62828869849683144 ) ) ;
#167881=CARTESIAN_POINT ( 'NONE',  ( -36.91746825000000598, 2.428612866367529932E-14, -5.124999997268813168 ) ) ;
#167889=VERTEX_POINT ( 'NONE', #187668 ) ;
#167977=CARTESIAN_POINT ( 'NONE',  ( -28.82186960331499037, 2.428612866367529932E-14, 140.2500000054623683 ) ) ;
#168049=CARTESIAN_POINT ( 'NONE',  ( 36.91746824999999887, 11.99521256947799053, -8.024999997268814411 ) ) ;
#168135=CARTESIAN_POINT ( 'NONE',  ( 27.73933785331498925, -9.013057229001033122, 145.7750000027311899 ) ) ;
#168140=CARTESIAN_POINT ( 'NONE',  ( 17.14385361876520264, -23.59649016807271238, 143.5750000027312012 ) ) ;
#168149=ORIENTED_EDGE ( 'NONE', *, *, #113740, .F. ) ;
#168186=LINE ( 'NONE', #16497, #31074 ) ;
#168210=CARTESIAN_POINT ( 'NONE',  ( -17.81289503416611097, -24.51734667627696496, 146.2999999999999829 ) ) ;
#168302=CARTESIAN_POINT ( 'NONE',  ( 35.44323460151742466, 3.757829821678515980, 38.50466947567800702 ) ) ;
#168334=DIRECTION ( 'NONE',  ( -1.000000000000000000, 0.000000000000000000, 0.000000000000000000 ) ) ;
#168370=CARTESIAN_POINT ( 'NONE',  ( 8.906447517083050158, 27.41122689804195645, 147.6500000054623740 ) ) ;
#168377=( BOUNDED_CURVE ( )  B_SPLINE_CURVE ( 2, ( #162897, #24406, #197242, #135570, #147744, #165905, #194254, #104224, #196264, #56735, #55721, #41567, #102230, #117393, #72908, #179092, #27403, #40561, #25415, #180099, #148742, #134577, #26406, #58703, #89048, #57733, #73900, #43549, #991, #31354, #186040, #140510, #106197, #91999, #110174, #153693, #48520, #152697, #155683, #77841, #167881, #29380, #1999, #183058, #91011, #185033, #14186, #108179, #79838, #169860, #141508, #138519, #93005, #18181, #16186, #199213, #123340, #46520, #63678, #154691, #139508, #125353, #187050, #171853, #62665, #75855, #156687, #2993, #15189, #61671, #33341 ),
 .UNSPECIFIED., .F., .T. ) 
 B_SPLINE_CURVE_WITH_KNOTS ( ( 3, 2, 2, 2, 2, 2, 2, 2, 2, 2, 2, 2, 2, 2, 2, 2, 2, 2, 2, 2, 2, 2, 2, 2, 2, 2, 2, 2, 2, 2, 2, 2, 2, 2, 2, 3 ),
 ( 0.000000000000000000, 0.02000000000000000042, 0.04000000000000000083, 0.05999999999999999084, 0.08000000000000000167, 0.1000000000000000056, 0.1199999999999999817, 0.1400000000000000133, 0.1600000000000000033, 0.1799999999999999933, 0.2000000000000000111, 0.2200000000000000011, 0.2399999999999999634, 0.2600000000000000089, 0.2800000000000000266, 0.2999999999999999889, 0.3200000000000000067, 0.3400000000000000244, 0.3599999999999999867, 0.3799999999999999489, 0.4000000000000000222, 0.4199999999999999845, 0.4400000000000000022, 0.4600000000000000200, 0.4799999999999999267, 0.5000000000000000000, 0.5200000000000000178, 0.5400000000000000355, 0.5600000000000000533, 0.5799999999999999600, 0.5999999999999999778, 0.6199999999999999956, 0.6400000000000000133, 0.6600000000000000311, 0.6800000000000000488, 0.6875575298689686754 ),
 .UNSPECIFIED. ) 
 CURVE ( )  GEOMETRIC_REPRESENTATION_ITEM ( )  RATIONAL_B_SPLINE_CURVE ( ( 1.000000000000000000, 0.9510565162951535312, 1.000000000000000000, 0.9510565162951535312, 1.000000000000000000, 0.9510565162951535312, 1.000000000000000000, 0.9510565162951535312, 1.000000000000000000, 0.9510565162951535312, 1.000000000000000000, 0.9510565162951535312, 1.000000000000000000, 0.9510565162951535312, 1.000000000000000000, 0.9510565162951535312, 1.000000000000000000, 0.9510565162951535312, 1.000000000000000000, 0.9510565162951535312, 1.000000000000000000, 0.9510565162951535312, 1.000000000000000000, 0.9510565162951535312, 1.000000000000000000, 0.9510565162951535312, 1.000000000000000000, 0.9510565162951535312, 1.000000000000000000, 0.9510565162951535312, 1.000000000000000000, 0.9510565162951535312, 1.000000000000000000, 0.9510565162951535312, 1.000000000000000000, 0.9510565162951535312, 1.000000000000000000, 0.9510565162951535312, 1.000000000000000000, 0.9510565162951535312, 1.000000000000000000, 0.9510565162951535312, 1.000000000000000000, 0.9510565162951535312, 1.000000000000000000, 0.9510565162951535312, 1.000000000000000000, 0.9510565162951535312, 1.000000000000000000, 0.9510565162951535312, 1.000000000000000000, 0.9510565162951535312, 1.000000000000000000, 0.9510565162951535312, 1.000000000000000000, 0.9510565162951535312, 1.000000000000000000, 0.9510565162951535312, 1.000000000000000000, 0.9510565162951535312, 1.000000000000000000, 0.9510565162951535312, 1.000000000000000000, 0.9510565162951535312, 1.000000000000000000, 0.9510565162951535312, 1.000000000000000000, 0.9510565162951535312, 1.000000000000000000, 0.9815054080004621540, 0.9769881591460138903 ) ) 
 REPRESENTATION_ITEM ( '' )  );
#168447=EDGE_CURVE ( 'NONE', #147006, #65515, #140986, .T. ) ;
#168491=CARTESIAN_POINT ( 'NONE',  ( 11.40812507854755253, -35.11059874428192273, -2.024999997268813079 ) ) ;
#168572=CARTESIAN_POINT ( 'NONE',  ( -36.95458794302616212, -5.320992724678917263, 43.56214547691710237 ) ) ;
#168601=CARTESIAN_POINT ( 'NONE',  ( 27.73933785331498214, 9.013057229001095294, 146.4750000027311501 ) ) ;
#168624=CARTESIAN_POINT ( 'NONE',  ( -35.50084720355936696, 3.323798168015720034, 38.27222404303020653 ) ) ;
#168639=EDGE_CURVE ( 'NONE', #189747, #130647, #2283, .T. ) ;
#168659=VERTEX_POINT ( 'NONE', #178469 ) ;
#168711=CARTESIAN_POINT ( 'NONE',  ( -17.14385361876520975, 23.59649016807275856, 148.5750000027311728 ) ) ;
#168728=CARTESIAN_POINT ( 'NONE',  ( 37.99626262588765258, 2.893932880411085066E-14, -7.002157773949822861 ) ) ;
#168835=CARTESIAN_POINT ( 'NONE',  ( -36.91746825000001309, -11.99521256947794789, -7.024999997268812635 ) ) ;
#168838=CARTESIAN_POINT ( 'NONE',  ( 37.99626262588765258, 2.893932880411085066E-14, -2.747842220587803475 ) ) ;
#168841=CARTESIAN_POINT ( 'NONE',  ( 33.79632059884288964, 5.461862605997787057, 94.26112944759007917 ) ) ;
#168862=CARTESIAN_POINT ( 'NONE',  ( -32.00000000000000000, -5.510910596163089556E-15, 45.00000000000000000 ) ) ;
#168875=CARTESIAN_POINT ( 'NONE',  ( -31.51098639601627838, -4.378554692192621722, 101.0941514966583412 ) ) ;
#168927=CARTESIAN_POINT ( 'NONE',  ( -8.906447517083053711, -27.41122689804191026, 142.6500000054623740 ) ) ;
#168938=CARTESIAN_POINT ( 'NONE',  ( -31.27056374934903715, 7.502136971886772088, 95.45648825569139717 ) ) ;
#169023=CARTESIAN_POINT ( 'NONE',  ( -22.81625015709510507, 31.40387420917330275, -3.424999997268813434 ) ) ;
#169034=ORIENTED_EDGE ( 'NONE', *, *, #108503, .T. ) ;
#169059=AXIS2_PLACEMENT_3D ( 'NONE', #117158, #28176, #194025 ) ;
#169116=CARTESIAN_POINT ( 'NONE',  ( -27.73933785331498925, 9.013057229001089965, 148.7750000027311899 ) ) ;
#169145=AXIS2_PLACEMENT_3D ( 'NONE', #129177, #113024, #143352 ) ;
#169155=EDGE_LOOP ( 'NONE', ( #170588, #120557, #15618, #83108, #180810 ) ) ;
#169215=CARTESIAN_POINT ( 'NONE',  ( 32.00000000000000000, -1.163414459189985801E-14, 89.49999999999897682 ) ) ;
#169216=CARTESIAN_POINT ( 'NONE',  ( 28.82186960331498327, 2.781578969918950771E-14, 139.2500000054623683 ) ) ;
#169233=FACE_OUTER_BOUND ( 'NONE', #27598, .T. ) ;
#169285=CARTESIAN_POINT ( 'NONE',  ( 35.50084720355934564, 3.323798168015733800, 38.27222404303021364 ) ) ;
#169393=TOROIDAL_SURFACE ( 'NONE', #33725, 2.700000000000000622, 0.2000000000000000111 ) ;
#169429=ORIENTED_EDGE ( 'NONE', *, *, #93300, .T. ) ;
#169480=CARTESIAN_POINT ( 'NONE',  ( -11.40812507854755609, 35.11059874428196537, -1.024999997268813301 ) ) ;
#169531=CIRCLE ( 'NONE', #75858, 40.00000000000002132 ) ;
#169553=PRODUCT_DEFINITION_FORMATION_WITH_SPECIFIED_SOURCE ( 'ANY', '', #29103, .NOT_KNOWN. ) ;
#169571=CARTESIAN_POINT ( 'NONE',  ( -36.81794758165438708, -5.500929263287721582, 45.34431116311557020 ) ) ;
#169601=CARTESIAN_POINT ( 'NONE',  ( -17.14385361876520619, 23.59649016807275856, 143.0750000027311444 ) ) ;
#169627=CARTESIAN_POINT ( 'NONE',  ( -35.59978325014670730, 2.421353778481746044, 37.88472941744216627 ) ) ;
#169649=CARTESIAN_POINT ( 'NONE',  ( -30.73962218707677962, -22.33364281372842441, -7.547842220587804185 ) ) ;
#169681=VECTOR ( 'NONE', #56733, 1000.000000000000000 ) ;
#169717=CARTESIAN_POINT ( 'NONE',  ( -27.73933785331498925, 9.013057229001088189, 142.7750000027311899 ) ) ;
#169732=CARTESIAN_POINT ( 'NONE',  ( 23.48298174826589246, 32.32155151706776053, -4.447842220587801876 ) ) ;
#169778=EDGE_CURVE ( 'NONE', #11483, #85078, #101047, .T. ) ;
#169799=CYLINDRICAL_SURFACE ( 'NONE', #157591, 2.649999999999992806 ) ;
#169842=CARTESIAN_POINT ( 'NONE',  ( 22.81625015709510151, -31.40387420917324590, -10.42499999726881477 ) ) ;
#169843=CARTESIAN_POINT ( 'NONE',  ( -34.42157296979473813, 2.272259278789487968, 89.98812102125175727 ) ) ;
#169848=CARTESIAN_POINT ( 'NONE',  ( 34.37139930337509952, 2.751904643975405573, 90.23455903727463578 ) ) ;
#169860=CARTESIAN_POINT ( 'NONE',  ( 36.91746824999999177, 11.99521256947799230, -6.024999997268812635 ) ) ;
#169870=EDGE_CURVE ( 'NONE', #81412, #191417, #54864, .T. ) ;
#169902=CARTESIAN_POINT ( 'NONE',  ( -28.82186960331499037, 2.428612866367529932E-14, 148.2500000054623683 ) ) ;
#169947=CARTESIAN_POINT ( 'NONE',  ( -31.54545164052522566, 7.106679946642016077, 92.55365670706888181 ) ) ;
#169979=EDGE_CURVE ( 'NONE', #50285, #48134, #131707, .T. ) ;
#170034=CARTESIAN_POINT ( 'NONE',  ( -5.950531402560715689E-15, 38.81732327939063509, -9.624999997268815832 ) ) ;
#170051=ORIENTED_EDGE ( 'NONE', *, *, #104283, .F. ) ;
#170053=LINE ( 'NONE', #91196, #79116 ) ;
#170116=CARTESIAN_POINT ( 'NONE',  ( 37.99626262588765258, 2.893932880411085066E-14, -5.002157773949823749 ) ) ;
#170121=CARTESIAN_POINT ( 'NONE',  ( -17.14385361876520619, 23.59649016807275856, 144.5750000027312012 ) ) ;
#170159=VERTEX_POINT ( 'NONE', #169902 ) ;
#170288=CARTESIAN_POINT ( 'NONE',  ( 34.72612402863278191, 2.419136457854856204, 52.10344399403046367 ) ) ;
#170447=CARTESIAN_POINT ( 'NONE',  ( 34.51794252349512249, -0.7246179257117796313, 89.53606970770105988 ) ) ;
#170481=CARTESIAN_POINT ( 'NONE',  ( -29.86685920354755552, 21.69954338932564397, -0.8249999972688133454 ) ) ;
#170571=CARTESIAN_POINT ( 'NONE',  ( -36.86570815857407979, -2.439361326604243096, 49.93277065412546278 ) ) ;
#170588=ORIENTED_EDGE ( 'NONE', *, *, #141481, .T. ) ;
#170602=CARTESIAN_POINT ( 'NONE',  ( 27.73933785331498925, -9.013057229001033122, 142.2750000027311899 ) ) ;
#170627=CARTESIAN_POINT ( 'NONE',  ( -17.81289503416611808, 24.51734667627700404, 147.9500000054623570 ) ) ;
#170715=CARTESIAN_POINT ( 'NONE',  ( 22.44159573604009239, 16.30477369853692693, 146.0750000027311728 ) ) ;
#170842=CARTESIAN_POINT ( 'NONE',  ( 29.86685920354754487, 21.69954338932564752, -1.424999997268813212 ) ) ;
#170843=CARTESIAN_POINT ( 'NONE',  ( -34.52594549653173317, 2.005792002353502844E-14, 89.49999999999897682 ) ) ;
#170847=DIRECTION ( 'NONE',  ( -1.000000000000000000, -0.000000000000000000, -0.000000000000000000 ) ) ;
#170890=CARTESIAN_POINT ( 'NONE',  ( 34.37176626784628297, -7.314009959508099179, 46.67821535514400466 ) ) ;
#170895=CARTESIAN_POINT ( 'NONE',  ( -3.573655867282028392E-15, 2.428612866367529932E-14, 139.9999999999999716 ) ) ;
#170919=CARTESIAN_POINT ( 'NONE',  ( -8.906447517083060816, 27.41122689804195645, 141.5999999999999943 ) ) ;
#170983=CARTESIAN_POINT ( 'NONE',  ( -37.99626262588766679, 2.428612866367529932E-14, 2.000000000000000000 ) ) ;
#170993=CARTESIAN_POINT ( 'NONE',  ( -36.91128768240056246, 1.976579976310101802E-14, 50.50000000000002842 ) ) ;
#171030=CARTESIAN_POINT ( 'NONE',  ( 11.40812507854755253, -35.11059874428192273, -4.524999997268813523 ) ) ;
#171081=CARTESIAN_POINT ( 'NONE',  ( -28.82186960331499037, 2.428612866367529617E-14, 146.2500000054623683 ) ) ;
#171088=CARTESIAN_POINT ( 'NONE',  ( 31.79999999999934346, 1.011436372600181938E-12, 95.00000000000021316 ) ) ;
#171099=VERTEX_POINT ( 'NONE', #141313 ) ;
#171119=CARTESIAN_POINT ( 'NONE',  ( -22.44159573604009950, -16.30477369853688430, 139.0750000027311728 ) ) ;
#171157=ORIENTED_EDGE ( 'NONE', *, *, #89680, .T. ) ;
#171253=EDGE_CURVE ( 'NONE', #89861, #191417, #5133, .T. ) ;
#171294=CIRCLE ( 'NONE', #158300, 28.82186960331498682 ) ;
#171446=CARTESIAN_POINT ( 'NONE',  ( 33.90027759800518936, -5.214635694306275049, 93.21535130585120044 ) ) ;
#171479=CARTESIAN_POINT ( 'NONE',  ( 36.91746824999999887, 11.99521256947799053, -3.524999997268813079 ) ) ;
#171492=EDGE_CURVE ( 'NONE', #54169, #34628, #99262, .T. ) ;
#171568=CARTESIAN_POINT ( 'NONE',  ( -36.77186724307693311, -4.769522647520278547, 47.74487706083468197 ) ) ;
#171598=CARTESIAN_POINT ( 'NONE',  ( 23.31738231874054534, 16.94106989632529192, 149.1999999999999886 ) ) ;
#171622=CARTESIAN_POINT ( 'NONE',  ( -23.31738231874055245, -16.94106989632524574, 146.4500000054623854 ) ) ;
#171641=CARTESIAN_POINT ( 'NONE',  ( 37.99626262588760994, -12.34573411038917357, -6.847842220587804007 ) ) ;
#171712=CARTESIAN_POINT ( 'NONE',  ( 1.784210473542230573E-15, -29.16686587814331588, 145.3750000027311842 ) ) ;
#171730=CARTESIAN_POINT ( 'NONE',  ( -28.82186960331499037, 2.428612866367530248E-14, 142.2500000054623683 ) ) ;
#171792=CARTESIAN_POINT ( 'NONE',  ( 37.87393738558668588, 2.428612866367529932E-14, 2.000000000000000000 ) ) ;
#171836=CARTESIAN_POINT ( 'NONE',  ( -11.40812507854755609, 35.11059874428196537, -7.024999997268813523 ) ) ;
#171853=CARTESIAN_POINT ( 'NONE',  ( -22.81625015709510507, 31.40387420917330275, -7.424999997268812102 ) ) ;
#171915=DIRECTION ( 'NONE',  ( 0.000000000000000000, 0.000000000000000000, -1.000000000000000000 ) ) ;
#171926=CARTESIAN_POINT ( 'NONE',  ( -31.72709406046301339, 2.040068635034919209E-14, 102.5000000000000142 ) ) ;
#171946=CARTESIAN_POINT ( 'NONE',  ( 30.00000000000000000, 40.00100000000004741, 37.49999999999999289 ) ) ;
#172023=CARTESIAN_POINT ( 'NONE',  ( 11.40812507854754365, 35.11059874428196537, -3.724999997268813701 ) ) ;
#172075=CARTESIAN_POINT ( 'NONE',  ( 28.82186960331518222, 9.364793116373306248, 143.0999999999999943 ) ) ;
#172087=CARTESIAN_POINT ( 'NONE',  ( 23.48298174826590667, -32.32155151706770368, -7.302157773949821795 ) ) ;
#172112=CARTESIAN_POINT ( 'NONE',  ( -27.73933785331498925, 9.013057229001089965, 142.7750000027311899 ) ) ;
#172117=CARTESIAN_POINT ( 'NONE',  ( -17.14385361876520619, 23.59649016807275856, 140.5750000027311728 ) ) ;
#172159=CIRCLE ( 'NONE', #1105, 7.500000000000007105 ) ;
#172184=CARTESIAN_POINT ( 'NONE',  ( 8.571926809382597767, 26.38167802310806209, 144.7750000027311899 ) ) ;
#172224=CARTESIAN_POINT ( 'NONE',  ( -6.020228577223754586E-15, 39.95556452105416412, -8.500000000000001776 ) ) ;
#172313=CARTESIAN_POINT ( 'NONE',  ( -35.68964480816960361, -0.9792624367684957809, 37.54765762180190336 ) ) ;
#172345=CARTESIAN_POINT ( 'NONE',  ( 36.91746824999999177, 2.880721459617395097E-14, -1.624999997268813390 ) ) ;
#172412=VERTEX_POINT ( 'NONE', #96768 ) ;
#172436=CARTESIAN_POINT ( 'NONE',  ( 33.80700117934222249, -2.275881256356157234, 100.0103016164005254 ) ) ;
#172470=CARTESIAN_POINT ( 'NONE',  ( -36.91746825000001309, 11.99521256947798342, -2.724999997268813701 ) ) ;
#172483=VECTOR ( 'NONE', #189250, 1000.000000000000000 ) ;
#172562=CARTESIAN_POINT ( 'NONE',  ( -23.48298174826590667, 32.32155151706776053, -6.047842220587802409 ) ) ;
#172563=CARTESIAN_POINT ( 'NONE',  ( 32.45678934495597900, -3.100610132747068093, 88.16656412605026105 ) ) ;
#172592=CARTESIAN_POINT ( 'NONE',  ( 27.73933785331498214, 9.013057229001095294, 140.4750000027311785 ) ) ;
#172615=CARTESIAN_POINT ( 'NONE',  ( 17.14385361876520264, 23.59649016807275856, 148.1750000027311955 ) ) ;
#172618=AXIS2_PLACEMENT_3D ( 'NONE', #155743, #20209, #171915 ) ;
#172708=CARTESIAN_POINT ( 'NONE',  ( 1.784210473542230573E-15, -29.16686587814331588, 141.3750000027311557 ) ) ;
#172836=CARTESIAN_POINT ( 'NONE',  ( -36.91746825000001309, -11.99521256947794789, -4.524999997268813523 ) ) ;
#172891=CARTESIAN_POINT ( 'NONE',  ( 35.09697802211634610, -5.650142709571455590, 40.04346530744799537 ) ) ;
#172899=ORIENTED_EDGE ( 'NONE', *, *, #13466, .T. ) ;
#172912=ORIENTED_EDGE ( 'NONE', *, *, #1987, .F. ) ;
#172916=CARTESIAN_POINT ( 'NONE',  ( -6.019987952026120409E-15, 39.95163481335720235, -4.502157773949821973 ) ) ;
#172922=CARTESIAN_POINT ( 'NONE',  ( 17.81289503416610742, 24.51734667627700404, 141.3000000000000114 ) ) ;
#173045=EDGE_LOOP ( 'NONE', ( #7202, #196214, #161469, #66335 ) ) ;
#173072=DIRECTION ( 'NONE',  ( 0.000000000000000000, 0.000000000000000000, -1.000000000000000000 ) ) ;
#173079=CYLINDRICAL_SURFACE ( 'NONE', #146899, 5.500000000000032863 ) ;
#173091=CARTESIAN_POINT ( 'NONE',  ( 30.73962218707677962, -22.33364281372841376, -7.202157773949823927 ) ) ;
#173117=CARTESIAN_POINT ( 'NONE',  ( 17.14385361876520264, -23.59649016807271238, 139.5750000027311444 ) ) ;
#173187=CARTESIAN_POINT ( 'NONE',  ( -27.73933785331498925, 9.013057229001088189, 147.2750000027311614 ) ) ;
#173318=CARTESIAN_POINT ( 'NONE',  ( -35.41276914313063173, -3.966036006072681364, 38.62970943314355310 ) ) ;
#173352=CARTESIAN_POINT ( 'NONE',  ( -36.91746825000000598, -11.99521256947794789, -6.524999997268811747 ) ) ;
#173436=CARTESIAN_POINT ( 'NONE',  ( -3.573655867282028392E-15, 2.428612866367529932E-14, 150.0000000000000000 ) ) ;
#173473=CARTESIAN_POINT ( 'NONE',  ( 11.40812507854755253, -35.11059874428192273, -8.024999997268814411 ) ) ;
#173565=CARTESIAN_POINT ( 'NONE',  ( 31.37911219714120037, -7.435064219939697239, 93.98466263399201637 ) ) ;
#173594=CARTESIAN_POINT ( 'NONE',  ( -22.44159573604009950, -16.30477369853688430, 139.5750000027311728 ) ) ;
#173616=CARTESIAN_POINT ( 'NONE',  ( -28.82186960331499392, 9.364793116373565596, 140.1500000054623740 ) ) ;
#173619=VECTOR ( 'NONE', #144993, 1000.000000000000000 ) ;
#173733=CARTESIAN_POINT ( 'NONE',  ( 36.77423900702710569, -4.677204790287845526, 47.89930394225363841 ) ) ;
#173836=CARTESIAN_POINT ( 'NONE',  ( 36.91746824999999177, 2.880721459617395097E-14, -7.624999997268813168 ) ) ;
#173862=ORIENTED_EDGE ( 'NONE', *, *, #59844, .F. ) ;
#173918=FACE_BOUND ( 'NONE', #74971, .T. ) ;
#173949=DIRECTION ( 'NONE',  ( 3.709348145883536076E-20, 0.000000000000000000, -1.000000000000000000 ) ) ;
#174025=CARTESIAN_POINT ( 'NONE',  ( -29.86685920354755197, -21.69954338932560134, -10.92499999726881299 ) ) ;
#174113=CARTESIAN_POINT ( 'NONE',  ( -22.44159573604010305, 16.30477369853692338, 149.1750000027311671 ) ) ;
#174150=CIRCLE ( 'NONE', #35432, 7.500000000000007105 ) ;
#174185=CARTESIAN_POINT ( 'NONE',  ( -22.44159573604009950, -16.30477369853688430, 145.5750000027311728 ) ) ;
#174232=DIRECTION ( 'NONE',  ( -3.709348145883536076E-20, 0.000000000000000000, 1.000000000000000000 ) ) ;
#174263=CARTESIAN_POINT ( 'NONE',  ( 37.99999999999999289, 2.893978650043524126E-14, -4.749999994537627224 ) ) ;
#174310=CARTESIAN_POINT ( 'NONE',  ( 37.07039049082555948, 4.937524616431669067, 42.55055737136174088 ) ) ;
#174313=CARTESIAN_POINT ( 'NONE',  ( -35.09697802211634610, -5.650142709571460031, 40.04346530744797406 ) ) ;
#174343=CARTESIAN_POINT ( 'NONE',  ( -36.91746825000000598, 2.428612866367529932E-14, -2.624999997268813168 ) ) ;
#174394=CARTESIAN_POINT ( 'NONE',  ( -3.573655867282028392E-15, 2.428612866367529932E-14, 0.000000000000000000 ) ) ;
#174430=CARTESIAN_POINT ( 'NONE',  ( 33.79565148458099344, -5.463178417057489966, 94.26852713616585788 ) ) ;
#174458=ORIENTED_EDGE ( 'NONE', *, *, #140456, .T. ) ;
#174463=CARTESIAN_POINT ( 'NONE',  ( -36.91746825000000598, 2.428612866367529932E-14, -6.624999997268814056 ) ) ;
#174476=TOROIDAL_SURFACE ( 'NONE', #19453, 2.700000000000000622, 0.2000000000000000111 ) ;
#174553=CARTESIAN_POINT ( 'NONE',  ( 31.40318257579880523, -7.397807925419288999, 93.74221852110635211 ) ) ;
#174586=CARTESIAN_POINT ( 'NONE',  ( 28.82186960331498327, 9.364793116373570925, 147.0999999999999943 ) ) ;
#174607=CARTESIAN_POINT ( 'NONE',  ( 23.31738231874054890, -16.94106989632523508, 143.0500000054623513 ) ) ;
#174712=CARTESIAN_POINT ( 'NONE',  ( -40.00000000000002842, 1.938754146708588393E-14, 0.000000000000000000 ) ) ;
#174773=CARTESIAN_POINT ( 'NONE',  ( -67.00000000000000000, -1.163414459189985801E-14, 95.00000000000000000 ) ) ;
#174791=CARTESIAN_POINT ( 'NONE',  ( -28.82186960331499037, 2.781578969918950771E-14, 139.9999999999999716 ) ) ;
#174816=CARTESIAN_POINT ( 'NONE',  ( -11.40812507854754720, -35.11059874428192273, -8.224999997268813701 ) ) ;
#174873=CARTESIAN_POINT ( 'NONE',  ( 35.63774670715082493, -1.952809719854257775, 37.74170157406051374 ) ) ;
#175092=CARTESIAN_POINT ( 'NONE',  ( -32.00000000000000000, -4.837354856632041508E-15, 50.50000000000002842 ) ) ;
#175098=CARTESIAN_POINT ( 'NONE',  ( 22.44159573604009239, 16.30477369853692693, 148.5750000027312012 ) ) ;
#175130=DIRECTION ( 'NONE',  ( -6.982962677686266711E-15, 0.000000000000000000, 1.000000000000000000 ) ) ;
#175171=CARTESIAN_POINT ( 'NONE',  ( -17.14385361876520264, -23.59649016807271238, 147.6750000027311671 ) ) ;
#175259=DIRECTION ( 'NONE',  ( -1.000000000000000000, 0.000000000000000000, 0.000000000000000000 ) ) ;
#175300=CARTESIAN_POINT ( 'NONE',  ( 29.86685920354754487, 21.69954338932564752, -5.924999997268813878 ) ) ;
#175318=VERTEX_POINT ( 'NONE', #16222 ) ;
#175332=CARTESIAN_POINT ( 'NONE',  ( -29.86685920354755197, -21.69954338932560134, -4.424999997268812990 ) ) ;
#175448=ORIENTED_EDGE ( 'NONE', *, *, #198419, .T. ) ;
#175453=CARTESIAN_POINT ( 'NONE',  ( 22.81625015709509441, 31.40387420917330275, -7.324999997268812457 ) ) ;
#175525=DIRECTION ( 'NONE',  ( 0.000000000000000000, 0.000000000000000000, -1.000000000000000000 ) ) ;
#175533=LINE ( 'NONE', #100674, #23998 ) ;
#175543=CARTESIAN_POINT ( 'NONE',  ( 31.24012740013091616, -7.112679799535560399, 97.39185870086457442 ) ) ;
#175573=CARTESIAN_POINT ( 'NONE',  ( -17.81289503416611808, 24.51734667627700404, 147.6999999999999886 ) ) ;
#175596=CARTESIAN_POINT ( 'NONE',  ( 28.82186960331499392, -9.364793116373510529, 141.1500000054623740 ) ) ;
#175621=AXIS2_PLACEMENT_3D ( 'NONE', #22537, #82177, #3373 ) ;
#175632=ORIENTED_EDGE ( 'NONE', *, *, #150856, .F. ) ;
#175705=FACE_OUTER_BOUND ( 'NONE', #193284, .T. ) ;
#175707=CARTESIAN_POINT ( 'NONE',  ( 36.89003987753539349, -5.463308683677074562, 44.27017301194418764 ) ) ;
#175744=FACE_OUTER_BOUND ( 'NONE', #101484, .T. ) ;
#175815=CARTESIAN_POINT ( 'NONE',  ( -36.91746825000000598, 2.428612866367529932E-14, -6.624999997268814056 ) ) ;
#175892=DIRECTION ( 'NONE',  ( 0.000000000000000000, -0.000000000000000000, -1.000000000000000000 ) ) ;
#175937=CIRCLE ( 'NONE', #85575, 2.649999999999992806 ) ;
#175994=VERTEX_POINT ( 'NONE', #82838 ) ;
#176019=CARTESIAN_POINT ( 'NONE',  ( 36.91746824999999887, 11.99521256947799053, -10.02499999726881086 ) ) ;
#176023=CYLINDRICAL_SURFACE ( 'NONE', #9083, 28.82186960331498682 ) ;
#176051=EDGE_CURVE ( 'NONE', #134298, #186418, #89762, .T. ) ;
#176105=CARTESIAN_POINT ( 'NONE',  ( -8.571926809382601320, -26.38167802310801591, 145.7750000027311899 ) ) ;
#176125=AXIS2_PLACEMENT_3D ( 'NONE', #67074, #175259, #68068 ) ;
#176156=EDGE_CURVE ( 'NONE', #168659, #60925, #101468, .T. ) ;
#176179=CARTESIAN_POINT ( 'NONE',  ( -8.571926809382601320, -26.38167802310801591, 145.7750000027311899 ) ) ;
#176223=DIRECTION ( 'NONE',  ( -0.06104853953485701173, -7.476289853398329258E-18, -0.9981347984218670311 ) ) ;
#176265=ORIENTED_EDGE ( 'NONE', *, *, #140456, .F. ) ;
#176305=CARTESIAN_POINT ( 'NONE',  ( -30.00000000000000000, -5.510910596163089556E-15, 45.00000000000000000 ) ) ;
#176307=CARTESIAN_POINT ( 'NONE',  ( -5.950531402560715689E-15, 38.81732327939063509, -3.624999997268813168 ) ) ;
#176310=CARTESIAN_POINT ( 'NONE',  ( 32.00000000000000000, -5.510910596163089556E-15, 45.00000000000000000 ) ) ;
#176321=EDGE_CURVE ( 'NONE', #55000, #17723, #157448, .T. ) ;
#176341=CARTESIAN_POINT ( 'NONE',  ( 11.40812507854754365, 35.11059874428196537, -3.224999997268813701 ) ) ;
#176393=FACE_OUTER_BOUND ( 'NONE', #60863, .T. ) ;
#176463=CARTESIAN_POINT ( 'NONE',  ( 11.74264578624799427, 36.14014761921585972, -0.5999999999999999778 ) ) ;
#176507=ORIENTED_EDGE ( 'NONE', *, *, #4359, .F. ) ;
#176527=ORIENTED_EDGE ( 'NONE', *, *, #151903, .T. ) ;
#176569=AXIS2_PLACEMENT_3D ( 'NONE', #67701, #83852, #192049 ) ;
#176586=CARTESIAN_POINT ( 'NONE',  ( -28.82186960331499392, -9.364793116373526516, 144.0999999999999659 ) ) ;
#176609=CARTESIAN_POINT ( 'NONE',  ( -23.31738231874055245, -16.94106989632524574, 142.4500000054623854 ) ) ;
#176636=CARTESIAN_POINT ( 'NONE',  ( 28.82186960331498327, 2.781578969918950771E-14, 147.2500000054623683 ) ) ;
#176704=CARTESIAN_POINT ( 'NONE',  ( -8.571926809382608425, 26.38167802310805854, 140.4750000027312069 ) ) ;
#176779=CARTESIAN_POINT ( 'NONE',  ( 28.82186960331498327, 2.781578969918950771E-14, 145.0000000000000000 ) ) ;
#176811=ORIENTED_EDGE ( 'NONE', *, *, #18367, .T. ) ;
#176832=VERTEX_POINT ( 'NONE', #37344 ) ;
#177031=CARTESIAN_POINT ( 'NONE',  ( 33.13409719347311722, -16.32441212556909349, -7.999999999999998224 ) ) ;
#177040=ORIENTED_EDGE ( 'NONE', *, *, #71047, .T. ) ;
#177116=CARTESIAN_POINT ( 'NONE',  ( -27.73933785331498925, 2.428612866367529932E-14, 141.3750000027311842 ) ) ;
#177147=DIRECTION ( 'NONE',  ( 0.000000000000000000, 0.000000000000000000, 1.000000000000000000 ) ) ;
#177188=CARTESIAN_POINT ( 'NONE',  ( 8.571926809382597767, 26.38167802310806209, 140.7750000027311899 ) ) ;
#177210=CARTESIAN_POINT ( 'NONE',  ( 40.00000000000001421, 2.428612866367529932E-14, 0.000000000000000000 ) ) ;
#177266=CARTESIAN_POINT ( 'NONE',  ( -38.00000000000000711, 2.428612866367529932E-14, -1.749999994537626558 ) ) ;
#177276=CARTESIAN_POINT ( 'NONE',  ( 31.79999999999967031, 4.791014396527177230E-13, 47.70000000000022311 ) ) ;
#177316=CARTESIAN_POINT ( 'NONE',  ( 37.51279278323692523, 1.941191203875218596, 39.85083793614483483 ) ) ;
#177319=CARTESIAN_POINT ( 'NONE',  ( -34.36947210329395119, -7.112397586384673787, 47.39260519897412394 ) ) ;
#177392=ORIENTED_EDGE ( 'NONE', *, *, #153999, .F. ) ;
#177469=CARTESIAN_POINT ( 'NONE',  ( 29.86685920354754842, -21.69954338932559068, -7.824999997268813345 ) ) ;
#177539=EDGE_CURVE ( 'NONE', #68554, #129957, #151128, .T. ) ;
#177581=DIRECTION ( 'NONE',  ( 1.000000000000000000, -0.000000000000000000, 6.982962677686266711E-15 ) ) ;
#177652=VERTEX_POINT ( 'NONE', #146512 ) ;
#177696=EDGE_CURVE ( 'NONE', #83841, #139003, #131611, .T. ) ;
#177699=ORIENTED_EDGE ( 'NONE', *, *, #68776, .F. ) ;
#177702=CARTESIAN_POINT ( 'NONE',  ( 17.14385361876520264, 23.59649016807275856, 140.1750000027311671 ) ) ;
#177719=CARTESIAN_POINT ( 'NONE',  ( 36.86570815857407268, -2.439361326604236879, 49.93277065412544857 ) ) ;
#177790=CARTESIAN_POINT ( 'NONE',  ( 22.93331243197825131, 29.30057843794256911, -8.000000000000003553 ) ) ;
#177793=CARTESIAN_POINT ( 'NONE',  ( 28.82186960331498327, 2.781578969918950771E-14, 145.0000000000000000 ) ) ;
#177820=CARTESIAN_POINT ( 'NONE',  ( 27.73933785331498569, 2.768321779492822058E-14, 148.3750000027311842 ) ) ;
#177865=CYLINDRICAL_SURFACE ( 'NONE', #73392, 7.500000000000007105 ) ;
#177881=CARTESIAN_POINT ( 'NONE',  ( -3.573655867282028392E-15, 2.428612866367529932E-14, 6.432029388270255055E-14 ) ) ;
#177897=DIRECTION ( 'NONE',  ( 0.000000000000000000, 0.000000000000000000, -1.000000000000000000 ) ) ;
#178020=CARTESIAN_POINT ( 'NONE',  ( 27.79211460164531999, -24.33005135171561051, -8.000000000000005329 ) ) ;
#178068=CARTESIAN_POINT ( 'NONE',  ( -33.86249154851668663, -5.319940558880595027, 93.55791698674944712 ) ) ;
#178069=CARTESIAN_POINT ( 'NONE',  ( 37.99626262588765258, -12.34573411038911672, -1.102157773949822506 ) ) ;
#178103=CARTESIAN_POINT ( 'NONE',  ( -31.91599925174812213, -5.957486376704252962, 90.41819350476903594 ) ) ;
#178107=CARTESIAN_POINT ( 'NONE',  ( -22.44159573604009950, -16.30477369853688430, 143.5750000027311728 ) ) ;
#178113=CARTESIAN_POINT ( 'NONE',  ( 3.765340386950246872E-15, -39.95163481335715971, -5.247842220587802586 ) ) ;
#178148=EDGE_CURVE ( 'NONE', #193619, #46374, #192517, .T. ) ;
#178194=CYLINDRICAL_SURFACE ( 'NONE', #141973, 5.500000000000032863 ) ;
#178260=CARTESIAN_POINT ( 'NONE',  ( 29.86685920354754842, -21.69954338932559068, -2.324999997268813345 ) ) ;
#178312=CARTESIAN_POINT ( 'NONE',  ( -34.40547513665163848, -6.508760260264954134, 48.73452191691475832 ) ) ;
#178328=ORIENTED_EDGE ( 'NONE', *, *, #171492, .F. ) ;
#178419=CARTESIAN_POINT ( 'NONE',  ( -37.99626262588766679, 2.428612866367529932E-14, -7.747842220587803475 ) ) ;
#178442=( BOUNDED_CURVE ( )  B_SPLINE_CURVE ( 2, ( #104094, #165777, #88920, #150612, #12108, #73771, #108047, #169732, #93879, #200078, #31227 ),
 .UNSPECIFIED., .F., .T. ) 
 B_SPLINE_CURVE_WITH_KNOTS ( ( 3, 2, 2, 2, 2, 3 ),
 ( 0.2000000000000000111, 0.2200000000000000289, 0.2400000000000000466, 0.2600000000000000644, 0.2800000000000001377, 0.3000000000000000999 ),
 .UNSPECIFIED. ) 
 CURVE ( )  GEOMETRIC_REPRESENTATION_ITEM ( )  RATIONAL_B_SPLINE_CURVE ( ( 1.000000000000000000, 0.9510565162951535312, 1.000000000000000000, 0.9510565162951535312, 1.000000000000000000, 0.9510565162951535312, 1.000000000000000000, 0.9510565162951535312, 1.000000000000000000, 0.9510565162951533091, 1.000000000000000222 ) ) 
 REPRESENTATION_ITEM ( '' )  );
#178463=CARTESIAN_POINT ( 'NONE',  ( -30.74264578624800492, -22.33583958711396278, -5.800000000000000711 ) ) ;
#178469=CARTESIAN_POINT ( 'NONE',  ( 35.70266437024449147, 2.428612576286966776E-14, 37.50000000000000000 ) ) ;
#178620=AXIS2_PLACEMENT_3D ( 'NONE', #68738, #102084, #56587 ) ;
#178647=ORIENTED_EDGE ( 'NONE', *, *, #112783, .F. ) ;
#178682=VECTOR ( 'NONE', #167615, 1000.000000000000000 ) ;
#178712=EDGE_CURVE ( 'NONE', #142504, #153137, #121634, .T. ) ;
#178790=CARTESIAN_POINT ( 'NONE',  ( 32.91334004812880920, 16.89252633786550817, -8.000000000000000000 ) ) ;
#178793=CARTESIAN_POINT ( 'NONE',  ( 17.81289503416611453, -24.51734667627695785, 144.6999999999999886 ) ) ;
#178834=EDGE_CURVE ( 'NONE', #44725, #15991, #58977, .T. ) ;
#178844=CARTESIAN_POINT ( 'NONE',  ( -34.59574315510281650, 4.379613810579283673, 51.09339236891209168 ) ) ;
#178847=ADVANCED_FACE ( 'NONE', ( #197509 ), #39820, .F. ) ;
#178956=CARTESIAN_POINT ( 'NONE',  ( 37.99626262588756731, 12.34573411038929436, -2.902157773949821884 ) ) ;
#179075=LINE ( 'NONE', #102215, #159721 ) ;
#179078=CARTESIAN_POINT ( 'NONE',  ( -13.41967750377774848, -34.84915157265046304, -8.000000000000001776 ) ) ;
#179082=AXIS2_PLACEMENT_3D ( 'NONE', #157854, #97146, #7139 ) ;
#179092=CARTESIAN_POINT ( 'NONE',  ( 3.556970738554034288E-15, -38.81732327939057114, -2.624999997268812724 ) ) ;
#179114=CARTESIAN_POINT ( 'NONE',  ( -32.50820986112750433, -2.649538386493586639, 87.97934651352352375 ) ) ;
#179118=CARTESIAN_POINT ( 'NONE',  ( -22.44159573604010305, 16.30477369853692338, 147.1750000027311671 ) ) ;
#179191=CARTESIAN_POINT ( 'NONE',  ( 17.14385361876520264, 23.59649016807275856, 148.1750000027311671 ) ) ;
#179269=CARTESIAN_POINT ( 'NONE',  ( 3.766062262543149401E-15, -39.95556452105413570, -11.24999999453762278 ) ) ;
#179280=( BOUNDED_CURVE ( )  B_SPLINE_CURVE ( 2, ( #187543, #105710, #158166, #34823, #110665, #82294, #52966, #98464, #49010, #67148, #172345, #191488, #141993, #143985, #5466, #128806, #84298, #7459, #188523, #21649, #174343, #69143, #6459, #114643, #190505, #65158, #176341, #18674, #37813, #51979, #50991, #112652, #96478, #50000, #113637, #145977, #142983, #97459, #175332, #111665, #3481, #36799, #99474, #126817, #33834, #159145, #19658, #35813, #160158, #68140, #95494, #127813, #129791, #20641, #83302, #81299, #144979, #161155, #130810, #173352, #22651, #157180, #80320, #4461, #66150, #189518, #195515, #89307, #86311, #40815, #148999, #131823, #146991, #116650, #134837 ),
 .UNSPECIFIED., .F., .F. ) 
 B_SPLINE_CURVE_WITH_KNOTS ( ( 3, 2, 2, 2, 2, 2, 2, 2, 2, 2, 2, 2, 2, 2, 2, 2, 2, 2, 2, 2, 2, 2, 2, 2, 2, 2, 2, 2, 2, 2, 2, 2, 2, 2, 2, 2, 2, 3 ),
 ( 0.000000000000000000, 0.02000000000000000042, 0.04000000000000000083, 0.05999999999999999778, 0.08000000000000000167, 0.1000000000000000056, 0.1199999999999999956, 0.1400000000000000133, 0.1600000000000000033, 0.1799999999999999933, 0.2000000000000000111, 0.2200000000000000011, 0.2399999999999999911, 0.2600000000000000089, 0.2800000000000000266, 0.2999999999999999889, 0.3200000000000000067, 0.3400000000000000244, 0.3599999999999999867, 0.3800000000000000044, 0.4000000000000000222, 0.4199999999999999845, 0.4400000000000000022, 0.4600000000000000200, 0.4799999999999999822, 0.5000000000000000000, 0.5200000000000000178, 0.5400000000000000355, 0.5600000000000000533, 0.5799999999999999600, 0.5999999999999999778, 0.6199999999999999956, 0.6400000000000000133, 0.6600000000000000311, 0.6800000000000000488, 0.6999999999999999556, 0.7199999999999999734, 0.7374174419963606120 ),
 .UNSPECIFIED. ) 
 CURVE ( )  GEOMETRIC_REPRESENTATION_ITEM ( )  RATIONAL_B_SPLINE_CURVE ( ( 1.000000000000000000, 0.9510565162951535312, 1.000000000000000000, 0.9510565162951535312, 1.000000000000000000, 0.9510565162951535312, 1.000000000000000000, 0.9510565162951535312, 1.000000000000000000, 0.9510565162951535312, 1.000000000000000000, 0.9510565162951535312, 1.000000000000000000, 0.9510565162951535312, 1.000000000000000000, 0.9510565162951535312, 1.000000000000000000, 0.9510565162951535312, 1.000000000000000000, 0.9510565162951535312, 1.000000000000000000, 0.9510565162951535312, 1.000000000000000000, 0.9510565162951535312, 1.000000000000000000, 0.9510565162951535312, 1.000000000000000000, 0.9510565162951535312, 1.000000000000000000, 0.9510565162951535312, 1.000000000000000000, 0.9510565162951535312, 1.000000000000000000, 0.9510565162951535312, 1.000000000000000000, 0.9510565162951535312, 1.000000000000000000, 0.9510565162951535312, 1.000000000000000000, 0.9510565162951535312, 1.000000000000000000, 0.9510565162951535312, 1.000000000000000000, 0.9510565162951535312, 1.000000000000000000, 0.9510565162951535312, 1.000000000000000000, 0.9510565162951535312, 1.000000000000000000, 0.9510565162951535312, 1.000000000000000000, 0.9510565162951535312, 1.000000000000000000, 0.9510565162951535312, 1.000000000000000000, 0.9510565162951535312, 1.000000000000000000, 0.9510565162951535312, 1.000000000000000000, 0.9510565162951535312, 1.000000000000000000, 0.9510565162951535312, 1.000000000000000000, 0.9510565162951535312, 1.000000000000000000, 0.9510565162951535312, 1.000000000000000000, 0.9510565162951535312, 1.000000000000000000, 0.9510565162951535312, 1.000000000000000000, 0.9510565162951535312, 1.000000000000000000, 0.9573764855735508172, 0.9889922301674735072 ) ) 
 REPRESENTATION_ITEM ( '' )  );
#179306=CARTESIAN_POINT ( 'NONE',  ( 32.57470439124677597, 1.954246231034476811, 87.74243420032607332 ) ) ;
#179313=CARTESIAN_POINT ( 'NONE',  ( 31.33613174426653458, -7.485780765379337787, 94.47638157584336227 ) ) ;
#179320=CARTESIAN_POINT ( 'NONE',  ( 36.89064505505185565, 5.462148823192609193, 44.26314855211815313 ) ) ;
#179368=DIRECTION ( 'NONE',  ( -0.000000000000000000, -0.000000000000000000, 1.000000000000000000 ) ) ;
#179434=DIRECTION ( 'NONE',  ( 0.000000000000000000, 0.000000000000000000, -1.000000000000000000 ) ) ;
#179464=ORIENTED_EDGE ( 'NONE', *, *, #39318, .T. ) ;
#179476=CARTESIAN_POINT ( 'NONE',  ( 38.00000000000000000, 12.34694845685046616, -4.900000000000000355 ) ) ;
#179521=ORIENTED_EDGE ( 'NONE', *, *, #69397, .T. ) ;
#179593=CARTESIAN_POINT ( 'NONE',  ( -8.906447517083053711, -27.41122689804191026, 142.4000000000000057 ) ) ;
#179627=FILL_AREA_STYLE ('',( #87587 ) ) ;
#179710=EDGE_CURVE ( 'NONE', #9032, #1947, #145754, .T. ) ;
#179727=CARTESIAN_POINT ( 'NONE',  ( 37.42090987696015247, -2.907880681671514367, 40.32815749938561112 ) ) ;
#179764=LINE ( 'NONE', #42236, #114970 ) ;
#179799=CARTESIAN_POINT ( 'NONE',  ( 31.44458473636817075, 19.57661126282215491, -8.000000000000001776 ) ) ;
#179852=CARTESIAN_POINT ( 'NONE',  ( -34.72612402863279613, 2.419136457854829558, 52.10344399403046367 ) ) ;
#179966=CARTESIAN_POINT ( 'NONE',  ( -6.019987952026120409E-15, 39.95163481335720235, -2.502157773949823305 ) ) ;
#180038=DIRECTION ( 'NONE',  ( 0.000000000000000000, 0.000000000000000000, 1.000000000000000000 ) ) ;
#180048=ORIENTED_EDGE ( 'NONE', *, *, #193551, .T. ) ;
#180079=CARTESIAN_POINT ( 'NONE',  ( 11.40812507854754365, 35.11059874428196537, -1.724999997268813479 ) ) ;
#180087=CARTESIAN_POINT ( 'NONE',  ( 3.765340386950246872E-15, -39.95163481335715971, -1.502157773949822639 ) ) ;
#180099=CARTESIAN_POINT ( 'NONE',  ( -36.91746825000000598, -11.99521256947794789, -3.024999997268813079 ) ) ;
#180121=CARTESIAN_POINT ( 'NONE',  ( -31.28611164036841785, -6.519914617504969812, 98.73992561365416520 ) ) ;
#180125=CARTESIAN_POINT ( 'NONE',  ( 8.571926809382597767, 26.38167802310806209, 146.7750000027311899 ) ) ;
#180147=VECTOR ( 'NONE', #179368, 1000.000000000000000 ) ;
#180157=CARTESIAN_POINT ( 'NONE',  ( -8.906447517083060816, 27.41122689804195645, 139.8500000054623911 ) ) ;
#180170=CARTESIAN_POINT ( 'NONE',  ( -28.82186960331499037, 2.428612866367529932E-14, 142.2500000054623683 ) ) ;
#180173=VECTOR ( 'NONE', #36176, 1000.000000000000114 ) ;
#180197=CARTESIAN_POINT ( 'NONE',  ( -27.73933785331498925, -9.013057229001049109, 141.4750000027312069 ) ) ;
#180270=CARTESIAN_POINT ( 'NONE',  ( 11.40812507854755253, -35.11059874428192273, -2.524999997268813523 ) ) ;
#180309=CARTESIAN_POINT ( 'NONE',  ( 32.36630342937671401, 3.758454152357569633, 88.50505952879542804 ) ) ;
#180353=CARTESIAN_POINT ( 'NONE',  ( -37.52489844900624405, 1.772207303729224970, 39.79021962610335095 ) ) ;
#180359=ADVANCED_FACE ( 'NONE', ( #133499 ), #176023, .F. ) ;
#180365=CARTESIAN_POINT ( 'NONE',  ( 27.73933785331498925, -9.013057229001033122, 145.7750000027311899 ) ) ;
#180431=FACE_OUTER_BOUND ( 'NONE', #155538, .T. ) ;
#180435=EDGE_CURVE ( 'NONE', #21447, #43523, #192787, .T. ) ;
#180436=CARTESIAN_POINT ( 'NONE',  ( -31.26591117326541536, 6.741338443544420578, 98.29621977100285335 ) ) ;
#180473=VERTEX_POINT ( 'NONE', #90950 ) ;
#180479=CARTESIAN_POINT ( 'NONE',  ( -38.00000000000000711, 2.428612866367529932E-14, -4.000000000000000000 ) ) ;
#180482=DIRECTION ( 'NONE',  ( 0.000000000000000000, 1.000000000000000000, 0.000000000000000000 ) ) ;
#180594=CARTESIAN_POINT ( 'NONE',  ( -23.31738231874055245, -16.94106989632524574, 142.1999999999999886 ) ) ;
#180629=DIRECTION ( 'NONE',  ( 1.000000000000000000, -0.000000000000000000, -0.000000000000000000 ) ) ;
#180724=CARTESIAN_POINT ( 'NONE',  ( -30.73962218707678318, 22.33364281372846705, -7.947842220587803652 ) ) ;
#180794=FACE_OUTER_BOUND ( 'NONE', #31630, .T. ) ;
#180797=DIRECTION ( 'NONE',  ( 1.000000000000000000, 0.000000000000000000, 0.000000000000000000 ) ) ;
#180810=ORIENTED_EDGE ( 'NONE', *, *, #158766, .F. ) ;
#180829=DIRECTION ( 'NONE',  ( -1.000000000000000000, 0.000000000000000000, -6.982962677686266711E-15 ) ) ;
#180847=CARTESIAN_POINT ( 'NONE',  ( -34.37196153507748164, 7.030587757552860140, 47.62314794725694611 ) ) ;
#181060=CIRCLE ( 'NONE', #16348, 35.99626262588765258 ) ;
#181061=DIRECTION ( 'NONE',  ( 0.000000000000000000, 0.000000000000000000, 1.000000000000000000 ) ) ;
#181067=CARTESIAN_POINT ( 'NONE',  ( -22.81625015709510507, 31.40387420917330275, -3.424999997268813434 ) ) ;
#181074=CARTESIAN_POINT ( 'NONE',  ( -35.81018071281594217, -12.25470802944819937, -7.999999999999998224 ) ) ;
#181108=CARTESIAN_POINT ( 'NONE',  ( -31.99650548583506193, -5.647492055662677757, 90.04056618753070040 ) ) ;
#181182=CARTESIAN_POINT ( 'NONE',  ( 28.82186960331498327, 2.781578969918950771E-14, 141.2500000054623683 ) ) ;
#181205=ADVANCED_FACE ( 'NONE', ( #44483 ), #169799, .F. ) ;
#181258=CARTESIAN_POINT ( 'NONE',  ( -36.91746825000000598, 2.428612866367529932E-14, -1.124999997268813390 ) ) ;
#181273=EDGE_LOOP ( 'NONE', ( #53281, #21832, #39551, #85416 ) ) ;
#181351=CARTESIAN_POINT ( 'NONE',  ( 22.44159573604009239, 16.30477369853692693, 146.0750000027311728 ) ) ;
#181391=( BOUNDED_SURFACE ( )  B_SPLINE_SURFACE ( 1, 2, ( 
 ( #59456, #74645, #155454, #170627, #1764, #107940, #121130, #186815, #109940, #106951, #91765, #140271, #105965, #90783, #139283, #60447, #167650, #93773, #171622, #185803, #29146, #198980, #151490, #154461, #184798, #199976, #138295, #152467, #30124, #122122, #12981, #760, #16944, #13953, #197986, #78598, #153460, #63441, #136311, #31123, #123113, #76617, #137299, #92771, #62431, #124103, #47290, #32116, #125117, #48285, #128078, #94766, #174607, #188789, #50272, #145245, #6726, #126106, #176609, #189781, #52241, #111930, #20907, #34103, #95760, #82566, #144247, #110929, #51253, #191756, #21914, #175596, #130056, #129065, #37072, #159412, #156448, #112913, #127081, #98732, #97722, #173616, #36073, #35086, #5731, #83566, #65420, #68404, #187802, #190766, #67410, #141270, #17948, #157445, #113898, #160425, #53239, #18940, #158428, #114916, #96739 ),
 ( #79601, #2760, #19916, #64436, #4727, #49271, #81558, #172615, #80585, #142259, #3743, #143244, #66417, #74164, #26673, #166177, #122624, #150002, #146239, #161423, #44806, #59963, #91269, #135836, #10499, #76121, #199483, #134850, #181351, #29636, #133835, #180365, #105479, #11508, #72160, #183325, #60949, #75136, #195526, #88314, #38083, #43816, #197505, #89318, #27678, #41833, #196528, #73179, #99739, #167166, #106461, #56999, #84561, #168140, #42830, #152960, #22915, #58972, #151011, #104495, #118674, #103501, #165178, #57999, #12502, #120640, #119669, #14458, #182338, #28665, #90300, #151985, #13473, #137799, #136806, #198490, #121629, #79099, #141765, #1258, #110436, #123605, #185300, #172117, #33603, #268, #140772, #81079, #111434, #64931, #19432, #18446, #126590, #48782, #65918, #2261, #16452, #188292, #187311, #78101, #63944 ) ),
 .UNSPECIFIED., .F., .F., .T. ) 
 B_SPLINE_SURFACE_WITH_KNOTS ( ( 2, 2 ),
 ( 3, 2, 2, 2, 2, 2, 2, 2, 2, 2, 2, 2, 2, 2, 2, 2, 2, 2, 2, 2, 2, 2, 2, 2, 2, 2, 2, 2, 2, 2, 2, 2, 2, 2, 2, 2, 2, 2, 2, 2, 2, 2, 2, 2, 2, 2, 2, 2, 2, 2, 3 ),
 ( 0.000000000000000000, 1.000000000000000000 ),
 ( 0.000000000000000000, 0.02000000000000000042, 0.04000000000000000083, 0.05999999999999999778, 0.08000000000000000167, 0.1000000000000000056, 0.1199999999999999956, 0.1400000000000000133, 0.1600000000000000033, 0.1799999999999999933, 0.2000000000000000111, 0.2200000000000000011, 0.2399999999999999911, 0.2600000000000000089, 0.2800000000000000266, 0.2999999999999999889, 0.3200000000000000067, 0.3400000000000000244, 0.3599999999999999867, 0.3800000000000000044, 0.4000000000000000222, 0.4199999999999999845, 0.4400000000000000022, 0.4600000000000000200, 0.4799999999999999822, 0.5000000000000000000, 0.5200000000000000178, 0.5400000000000000355, 0.5600000000000000533, 0.5799999999999999600, 0.5999999999999999778, 0.6199999999999999956, 0.6400000000000000133, 0.6600000000000000311, 0.6800000000000000488, 0.6999999999999999556, 0.7199999999999999734, 0.7399999999999999911, 0.7600000000000000089, 0.7800000000000000266, 0.8000000000000000444, 0.8199999999999999512, 0.8399999999999999689, 0.8599999999999999867, 0.8800000000000000044, 0.9000000000000000222, 0.9200000000000000400, 0.9399999999999999467, 0.9599999999999999645, 0.9799999999999999822, 1.000000000000000000 ),
 .UNSPECIFIED. ) 
 GEOMETRIC_REPRESENTATION_ITEM ( )  RATIONAL_B_SPLINE_SURFACE ( (
 ( 1.000000000000000000, 0.9510565162951535312, 1.000000000000000000, 0.9510565162951535312, 1.000000000000000000, 0.9510565162951535312, 1.000000000000000000, 0.9510565162951535312, 1.000000000000000000, 0.9510565162951535312, 1.000000000000000000, 0.9510565162951535312, 1.000000000000000000, 0.9510565162951535312, 1.000000000000000000, 0.9510565162951535312, 1.000000000000000000, 0.9510565162951535312, 1.000000000000000000, 0.9510565162951535312, 1.000000000000000000, 0.9510565162951535312, 1.000000000000000000, 0.9510565162951535312, 1.000000000000000000, 0.9510565162951535312, 1.000000000000000000, 0.9510565162951535312, 1.000000000000000000, 0.9510565162951535312, 1.000000000000000000, 0.9510565162951535312, 1.000000000000000000, 0.9510565162951535312, 1.000000000000000000, 0.9510565162951535312, 1.000000000000000000, 0.9510565162951535312, 1.000000000000000000, 0.9510565162951535312, 1.000000000000000000, 0.9510565162951535312, 1.000000000000000000, 0.9510565162951535312, 1.000000000000000000, 0.9510565162951535312, 1.000000000000000000, 0.9510565162951535312, 1.000000000000000000, 0.9510565162951535312, 1.000000000000000000, 0.9510565162951535312, 1.000000000000000000, 0.9510565162951535312, 1.000000000000000000, 0.9510565162951535312, 1.000000000000000000, 0.9510565162951535312, 1.000000000000000000, 0.9510565162951535312, 1.000000000000000000, 0.9510565162951535312, 1.000000000000000000, 0.9510565162951535312, 1.000000000000000000, 0.9510565162951535312, 1.000000000000000000, 0.9510565162951535312, 1.000000000000000000, 0.9510565162951535312, 1.000000000000000000, 0.9510565162951535312, 1.000000000000000000, 0.9510565162951535312, 1.000000000000000000, 0.9510565162951535312, 1.000000000000000000, 0.9510565162951535312, 1.000000000000000000, 0.9510565162951535312, 1.000000000000000000, 0.9510565162951535312, 1.000000000000000000, 0.9510565162951535312, 1.000000000000000000, 0.9510565162951535312, 1.000000000000000000, 0.9510565162951535312, 1.000000000000000000, 0.9510565162951535312, 1.000000000000000000, 0.9510565162951535312, 1.000000000000000000, 0.9510565162951535312, 1.000000000000000000, 0.9510565162951535312, 1.000000000000000000, 0.9510565162951535312, 1.000000000000000000, 0.9510565162951535312, 1.000000000000000000),
 ( 1.000000000000000000, 0.9510565162951535312, 1.000000000000000000, 0.9510565162951535312, 1.000000000000000000, 0.9510565162951535312, 1.000000000000000000, 0.9510565162951535312, 1.000000000000000000, 0.9510565162951535312, 1.000000000000000000, 0.9510565162951535312, 1.000000000000000000, 0.9510565162951535312, 1.000000000000000000, 0.9510565162951535312, 1.000000000000000000, 0.9510565162951535312, 1.000000000000000000, 0.9510565162951535312, 1.000000000000000000, 0.9510565162951535312, 1.000000000000000000, 0.9510565162951535312, 1.000000000000000000, 0.9510565162951535312, 1.000000000000000000, 0.9510565162951535312, 1.000000000000000000, 0.9510565162951535312, 1.000000000000000000, 0.9510565162951535312, 1.000000000000000000, 0.9510565162951535312, 1.000000000000000000, 0.9510565162951535312, 1.000000000000000000, 0.9510565162951535312, 1.000000000000000000, 0.9510565162951535312, 1.000000000000000000, 0.9510565162951535312, 1.000000000000000000, 0.9510565162951535312, 1.000000000000000000, 0.9510565162951535312, 1.000000000000000000, 0.9510565162951535312, 1.000000000000000000, 0.9510565162951535312, 1.000000000000000000, 0.9510565162951535312, 1.000000000000000000, 0.9510565162951535312, 1.000000000000000000, 0.9510565162951535312, 1.000000000000000000, 0.9510565162951535312, 1.000000000000000000, 0.9510565162951535312, 1.000000000000000000, 0.9510565162951535312, 1.000000000000000000, 0.9510565162951535312, 1.000000000000000000, 0.9510565162951535312, 1.000000000000000000, 0.9510565162951535312, 1.000000000000000000, 0.9510565162951535312, 1.000000000000000000, 0.9510565162951535312, 1.000000000000000000, 0.9510565162951535312, 1.000000000000000000, 0.9510565162951535312, 1.000000000000000000, 0.9510565162951535312, 1.000000000000000000, 0.9510565162951535312, 1.000000000000000000, 0.9510565162951535312, 1.000000000000000000, 0.9510565162951535312, 1.000000000000000000, 0.9510565162951535312, 1.000000000000000000, 0.9510565162951535312, 1.000000000000000000, 0.9510565162951535312, 1.000000000000000000, 0.9510565162951535312, 1.000000000000000000, 0.9510565162951535312, 1.000000000000000000, 0.9510565162951535312, 1.000000000000000000, 0.9510565162951535312, 1.000000000000000000, 0.9510565162951535312, 1.000000000000000000) ) ) 
 REPRESENTATION_ITEM ( '' )  SURFACE ( )  );
#181461=CARTESIAN_POINT ( 'NONE',  ( -6.020228577223754586E-15, 39.95556452105416412, -2.500000000000000444 ) ) ;
#181467=CARTESIAN_POINT ( 'NONE',  ( 31.79999999999936477, 1.011767027235951731E-12, 92.30000000000021032 ) ) ;
#181511=CARTESIAN_POINT ( 'NONE',  ( 34.37196153507746743, 7.030587757552861916, 47.62314794725693901 ) ) ;
#181576=CARTESIAN_POINT ( 'NONE',  ( -5.429308488886486681E-15, 30.30510711980690175, 147.7500000054623683 ) ) ;
#181629=CARTESIAN_POINT ( 'NONE',  ( 37.99626262588765258, 2.893932880411085066E-14, -1.002157773949823083 ) ) ;
#181705=CARTESIAN_POINT ( 'NONE',  ( 37.58407650405589351, 2.428612866815129610E-14, 39.49999999999996447 ) ) ;
#181775=LINE ( 'NONE', #101932, #115496 ) ;
#181788=EDGE_CURVE ( 'NONE', #26617, #108481, #157322, .T. ) ;
#181807=CARTESIAN_POINT ( 'NONE',  ( -22.44159573604010305, 16.30477369853692338, 145.1750000027311671 ) ) ;
#181831=CARTESIAN_POINT ( 'NONE',  ( -34.36935609104192224, 7.254501760396899535, 46.91913033384989262 ) ) ;
#181907=CARTESIAN_POINT ( 'NONE',  ( 23.48298174826590667, -32.32155151706770368, -3.302157773949822683 ) ) ;
#182006=AXIS2_PLACEMENT_3D ( 'NONE', #18158, #53448, #111139 ) ;
#182017=ORIENTED_EDGE ( 'NONE', *, *, #135020, .F. ) ;
#182048=CARTESIAN_POINT ( 'NONE',  ( -11.40812507854755609, 35.11059874428196537, -9.524999997268816188 ) ) ;
#182054=CARTESIAN_POINT ( 'NONE',  ( -29.87996255909766319, -22.90263037402382551, -8.000000000000003553 ) ) ;
#182093=CARTESIAN_POINT ( 'NONE',  ( -28.28060372831499336, 2.428612866367529932E-14, 148.5625000040967620 ) ) ;
#182122=CARTESIAN_POINT ( 'NONE',  ( 28.82186960331498327, 2.781578969918950771E-14, 139.2500000054623683 ) ) ;
#182155=VECTOR ( 'NONE', #74905, 1000.000000000000114 ) ;
#182159=ORIENTED_EDGE ( 'NONE', *, *, #43648, .T. ) ;
#182236=CARTESIAN_POINT ( 'NONE',  ( -36.91746825000000598, 2.428612866367529932E-14, -3.124999997268813168 ) ) ;
#182247=EDGE_LOOP ( 'NONE', ( #189215, #64449, #55097, #28582 ) ) ;
#182332=CARTESIAN_POINT ( 'NONE',  ( -27.73933785331498925, 2.428612866367529932E-14, 146.8750000027311842 ) ) ;
#182338=CARTESIAN_POINT ( 'NONE',  ( 22.44159573604009239, 16.30477369853692693, 142.0750000027311728 ) ) ;
#182342=DIRECTION ( 'NONE',  ( 1.000000000000000000, -0.000000000000000000, -0.000000000000000000 ) ) ;
#182431=DIRECTION ( 'NONE',  ( 1.000000000000000000, 0.000000000000000000, 0.000000000000000000 ) ) ;
#182445=CARTESIAN_POINT ( 'NONE',  ( 11.74264578624799427, 36.14014761921585972, -6.599999999999999645 ) ) ;
#182448=CARTESIAN_POINT ( 'NONE',  ( 37.99626262588765258, 2.893932880411085066E-14, -6.747842220587804363 ) ) ;
#182497=DIRECTION ( 'NONE',  ( -1.000000000000000000, 0.000000000000000000, -0.000000000000000000 ) ) ;
#182511=VECTOR ( 'NONE', #155004, 1000.000000000000000 ) ;
#182532=DIRECTION ( 'NONE',  ( 1.000000000000000000, 0.000000000000000000, 0.000000000000000000 ) ) ;
#182567=CARTESIAN_POINT ( 'NONE',  ( 28.82186960331477010, -9.364793116373819615, 139.1500000054623740 ) ) ;
#182771=CARTESIAN_POINT ( 'NONE',  ( -28.82186960331499037, 2.428612866367529932E-14, 144.0000000000000000 ) ) ;
#182774=VECTOR ( 'NONE', #157174, 1000.000000000000114 ) ;
#182799=CARTESIAN_POINT ( 'NONE',  ( -22.44159573604010305, 16.30477369853692338, 141.1750000027311671 ) ) ;
#182815=( BOUNDED_CURVE ( )  B_SPLINE_CURVE ( 2, ( #195312, #56793, #180157, #120430, #41626, #103290, #75917, #104282, #182122 ),
 .UNSPECIFIED., .F., .T. ) 
 B_SPLINE_CURVE_WITH_KNOTS ( ( 3, 2, 2, 2, 3 ),
 ( 0.8250928956683720727, 0.8400000000000000799, 0.8600000000000003197, 0.8800000000000005596, 0.9000000000000007994 ),
 .UNSPECIFIED. ) 
 CURVE ( )  GEOMETRIC_REPRESENTATION_ITEM ( )  RATIONAL_B_SPLINE_CURVE ( ( 0.9814209735438295112, 0.9635197191029262198, 1.000000000000000000, 0.9510565162951535312, 1.000000000000000000, 0.9510565162951535312, 1.000000000000000000, 0.9510565162951516438, 1.000000000000001998 ) ) 
 REPRESENTATION_ITEM ( '' )  );
#182824=CARTESIAN_POINT ( 'NONE',  ( -35.67631076299765169, 1.230297745838609957, 37.59750771353017740 ) ) ;
#183040=CARTESIAN_POINT ( 'NONE',  ( 22.81625015709509441, 31.40387420917330275, -1.324999997268813123 ) ) ;
#183046=CARTESIAN_POINT ( 'NONE',  ( 33.75669036400348944, 3.362847000060356972, 99.36731340788949751 ) ) ;
#183058=CARTESIAN_POINT ( 'NONE',  ( -22.81625015709510507, 31.40387420917330275, -5.424999997268812990 ) ) ;
#183086=CARTESIAN_POINT ( 'NONE',  ( 27.73933785331498925, -9.013057229001033122, 140.2750000027311330 ) ) ;
#183117=CARTESIAN_POINT ( 'NONE',  ( -40.00200000000003087, -1.163414459189985801E-14, 87.50000000000000000 ) ) ;
#183230=CARTESIAN_POINT ( 'NONE',  ( -11.40812507854754720, -35.11059874428192273, -8.724999997268813701 ) ) ;
#183281=CARTESIAN_POINT ( 'NONE',  ( -28.82186960331499037, 2.428612866367529932E-14, 142.0000000000000000 ) ) ;
#183313=CARTESIAN_POINT ( 'NONE',  ( -36.77885060843721021, 5.319724886534321406, 46.40826345025692490 ) ) ;
#183320=CARTESIAN_POINT ( 'NONE',  ( -8.571926809382601320, -26.38167802310801591, 143.2750000027311899 ) ) ;
#183325=CARTESIAN_POINT ( 'NONE',  ( 1.784210473542230573E-15, -29.16686587814331588, 145.3750000027311842 ) ) ;
#183473=VECTOR ( 'NONE', #185910, 1000.000000000000000 ) ;
#183486=CARTESIAN_POINT ( 'NONE',  ( 34.91303292417840964, 6.360705039060885468, 41.01876028008884845 ) ) ;
#183676=CARTESIAN_POINT ( 'NONE',  ( 36.91746824999999177, 2.880721459617395097E-14, -1.624999997268813390 ) ) ;
#183759=CARTESIAN_POINT ( 'NONE',  ( -36.84749596837620089, -2.912325675875796716, 49.66910675224617222 ) ) ;
#183788=CARTESIAN_POINT ( 'NONE',  ( -22.44159573604010305, 16.30477369853692338, 143.1750000027311671 ) ) ;
#183832=CARTESIAN_POINT ( 'NONE',  ( -11.74149087413294623, -36.13659316521243881, -7.347842220587803119 ) ) ;
#183915=DIRECTION ( 'NONE',  ( 1.000000000000000000, 0.000000000000000000, 0.000000000000000000 ) ) ;
#183917=CARTESIAN_POINT ( 'NONE',  ( -5.429308488886486681E-15, 30.30510711980690175, 141.7500000054623683 ) ) ;
#184020=FACE_OUTER_BOUND ( 'NONE', #62328, .T. ) ;
#184027=CARTESIAN_POINT ( 'NONE',  ( -36.91746825000000598, 2.428612866367529932E-14, -2.624999997268813168 ) ) ;
#184033=CARTESIAN_POINT ( 'NONE',  ( 33.98302989258738194, 4.936846515367096622, 92.54907045995906856 ) ) ;
#184067=CARTESIAN_POINT ( 'NONE',  ( -31.65994483839897100, -2.419126180341527821, 102.1034561864646122 ) ) ;
#184072=CARTESIAN_POINT ( 'NONE',  ( 8.571926809382597767, 26.38167802310806209, 140.7750000027311899 ) ) ;
#184156=DIRECTION ( 'NONE',  ( 1.000000000000000000, 0.000000000000000000, 0.000000000000000000 ) ) ;
#184217=CARTESIAN_POINT ( 'NONE',  ( 36.91746824999999177, 2.880721459617395097E-14, -4.124999997268813168 ) ) ;
#184303=CARTESIAN_POINT ( 'NONE',  ( -36.78370799935940738, 4.380135692641567324, 48.34576877258191274 ) ) ;
#184309=CARTESIAN_POINT ( 'NONE',  ( 1.784210473542230573E-15, -29.16686587814331588, 143.3750000027311557 ) ) ;
#184358=CARTESIAN_POINT ( 'NONE',  ( -3.573655867282028392E-15, 2.428612866367529932E-14, 139.9999999999999716 ) ) ;
#184383=CARTESIAN_POINT ( 'NONE',  ( 8.571926809382597767, 26.38167802310806209, 148.7750000027311899 ) ) ;
#184390=EDGE_CURVE ( 'NONE', #153137, #72946, #196036, .T. ) ;
#184473=CARTESIAN_POINT ( 'NONE',  ( 34.77165353390492442, 6.824181688848570460, 41.87898302971509423 ) ) ;
#184500=CARTESIAN_POINT ( 'NONE',  ( -3.573655867282028392E-15, 2.428612866367529932E-14, 0.000000000000000000 ) ) ;
#184629=ADVANCED_FACE ( 'NONE', ( #109868 ), #17879, .F. ) ;
#184655=VERTEX_POINT ( 'NONE', #46215 ) ;
#184660=CARTESIAN_POINT ( 'NONE',  ( -36.91746825000000598, 2.428612866367529932E-14, -0.6249999972688132788 ) ) ;
#184730=DIRECTION ( 'NONE',  ( 1.000000000000000000, 0.000000000000000000, 0.000000000000000000 ) ) ;
#184745=CARTESIAN_POINT ( 'NONE',  ( -37.43820758241025715, -2.754439498815796750, 40.23603015349058154 ) ) ;
#184765=DIRECTION ( 'NONE',  ( 1.000000000000000000, 0.000000000000000000, 3.709348145883536076E-20 ) ) ;
#184775=CARTESIAN_POINT ( 'NONE',  ( -22.44159573604009950, -16.30477369853688430, 143.5750000027311728 ) ) ;
#184798=CARTESIAN_POINT ( 'NONE',  ( -8.906447517083060816, 27.41122689804195645, 145.8500000054623627 ) ) ;
#184837=ORIENTED_EDGE ( 'NONE', *, *, #77338, .F. ) ;
#184890=CARTESIAN_POINT ( 'NONE',  ( 8.571926809382597767, 26.38167802310806209, 146.2750000027311899 ) ) ;
#184987=DIRECTION ( 'NONE',  ( 0.000000000000000000, 0.000000000000000000, 1.000000000000000000 ) ) ;
#185014=CARTESIAN_POINT ( 'NONE',  ( 3.556970738554033499E-15, -38.81732327939057825, -10.62499999726881050 ) ) ;
#185018=CARTESIAN_POINT ( 'NONE',  ( -37.99626262588765968, -12.34573411038913626, -3.647842220587803386 ) ) ;
#185033=CARTESIAN_POINT ( 'NONE',  ( -5.950531402560715689E-15, 38.81732327939063509, -5.624999997268813168 ) ) ;
#185117=CARTESIAN_POINT ( 'NONE',  ( -31.25082632804102190, 7.456723613865049671, 95.94516017006300501 ) ) ;
#185131=EDGE_LOOP ( 'NONE', ( #33592, #146822, #16667, #61157 ) ) ;
#185203=CARTESIAN_POINT ( 'NONE',  ( -29.86685920354755552, 21.69954338932564397, -9.324999997268813345 ) ) ;
#185289=DIRECTION ( 'NONE',  ( 1.000000000000000000, -0.000000000000000000, -0.000000000000000000 ) ) ;
#185293=AXIS2_PLACEMENT_3D ( 'NONE', #157159, #18654, #188501 ) ;
#185295=CARTESIAN_POINT ( 'NONE',  ( -27.73933785331498925, 2.428612866367529932E-14, 144.8750000027311842 ) ) ;
#185300=CARTESIAN_POINT ( 'NONE',  ( -22.44159573604010305, 16.30477369853692338, 140.6750000027311671 ) ) ;
#185369=CARTESIAN_POINT ( 'NONE',  ( -27.73933785331498925, 9.013057229001088189, 149.2750000027311614 ) ) ;
#185409=CARTESIAN_POINT ( 'NONE',  ( -11.74264578624800670, 36.14014761921585972, -8.400000000000000355 ) ) ;
#185427=CIRCLE ( 'NONE', #43410, 7.500000000000007105 ) ;
#185461=CARTESIAN_POINT ( 'NONE',  ( 35.63758492646879006, 1.954004632199990432, 37.74231687961066228 ) ) ;
#185652=CARTESIAN_POINT ( 'NONE',  ( -22.81625015709510507, 31.40387420917330275, -4.924999997268813878 ) ) ;
#185727=DIRECTION ( 'NONE',  ( 0.000000000000000000, 0.000000000000000000, -1.000000000000000000 ) ) ;
#185778=CARTESIAN_POINT ( 'NONE',  ( 27.73933785331498214, 9.013057229001095294, 142.4750000027311785 ) ) ;
#185801=CIRCLE ( 'NONE', #63101, 0.1999999999999987899 ) ;
#185803=CARTESIAN_POINT ( 'NONE',  ( -28.82186960331499392, -9.364793116373526516, 146.3500000054623627 ) ) ;
#185806=EDGE_CURVE ( 'NONE', #36039, #2296, #167008, .T. ) ;
#185896=CARTESIAN_POINT ( 'NONE',  ( -8.571926809382601320, -26.38167802310801591, 145.2750000027311899 ) ) ;
#185910=DIRECTION ( 'NONE',  ( 0.000000000000000000, 0.000000000000000000, 1.000000000000000000 ) ) ;
#186024=CARTESIAN_POINT ( 'NONE',  ( -36.91746825000001309, 11.99521256947798342, -2.724999997268813701 ) ) ;
#186029=CARTESIAN_POINT ( 'NONE',  ( 34.11680238834244250, 4.370175642590067078, 91.64155955192001102 ) ) ;
#186040=CARTESIAN_POINT ( 'NONE',  ( 36.91746824999999177, 2.880721459617395097E-14, -4.124999997268813168 ) ) ;
#186113=( BOUNDED_SURFACE ( )  B_SPLINE_SURFACE ( 1, 2, ( 
 ( #89029, #118385, #150720, #26387, #128774, #99443, #180079, #97428, #72889, #114609, #84266, #149714, #134557, #192470, #68109, #56713, #41548, #27383, #160126, #103211, #52935, #104205, #57714, #181067, #35781, #176307, #5432, #119384, #145947, #37779, #164893, #11213, #129761, #113606, #196245, #42542, #135552, #165886, #12219, #161123, #7428, #159114, #73882, #20608, #130778, #143952, #197224, #58686, #175300, #67116, #82260, #190473, #51946, #36766, #21614, #83272, #144946, #6427, #191457, #168835, #90022, #199195, #32333, #155666, #30340, #93986, #74861, #15172, #47506, #63662, #153675, #92987, #60663, #122336, #76831, #123321, #75836, #109162, #78815, #45509, #16168, #138503, #200184, #14168, #182048, #61653, #91981, #17162, #28384, #151705, #107164, #140494, #13198, #169842, #1982, #185014, #198204, #46500, #154673, #43531, #105196 ),
 ( #108160, #136523, #31336, #166883, #59675, #121347, #77822, #183040, #170842, #44523, #62649, #139491, #106179, #90992, #167862, #973, #124326, #29362, #152679, #137514, #184027, #186024, #66628, #94984, #128292, #114112, #189009, #156669, #19152, #3957, #141491, #36281, #98946, #160636, #158637, #65636, #189990, #110157, #126316, #172836, #145457, #21124, #50484, #33323, #82780, #187033, #20128, #159629, #2975, #51465, #144461, #5946, #112144, #49483, #18164, #34315, #48503, #113126, #127296, #22127, #175815, #64654, #80801, #142479, #171836, #79820, #37288, #81772, #143459, #67623, #173836, #35302, #97936, #129283, #4944, #157662, #174816, #190978, #83778, #188013, #52455, #96957, #6939, #125335, #111146, #95978, #8966, #38295, #149467, #55455, #70635, #25147, #194983, #162631, #146452, #71627, #9967, #165640, #56461, #72636, #132301 ) ),
 .UNSPECIFIED., .F., .F., .F. ) 
 B_SPLINE_SURFACE_WITH_KNOTS ( ( 2, 2 ),
 ( 3, 2, 2, 2, 2, 2, 2, 2, 2, 2, 2, 2, 2, 2, 2, 2, 2, 2, 2, 2, 2, 2, 2, 2, 2, 2, 2, 2, 2, 2, 2, 2, 2, 2, 2, 2, 2, 2, 2, 2, 2, 2, 2, 2, 2, 2, 2, 2, 2, 2, 3 ),
 ( 0.000000000000000000, 1.000000000000000000 ),
 ( 0.000000000000000000, 0.02000000000000000042, 0.04000000000000000083, 0.05999999999999999778, 0.08000000000000000167, 0.1000000000000000056, 0.1199999999999999956, 0.1400000000000000133, 0.1600000000000000033, 0.1799999999999999933, 0.2000000000000000111, 0.2200000000000000011, 0.2399999999999999911, 0.2600000000000000089, 0.2800000000000000266, 0.2999999999999999889, 0.3200000000000000067, 0.3400000000000000244, 0.3599999999999999867, 0.3800000000000000044, 0.4000000000000000222, 0.4199999999999999845, 0.4400000000000000022, 0.4600000000000000200, 0.4799999999999999822, 0.5000000000000000000, 0.5200000000000000178, 0.5400000000000000355, 0.5600000000000000533, 0.5799999999999999600, 0.5999999999999999778, 0.6199999999999999956, 0.6400000000000000133, 0.6600000000000000311, 0.6800000000000000488, 0.6999999999999999556, 0.7199999999999999734, 0.7399999999999999911, 0.7600000000000000089, 0.7800000000000000266, 0.8000000000000000444, 0.8199999999999999512, 0.8399999999999999689, 0.8599999999999999867, 0.8800000000000000044, 0.9000000000000000222, 0.9200000000000000400, 0.9399999999999999467, 0.9599999999999999645, 0.9799999999999999822, 1.000000000000000000 ),
 .UNSPECIFIED. ) 
 GEOMETRIC_REPRESENTATION_ITEM ( )  RATIONAL_B_SPLINE_SURFACE ( (
 ( 1.000000000000000000, 0.9510565162951535312, 1.000000000000000000, 0.9510565162951535312, 1.000000000000000000, 0.9510565162951535312, 1.000000000000000000, 0.9510565162951535312, 1.000000000000000000, 0.9510565162951535312, 1.000000000000000000, 0.9510565162951535312, 1.000000000000000000, 0.9510565162951535312, 1.000000000000000000, 0.9510565162951535312, 1.000000000000000000, 0.9510565162951535312, 1.000000000000000000, 0.9510565162951535312, 1.000000000000000000, 0.9510565162951535312, 1.000000000000000000, 0.9510565162951535312, 1.000000000000000000, 0.9510565162951535312, 1.000000000000000000, 0.9510565162951535312, 1.000000000000000000, 0.9510565162951535312, 1.000000000000000000, 0.9510565162951535312, 1.000000000000000000, 0.9510565162951535312, 1.000000000000000000, 0.9510565162951535312, 1.000000000000000000, 0.9510565162951535312, 1.000000000000000000, 0.9510565162951535312, 1.000000000000000000, 0.9510565162951535312, 1.000000000000000000, 0.9510565162951535312, 1.000000000000000000, 0.9510565162951535312, 1.000000000000000000, 0.9510565162951535312, 1.000000000000000000, 0.9510565162951535312, 1.000000000000000000, 0.9510565162951535312, 1.000000000000000000, 0.9510565162951535312, 1.000000000000000000, 0.9510565162951535312, 1.000000000000000000, 0.9510565162951535312, 1.000000000000000000, 0.9510565162951535312, 1.000000000000000000, 0.9510565162951535312, 1.000000000000000000, 0.9510565162951535312, 1.000000000000000000, 0.9510565162951535312, 1.000000000000000000, 0.9510565162951535312, 1.000000000000000000, 0.9510565162951535312, 1.000000000000000000, 0.9510565162951535312, 1.000000000000000000, 0.9510565162951535312, 1.000000000000000000, 0.9510565162951535312, 1.000000000000000000, 0.9510565162951535312, 1.000000000000000000, 0.9510565162951535312, 1.000000000000000000, 0.9510565162951535312, 1.000000000000000000, 0.9510565162951535312, 1.000000000000000000, 0.9510565162951535312, 1.000000000000000000, 0.9510565162951535312, 1.000000000000000000, 0.9510565162951535312, 1.000000000000000000, 0.9510565162951535312, 1.000000000000000000, 0.9510565162951535312, 1.000000000000000000, 0.9510565162951535312, 1.000000000000000000, 0.9510565162951535312, 1.000000000000000000, 0.9510565162951535312, 1.000000000000000000),
 ( 1.000000000000000000, 0.9510565162951535312, 1.000000000000000000, 0.9510565162951535312, 1.000000000000000000, 0.9510565162951535312, 1.000000000000000000, 0.9510565162951535312, 1.000000000000000000, 0.9510565162951535312, 1.000000000000000000, 0.9510565162951535312, 1.000000000000000000, 0.9510565162951535312, 1.000000000000000000, 0.9510565162951535312, 1.000000000000000000, 0.9510565162951535312, 1.000000000000000000, 0.9510565162951535312, 1.000000000000000000, 0.9510565162951535312, 1.000000000000000000, 0.9510565162951535312, 1.000000000000000000, 0.9510565162951535312, 1.000000000000000000, 0.9510565162951535312, 1.000000000000000000, 0.9510565162951535312, 1.000000000000000000, 0.9510565162951535312, 1.000000000000000000, 0.9510565162951535312, 1.000000000000000000, 0.9510565162951535312, 1.000000000000000000, 0.9510565162951535312, 1.000000000000000000, 0.9510565162951535312, 1.000000000000000000, 0.9510565162951535312, 1.000000000000000000, 0.9510565162951535312, 1.000000000000000000, 0.9510565162951535312, 1.000000000000000000, 0.9510565162951535312, 1.000000000000000000, 0.9510565162951535312, 1.000000000000000000, 0.9510565162951535312, 1.000000000000000000, 0.9510565162951535312, 1.000000000000000000, 0.9510565162951535312, 1.000000000000000000, 0.9510565162951535312, 1.000000000000000000, 0.9510565162951535312, 1.000000000000000000, 0.9510565162951535312, 1.000000000000000000, 0.9510565162951535312, 1.000000000000000000, 0.9510565162951535312, 1.000000000000000000, 0.9510565162951535312, 1.000000000000000000, 0.9510565162951535312, 1.000000000000000000, 0.9510565162951535312, 1.000000000000000000, 0.9510565162951535312, 1.000000000000000000, 0.9510565162951535312, 1.000000000000000000, 0.9510565162951535312, 1.000000000000000000, 0.9510565162951535312, 1.000000000000000000, 0.9510565162951535312, 1.000000000000000000, 0.9510565162951535312, 1.000000000000000000, 0.9510565162951535312, 1.000000000000000000, 0.9510565162951535312, 1.000000000000000000, 0.9510565162951535312, 1.000000000000000000, 0.9510565162951535312, 1.000000000000000000, 0.9510565162951535312, 1.000000000000000000, 0.9510565162951535312, 1.000000000000000000, 0.9510565162951535312, 1.000000000000000000, 0.9510565162951535312, 1.000000000000000000) ) ) 
 REPRESENTATION_ITEM ( '' )  SURFACE ( )  );
#186217=CARTESIAN_POINT ( 'NONE',  ( -22.81625015709510507, 31.40387420917330275, -7.424999997268812990 ) ) ;
#186268=CARTESIAN_POINT ( 'NONE',  ( 8.906447517083050158, 27.41122689804195645, 143.4000000000000057 ) ) ;
#186305=CARTESIAN_POINT ( 'NONE',  ( 27.73933785331498214, 9.013057229001095294, 141.9750000027311501 ) ) ;
#186365=EDGE_CURVE ( 'NONE', #184655, #36039, #144936, .T. ) ;
#186403=CARTESIAN_POINT ( 'NONE',  ( 23.31738231874054890, -16.94106989632523508, 145.0500000054623513 ) ) ;
#186418=VERTEX_POINT ( 'NONE', #128764 ) ;
#186423=CARTESIAN_POINT ( 'NONE',  ( -38.00000000000001421, -12.34694845685042708, -9.899999999999998579 ) ) ;
#186432=FACE_OUTER_BOUND ( 'NONE', #29005, .T. ) ;
#186529=CIRCLE ( 'NONE', #102523, 37.99626262588765968 ) ;
#186535=ORIENTED_EDGE ( 'NONE', *, *, #47794, .F. ) ;
#186595=DIRECTION ( 'NONE',  ( -1.000000000000000000, 0.000000000000000000, 0.000000000000000000 ) ) ;
#186630=CARTESIAN_POINT ( 'NONE',  ( -28.82186960331499037, 2.428612866367529932E-14, 146.0000000000000000 ) ) ;
#186635=CARTESIAN_POINT ( 'NONE',  ( 33.72427247603957312, -5.492275790717719985, 95.34298344322786534 ) ) ;
#186703=ADVANCED_FACE ( 'NONE', ( #112610 ), #97417, .T. ) ;
#186714=ORIENTED_EDGE ( 'NONE', *, *, #69759, .T. ) ;
#186743=DIRECTION ( 'NONE',  ( 1.000000000000000000, 0.000000000000000000, 0.000000000000000000 ) ) ;
#186759=CARTESIAN_POINT ( 'NONE',  ( -28.28060372831499336, 2.428612866367529932E-14, 138.5625000040967620 ) ) ;
#186790=CARTESIAN_POINT ( 'NONE',  ( -23.31738231874055245, -16.94106989632524574, 146.1999999999999886 ) ) ;
#186815=CARTESIAN_POINT ( 'NONE',  ( 17.81289503416610742, 24.51734667627700404, 147.5500000054623229 ) ) ;
#186903=EDGE_LOOP ( 'NONE', ( #188038, #134060, #97262, #43557 ) ) ;
#186906=CARTESIAN_POINT ( 'NONE',  ( 8.571926809382597767, 26.38167802310806209, 144.2750000027311899 ) ) ;
#186951=( BOUNDED_CURVE ( )  B_SPLINE_CURVE ( 2, ( #87556, #149243, #197732, #103734, #147237, #88550, #59198, #8729, #118912, #26907, #44050 ),
 .UNSPECIFIED., .F., .T. ) 
 B_SPLINE_CURVE_WITH_KNOTS ( ( 3, 2, 2, 2, 2, 3 ),
 ( 0.4000000000000003553, 0.4200000000000003175, 0.4400000000000003908, 0.4600000000000004086, 0.4800000000000004263, 0.5000000000000004441 ),
 .UNSPECIFIED. ) 
 CURVE ( )  GEOMETRIC_REPRESENTATION_ITEM ( )  RATIONAL_B_SPLINE_CURVE ( ( 0.9999999999999992228, 0.9510565162951543083, 1.000000000000000000, 0.9510565162951535312, 1.000000000000000000, 0.9510565162951535312, 1.000000000000000000, 0.9510565162951535312, 1.000000000000000000, 0.9510565162951524210, 1.000000000000001110 ) ) 
 REPRESENTATION_ITEM ( '' )  );
#187021=ORIENTED_EDGE ( 'NONE', *, *, #59945, .T. ) ;
#187033=CARTESIAN_POINT ( 'NONE',  ( -5.950531402560715689E-15, 38.81732327939063509, -5.124999997268813168 ) ) ;
#187036=CARTESIAN_POINT ( 'NONE',  ( 3.765340386950246872E-15, -39.95163481335715971, -3.247842220587803030 ) ) ;
#187050=CARTESIAN_POINT ( 'NONE',  ( -29.86685920354755552, 21.69954338932564397, -7.324999997268814234 ) ) ;
#187084=DIRECTION ( 'NONE',  ( 1.000000000000000000, 0.000000000000000000, 3.709348145883536076E-20 ) ) ;
#187091=ORIENTED_EDGE ( 'NONE', *, *, #184390, .T. ) ;
#187219=CARTESIAN_POINT ( 'NONE',  ( 29.86685920354754842, -21.69954338932559068, -8.324999997268813345 ) ) ;
#187246=CARTESIAN_POINT ( 'NONE',  ( -3.573655867282028392E-15, 2.428612866367529932E-14, 2.000000000000000000 ) ) ;
#187248=EDGE_CURVE ( 'NONE', #83417, #189747, #47195, .T. ) ;
#187277=DIRECTION ( 'NONE',  ( -1.000000000000000000, 0.000000000000000000, -6.982962677686266711E-15 ) ) ;
#187300=CARTESIAN_POINT ( 'NONE',  ( 38.00373040315627549, 2.428612866367529932E-14, -0.1220970790697140096 ) ) ;
#187306=CARTESIAN_POINT ( 'NONE',  ( 8.571926809382597767, 26.38167802310806209, 140.2750000027311899 ) ) ;
#187311=CARTESIAN_POINT ( 'NONE',  ( -22.44159573604009950, -16.30477369853688430, 139.0750000027311728 ) ) ;
#187379=CARTESIAN_POINT ( 'NONE',  ( -5.359611314223446995E-15, 29.16686587814335851, 142.8750000027311842 ) ) ;
#187420=CARTESIAN_POINT ( 'NONE',  ( -11.74264578624799782, -36.14014761921581709, -7.599999999999999645 ) ) ;
#187433=PRODUCT_DEFINITION_SHAPE ( 'NONE', 'NONE',  #117858 ) ;
#187543=CARTESIAN_POINT ( 'NONE',  ( -36.91746825000000598, 2.428612866367529932E-14, -0.6249999972688132788 ) ) ;
#187627=CARTESIAN_POINT ( 'NONE',  ( 34.48725679702496905, -1.430676605895442766, 89.67714645826993092 ) ) ;
#187660=CARTESIAN_POINT ( 'NONE',  ( 11.40812507854754365, 35.11059874428196537, -1.224999997268813479 ) ) ;
#187668=CARTESIAN_POINT ( 'NONE',  ( -37.99626262588766679, 2.428612866367529932E-14, -4.002157773949823749 ) ) ;
#187750=CARTESIAN_POINT ( 'NONE',  ( 32.64453336272026718, -0.4913453444576664220, 87.50000000000002842 ) ) ;
#187753=DIRECTION ( 'NONE',  ( 0.000000000000000000, 0.000000000000000000, -1.000000000000000000 ) ) ;
#187778=CARTESIAN_POINT ( 'NONE',  ( -27.73933785331498925, -9.013057229001049109, 139.4750000027311785 ) ) ;
#187802=CARTESIAN_POINT ( 'NONE',  ( 23.31738231874054534, 16.94106989632529192, 139.4500000054623570 ) ) ;
#187889=ORIENTED_EDGE ( 'NONE', *, *, #39120, .T. ) ;
#187892=CARTESIAN_POINT ( 'NONE',  ( -27.73933785331498925, -9.013057229001049109, 146.9750000027311785 ) ) ;
#187938=VERTEX_POINT ( 'NONE', #79810 ) ;
#188013=CARTESIAN_POINT ( 'NONE',  ( -36.91746825000001309, -11.99521256947794789, -8.524999997268812635 ) ) ;
#188014=CARTESIAN_POINT ( 'NONE',  ( -33.76801240946108607, 5.498839508946046450, 94.61983786177950151 ) ) ;
#188038=ORIENTED_EDGE ( 'NONE', *, *, #49302, .F. ) ;
#188066=CARTESIAN_POINT ( 'NONE',  ( 35.50125023021172410, -3.320518091344034417, 38.27062242752713672 ) ) ;
#188095=CARTESIAN_POINT ( 'NONE',  ( 31.99364916731008179, -5.510910596142776387E-15, 42.35000000000022169 ) ) ;
#188202=CARTESIAN_POINT ( 'NONE',  ( 3.556970738554033499E-15, -38.81732327939057825, -10.62499999726881050 ) ) ;
#188288=CARTESIAN_POINT ( 'NONE',  ( -8.571926809382601320, -26.38167802310801591, 141.2750000027311899 ) ) ;
#188292=CARTESIAN_POINT ( 'NONE',  ( -17.14385361876520264, -23.59649016807271593, 139.1750000027311955 ) ) ;
#188321=VERTEX_POINT ( 'NONE', #86778 ) ;
#188345=ADVANCED_FACE ( 'NONE', ( #149457 ), #161626, .T. ) ;
#188359=CARTESIAN_POINT ( 'NONE',  ( 22.44159573604009594, -16.30477369853687364, 148.1750000027311671 ) ) ;
#188490=CARTESIAN_POINT ( 'NONE',  ( -35.52771690032648166, -3.099362195827484179, 38.16599597228981366 ) ) ;
#188501=DIRECTION ( 'NONE',  ( 0.000000000000000000, 0.000000000000000000, -1.000000000000000000 ) ) ;
#188523=CARTESIAN_POINT ( 'NONE',  ( -29.86685920354755197, -21.69954338932560134, -2.424999997268813434 ) ) ;
#188611=CARTESIAN_POINT ( 'NONE',  ( 33.86249154851669374, -5.319940558880595916, 93.55791698674948975 ) ) ;
#188646=CARTESIAN_POINT ( 'NONE',  ( 3.556970738554033499E-15, -38.81732327939057825, -10.12499999726881228 ) ) ;
#188719=DIRECTION ( 'NONE',  ( 1.000000000000000000, -0.000000000000000000, -0.000000000000000000 ) ) ;
#188760=AXIS2_PLACEMENT_3D ( 'NONE', #52706, #144713, #143718 ) ;
#188766=CARTESIAN_POINT ( 'NONE',  ( 27.73933785331498569, 2.768321779492822058E-14, 140.3750000027311842 ) ) ;
#188788=CARTESIAN_POINT ( 'NONE',  ( -23.31738231874055245, -16.94106989632524574, 140.1999999999999886 ) ) ;
#188789=CARTESIAN_POINT ( 'NONE',  ( 17.81289503416611453, -24.51734667627695785, 142.9500000054623854 ) ) ;
#188792=VECTOR ( 'NONE', #145509, 1000.000000000000000 ) ;
#188880=ORIENTED_EDGE ( 'NONE', *, *, #154932, .F. ) ;
#188883=CARTESIAN_POINT ( 'NONE',  ( -8.571926809382608425, 26.38167802310805854, 142.4750000027312069 ) ) ;
#188941=VECTOR ( 'NONE', #58450, 1000.000000000000000 ) ;
#189009=CARTESIAN_POINT ( 'NONE',  ( 11.40812507854754365, 35.11059874428196537, -3.224999997268813701 ) ) ;
#189055=VERTEX_POINT ( 'NONE', #166630 ) ;
#189067=CARTESIAN_POINT ( 'NONE',  ( 34.77074502975525405, -6.826893893699448768, 41.88499232265944272 ) ) ;
#189215=ORIENTED_EDGE ( 'NONE', *, *, #199664, .F. ) ;
#189250=DIRECTION ( 'NONE',  ( 0.000000000000000000, 0.000000000000000000, 1.000000000000000000 ) ) ;
#189251=CARTESIAN_POINT ( 'NONE',  ( 2.366582413085430048, -37.03054742343285710, -7.999999999999996447 ) ) ;
#189269=ORIENTED_EDGE ( 'NONE', *, *, #157283, .F. ) ;
#189286=CARTESIAN_POINT ( 'NONE',  ( 22.44159573604009239, 16.30477369853692693, 140.0750000027311728 ) ) ;
#189298=EDGE_LOOP ( 'NONE', ( #140803, #129720 ) ) ;
#189357=CARTESIAN_POINT ( 'NONE',  ( -27.73933785331498925, -9.013057229001049109, 147.4750000027311785 ) ) ;
#189434=CARTESIAN_POINT ( 'NONE',  ( -6.020228577223754586E-15, 39.95556452105416412, -4.249999994537627224 ) ) ;
#189447=CARTESIAN_POINT ( 'NONE',  ( -37.99533089065118219, -0.2660902954431525469, -7.999999999999996447 ) ) ;
#189473=CARTESIAN_POINT ( 'NONE',  ( 40.00000000000001421, 2.428612866367529932E-14, 0.000000000000000000 ) ) ;
#189518=CARTESIAN_POINT ( 'NONE',  ( -5.950531402560715689E-15, 38.81732327939063509, -7.124999997268814056 ) ) ;
#189636=CARTESIAN_POINT ( 'NONE',  ( -6.020228577223754586E-15, 39.95556452105416412, -0.4999999999999999445 ) ) ;
#189728=CARTESIAN_POINT ( 'NONE',  ( 31.37893600750392409, -5.659358439387617068, 99.94586368981259739 ) ) ;
#189746=EDGE_CURVE ( 'NONE', #59237, #126834, #123079, .T. ) ;
#189747=VERTEX_POINT ( 'NONE', #75586 ) ;
#189759=CARTESIAN_POINT ( 'NONE',  ( -8.571926809382601320, -26.38167802310801591, 139.7750000027311899 ) ) ;
#189772=ADVANCED_FACE ( 'NONE', ( #90749, #195987 ), #153427, .T. ) ;
#189781=CARTESIAN_POINT ( 'NONE',  ( -28.82186960331499392, -9.364793116373526516, 142.3500000054623342 ) ) ;
#189844=CARTESIAN_POINT ( 'NONE',  ( 11.74149087413294268, 36.13659316521247433, -2.347842220587804452 ) ) ;
#189886=CARTESIAN_POINT ( 'NONE',  ( -17.81289503416611097, -24.51734667627696496, 148.2999999999999545 ) ) ;
#189890=CARTESIAN_POINT ( 'NONE',  ( 36.77739090780051612, -5.326908766905467552, 46.41547615974452867 ) ) ;
#189917=ORIENTED_EDGE ( 'NONE', *, *, #150856, .T. ) ;
#189990=CARTESIAN_POINT ( 'NONE',  ( -11.40812507854754720, -35.11059874428192273, -4.224999997268813701 ) ) ;
#190020=ORIENTED_EDGE ( 'NONE', *, *, #127529, .T. ) ;
#190063=DIRECTION ( 'NONE',  ( 0.000000000000000000, -1.000000000000000000, 0.000000000000000000 ) ) ;
#190182=CARTESIAN_POINT ( 'NONE',  ( -36.91746825000000598, 2.428612866367529932E-14, -11.12499999726881228 ) ) ;
#190230=LINE ( 'NONE', #192231, #172483 ) ;
#190269=CARTESIAN_POINT ( 'NONE',  ( 17.14385361876520264, 23.59649016807275856, 142.1750000027311671 ) ) ;
#190341=CARTESIAN_POINT ( 'NONE',  ( -5.359611314223446995E-15, 29.16686587814335851, 146.8750000027311557 ) ) ;
#190420=CARTESIAN_POINT ( 'NONE',  ( 3.766062262543149401E-15, -39.95556452105413570, -5.249999994537625447 ) ) ;
#190463=CARTESIAN_POINT ( 'NONE',  ( -3.573655867282028392E-15, 2.428612866367529932E-14, 139.9999999999999716 ) ) ;
#190471=CARTESIAN_POINT ( 'NONE',  ( 37.58407650405589351, 2.428612866815129610E-14, 39.49999999999996447 ) ) ;
#190473=CARTESIAN_POINT ( 'NONE',  ( 36.91746825000000598, -11.99521256947793546, -6.224999997268814589 ) ) ;
#190505=CARTESIAN_POINT ( 'NONE',  ( -11.40812507854755609, 35.11059874428196537, -3.024999997268813523 ) ) ;
#190625=CARTESIAN_POINT ( 'NONE',  ( 36.91746825000000598, -11.99521256947793546, -9.724999997268813701 ) ) ;
#190716=CARTESIAN_POINT ( 'NONE',  ( 31.48242569098776755, -7.251655820954947096, 93.02470426148725835 ) ) ;
#190745=CARTESIAN_POINT ( 'NONE',  ( -5.429308488886486681E-15, 30.30510711980690175, 149.5000000000000000 ) ) ;
#190766=CARTESIAN_POINT ( 'NONE',  ( 28.82186960331498327, 9.364793116373570925, 139.3500000054623911 ) ) ;
#190781=EDGE_CURVE ( 'NONE', #49688, #4689, #116880, .T. ) ;
#190809=EDGE_LOOP ( 'NONE', ( #139690, #154931, #99937, #76397 ) ) ;
#190875=FACE_OUTER_BOUND ( 'NONE', #51934, .T. ) ;
#190877=CARTESIAN_POINT ( 'NONE',  ( 36.76911729423384401, -4.939512937650262003, 47.42567687524350362 ) ) ;
#190978=CARTESIAN_POINT ( 'NONE',  ( -22.81625015709509441, -31.40387420917324590, -8.324999997268815122 ) ) ;
#191035=CARTESIAN_POINT ( 'NONE',  ( 35.70266437024449147, 2.428612576286966776E-14, 37.50000000000000000 ) ) ;
#191100=ADVANCED_FACE ( 'NONE', ( #110551, #186432 ), #66036, .T. ) ;
#191142=DIRECTION ( 'NONE',  ( 0.000000000000000000, 0.000000000000000000, -1.000000000000000000 ) ) ;
#191228=DIRECTION ( 'NONE',  ( -1.000000000000000000, 0.000000000000000000, 0.000000000000000000 ) ) ;
#191262=CARTESIAN_POINT ( 'NONE',  ( -27.73933785331498925, -9.013057229001049109, 145.4750000027311501 ) ) ;
#191272=ORIENTED_EDGE ( 'NONE', *, *, #130121, .F. ) ;
#191331=CARTESIAN_POINT ( 'NONE',  ( -27.73933785331498925, -9.013057229001049109, 143.4750000027312069 ) ) ;
#191409=CARTESIAN_POINT ( 'NONE',  ( 30.74264578624800137, -22.33583958711395212, -6.949999994537627401 ) ) ;
#191417=VERTEX_POINT ( 'NONE', #67034 ) ;
#191443=CARTESIAN_POINT ( 'NONE',  ( 31.64616484836359334, 2.655180720736611377, 102.0186121717492682 ) ) ;
#191456=CARTESIAN_POINT ( 'NONE',  ( 37.54602941011386719, 1.427078192699139159, 39.68530545529165465 ) ) ;
#191457=CARTESIAN_POINT ( 'NONE',  ( -29.86685920354755197, -21.69954338932560134, -6.924999997268813878 ) ) ;
#191459=CARTESIAN_POINT ( 'NONE',  ( -35.70266437024450568, -5.510913496957479854E-15, 37.50000000000000000 ) ) ;
#191488=CARTESIAN_POINT ( 'NONE',  ( 36.91746824999999887, -11.99521256947793546, -1.724999997268813479 ) ) ;
#191612=CARTESIAN_POINT ( 'NONE',  ( -36.91746825000000598, 2.428612866367529932E-14, -10.62499999726881406 ) ) ;
#191697=DIRECTION ( 'NONE',  ( 0.000000000000000000, 0.000000000000000000, -1.000000000000000000 ) ) ;
#191732=CARTESIAN_POINT ( 'NONE',  ( 23.31738231874054890, -16.94106989632523508, 144.7999999999999829 ) ) ;
#191756=CARTESIAN_POINT ( 'NONE',  ( 28.82186960331498327, 9.364793116373570925, 141.3500000054623627 ) ) ;
#191948=DIRECTION ( 'NONE',  ( 0.000000000000000000, 0.000000000000000000, -1.000000000000000000 ) ) ;
#191969=CARTESIAN_POINT ( 'NONE',  ( 27.73933785331498925, -9.013057229001033122, 148.2750000027311330 ) ) ;
#192049=DIRECTION ( 'NONE',  ( 1.000000000000000000, 0.000000000000000000, 0.000000000000000000 ) ) ;
#192053=DIRECTION ( 'NONE',  ( -0.000000000000000000, -0.000000000000000000, -1.000000000000000000 ) ) ;
#192072=FACE_OUTER_BOUND ( 'NONE', #160937, .T. ) ;
#192182=CARTESIAN_POINT ( 'NONE',  ( 36.91631499011236883, -2.427738359554614700, -8.000000000000001776 ) ) ;
#192231=CARTESIAN_POINT ( 'NONE',  ( 28.82186960331498327, 2.428612866367529932E-14, 139.9999999999999716 ) ) ;
#192266=CARTESIAN_POINT ( 'NONE',  ( -31.68593437162162729, -6.718755962661541403, 91.65819149638744534 ) ) ;
#192270=CARTESIAN_POINT ( 'NONE',  ( -8.571926809382601320, -26.38167802310801591, 141.7750000027311899 ) ) ;
#192344=CARTESIAN_POINT ( 'NONE',  ( 27.73933785331498925, -9.013057229001034898, 140.2750000027311614 ) ) ;
#192387=DIRECTION ( 'NONE',  ( 1.000000000000000000, 0.000000000000000000, 0.000000000000000000 ) ) ;
#192421=CARTESIAN_POINT ( 'NONE',  ( 11.74264578624799427, 36.14014761921585972, -2.349999994537626868 ) ) ;
#192468=CARTESIAN_POINT ( 'NONE',  ( 37.58407650405589351, 0.3600258186295152152, 39.49999999999997868 ) ) ;
#192470=CARTESIAN_POINT ( 'NONE',  ( 22.81625015709510151, -31.40387420917324590, -2.424999997268812546 ) ) ;
#192501=CARTESIAN_POINT ( 'NONE',  ( -37.58407650405589351, 1.968340676919130544E-14, 39.49999999999996447 ) ) ;
#192515=EDGE_CURVE ( 'NONE', #44815, #68886, #172159, .T. ) ;
#192517=LINE ( 'NONE', #97473, #173619 ) ;
#192553=DIRECTION ( 'NONE',  ( -1.000000000000000000, 0.000000000000000000, 0.000000000000000000 ) ) ;
#192574=VECTOR ( 'NONE', #21921, 1000.000000000000000 ) ;
#192624=CARTESIAN_POINT ( 'NONE',  ( 36.91746824999999177, 2.880721459617395097E-14, -9.624999997268814056 ) ) ;
#192787=B_SPLINE_CURVE_WITH_KNOTS ( 'NONE', 3,
 ( #83983, #145662, #116331, #7143, #23333, #68826, #130485, #192182, #53663, #115341, #38501, #101148, #177031, #193184, #84977, #146659, #8153, #178020, #162834, #85993, #200142, #27343, #198163, #45468 ),
 .UNSPECIFIED., .F., .F.,
 ( 4, 2, 2, 2, 2, 2, 2, 2, 2, 2, 2, 4 ),
 ( 0.000000000000000000, 0.007239606870481569631, 0.01085941030572235705, 0.01447921374096314273, 0.02171882061144471757, 0.02895842748192629240, 0.03257823091716707808, 0.03619803435240785683, 0.03981783778764864251, 0.04343764122288943513, 0.05067724809337099262, 0.05791685496385254317 ),
 .UNSPECIFIED. ) ;
#192893=ADVANCED_FACE ( 'NONE', ( #184020 ), #10829, .F. ) ;
#192983=CARTESIAN_POINT ( 'NONE',  ( 22.44159573604009239, 16.30477369853692693, 148.5750000027312012 ) ) ;
#192992=ORIENTED_EDGE ( 'NONE', *, *, #93145, .F. ) ;
#193006=CARTESIAN_POINT ( 'NONE',  ( -34.45218533337747147, 5.971079431359530787, 49.56529461667049219 ) ) ;
#193177=CARTESIAN_POINT ( 'NONE',  ( 3.765340386950246872E-15, -39.95163481335715971, -5.502157773949822861 ) ) ;
#193184=CARTESIAN_POINT ( 'NONE',  ( 31.99765134899338648, -18.45278125975086070, -7.999999999999998224 ) ) ;
#193233=CARTESIAN_POINT ( 'NONE',  ( -34.02657648861389106, -4.769071838117368678, 92.23683055719308754 ) ) ;
#193272=CARTESIAN_POINT ( 'NONE',  ( 22.44159573604009594, -16.30477369853687364, 144.1750000027311671 ) ) ;
#193284=EDGE_LOOP ( 'NONE', ( #32152, #18454, #168149, #199313 ) ) ;
#193304=DIRECTION ( 'NONE',  ( -1.000000000000000000, 0.000000000000000000, -6.982962677686266711E-15 ) ) ;
#193344=DIRECTION ( 'NONE',  ( 1.000000000000000000, 0.000000000000000000, 0.000000000000000000 ) ) ;
#193346=CARTESIAN_POINT ( 'NONE',  ( 27.73933785331498569, 2.768321779492822058E-14, 147.8750000027311842 ) ) ;
#193422=CARTESIAN_POINT ( 'NONE',  ( 38.00000000000000711, -12.34694845685040754, -2.849999994537626424 ) ) ;
#193551=EDGE_CURVE ( 'NONE', #122026, #199732, #156136, .T. ) ;
#193587=DIRECTION ( 'NONE',  ( 0.000000000000000000, 0.000000000000000000, 1.000000000000000000 ) ) ;
#193592=CARTESIAN_POINT ( 'NONE',  ( -31.99364916731038022, -5.510910596163089556E-15, 45.00000000000000000 ) ) ;
#193619=VERTEX_POINT ( 'NONE', #129276 ) ;
#193625=ORIENTED_EDGE ( 'NONE', *, *, #156164, .F. ) ;
#193630=CARTESIAN_POINT ( 'NONE',  ( -30.74264578624800492, 22.33583958711400186, -6.200000000000001066 ) ) ;
#193659=AXIS2_PLACEMENT_3D ( 'NONE', #105313, #74000, #42663 ) ;
#193718=DIRECTION ( 'NONE',  ( -1.000000000000000000, -0.000000000000000000, -0.000000000000000000 ) ) ;
#193753=CARTESIAN_POINT ( 'NONE',  ( -23.31738231874055600, 16.94106989632528837, 148.0500000054623797 ) ) ;
#193755=CARTESIAN_POINT ( 'NONE',  ( -8.906447517083053711, -27.41122689804191026, 138.6500000054623740 ) ) ;
#193801=( BOUNDED_CURVE ( )  B_SPLINE_CURVE ( 2, ( #168728, #156562, #47400, #80697, #868, #200080, #142374, #62543, #91874, #61548, #3854 ),
 .UNSPECIFIED., .F., .F. ) 
 B_SPLINE_CURVE_WITH_KNOTS ( ( 3, 2, 2, 2, 2, 3 ),
 ( 0.3000000000000000999, 0.3200000000000000067, 0.3400000000000000799, 0.3600000000000000977, 0.3800000000000001155, 0.4000000000000001332 ),
 .UNSPECIFIED. ) 
 CURVE ( )  GEOMETRIC_REPRESENTATION_ITEM ( )  RATIONAL_B_SPLINE_CURVE ( ( 0.9999999999999998890, 0.9510565162951536422, 1.000000000000000000, 0.9510565162951535312, 1.000000000000000000, 0.9510565162951535312, 1.000000000000000000, 0.9510565162951535312, 1.000000000000000000, 0.9510565162951533091, 1.000000000000000222 ) ) 
 REPRESENTATION_ITEM ( '' )  );
#193804=CARTESIAN_POINT ( 'NONE',  ( 1.993301997531345686E-15, -30.30510711980685556, 146.7500000054623683 ) ) ;
#193819=EDGE_LOOP ( 'NONE', ( #197427, #98773, #45334, #33633 ) ) ;
#193885=CARTESIAN_POINT ( 'NONE',  ( -32.00000000000000711, -1.163414459189985801E-14, 92.30000000000001137 ) ) ;
#193961=CARTESIAN_POINT ( 'NONE',  ( -7.963732510761932559, 36.86606204792785491, -8.000000000000001776 ) ) ;
#193964=CARTESIAN_POINT ( 'NONE',  ( 36.91128768240056246, 2.428612879436746321E-14, 50.50000000000002842 ) ) ;
#193976=ORIENTED_EDGE ( 'NONE', *, *, #100974, .F. ) ;
#194016=CARTESIAN_POINT ( 'NONE',  ( -35.09778042078744420, 5.635567127521238007, 40.04523299337172659 ) ) ;
#194025=DIRECTION ( 'NONE',  ( -1.000000000000000000, 0.000000000000000000, 0.000000000000000000 ) ) ;
#194242=CYLINDRICAL_SURFACE ( 'NONE', #114700, 2.649999999999999467 ) ;
#194254=CARTESIAN_POINT ( 'NONE',  ( 11.40812507854754365, 35.11059874428196537, -1.724999997268813479 ) ) ;
#194279=CARTESIAN_POINT ( 'NONE',  ( 22.44159573604009239, 16.30477369853692693, 142.5750000027311728 ) ) ;
#194353=CARTESIAN_POINT ( 'NONE',  ( 8.571926809382603096, -26.38167802310801235, 139.9750000027311785 ) ) ;
#194354=ADVANCED_FACE ( 'NONE', ( #20529 ), #97350, .F. ) ;
#194357=CYLINDRICAL_SURFACE ( 'NONE', #74152, 37.99626262588765968 ) ;
#194425=CARTESIAN_POINT ( 'NONE',  ( -11.74264578624799782, -36.14014761921581709, -9.349999994537627757 ) ) ;
#194460=CARTESIAN_POINT ( 'NONE',  ( 32.53418548917480990, 2.421649558188258666, 87.88477275112332165 ) ) ;
#194474=CARTESIAN_POINT ( 'NONE',  ( 36.80083376053583066, 5.466397602639213815, 45.70522705241149453 ) ) ;
#194477=CARTESIAN_POINT ( 'NONE',  ( -34.46950536905809770, -7.498137530812974738, 44.48224578455060652 ) ) ;
#194505=CARTESIAN_POINT ( 'NONE',  ( -36.93866063236283281, 5.356020730800094221, 43.73704834337281966 ) ) ;
#194589=CARTESIAN_POINT ( 'NONE',  ( -31.45250202946436247, 4.971043627493211048, 100.6372900316469412 ) ) ;
#194631=CARTESIAN_POINT ( 'NONE',  ( -38.00000000000000711, 2.428612866367529932E-14, -2.000000000000000000 ) ) ;
#194678=ORIENTED_EDGE ( 'NONE', *, *, #54770, .F. ) ;
#194742=PLANE ( 'NONE',  #133395 ) ;
#194750=CARTESIAN_POINT ( 'NONE',  ( 17.81289503416610742, 24.51734667627700404, 143.2999999999999829 ) ) ;
#194782=LINE ( 'NONE', #85583, #127522 ) ;
#194923=VECTOR ( 'NONE', #73219, 1000.000000000000114 ) ;
#194939=CARTESIAN_POINT ( 'NONE',  ( -17.81289503416611808, 24.51734667627700404, 145.6999999999999886 ) ) ;
#194953=CARTESIAN_POINT ( 'NONE',  ( -15.89947302414459607, 34.30766951777760454, -8.000000000000000000 ) ) ;
#194956=CARTESIAN_POINT ( 'NONE',  ( 1.993301997531345686E-15, -30.30510711980685556, 144.4999999999999716 ) ) ;
#194983=CARTESIAN_POINT ( 'NONE',  ( 29.86685920354754842, -21.69954338932559068, -9.824999997268813345 ) ) ;
#195006=CARTESIAN_POINT ( 'NONE',  ( -34.64436006561231096, 3.766901597203496710, 51.50401746017936944 ) ) ;
#195096=AXIS2_PLACEMENT_3D ( 'NONE', #152521, #51058, #33906 ) ;
#195272=ORIENTED_EDGE ( 'NONE', *, *, #108717, .T. ) ;
#195278=CARTESIAN_POINT ( 'NONE',  ( -17.14385361876520619, 23.59649016807275856, 147.0750000027311728 ) ) ;
#195312=CARTESIAN_POINT ( 'NONE',  ( -20.34036572606774484, 20.41983568886641365, 139.9999999999999716 ) ) ;
#195349=EDGE_LOOP ( 'NONE', ( #198524, #88018 ) ) ;
#195430=CARTESIAN_POINT ( 'NONE',  ( -29.86685920354755552, 21.69954338932564397, -1.324999997268813345 ) ) ;
#195475=CARTESIAN_POINT ( 'NONE',  ( 31.60163464511076015, -3.334671618079683597, 101.7358725107059598 ) ) ;
#195482=CARTESIAN_POINT ( 'NONE',  ( 36.99206003604233217, 5.206627989871538631, 43.21856904651838960 ) ) ;
#195485=CARTESIAN_POINT ( 'NONE',  ( -34.80541354469661997, -6.720605140086532536, 41.66184804092133476 ) ) ;
#195515=CARTESIAN_POINT ( 'NONE',  ( 11.40812507854754365, 35.11059874428196537, -7.224999997268813701 ) ) ;
#195526=CARTESIAN_POINT ( 'NONE',  ( -22.44159573604009950, -16.30477369853688430, 145.0750000027311728 ) ) ;
#195531=CARTESIAN_POINT ( 'NONE',  ( -40.00200000000003087, -4.592425496802575156E-15, 52.50000000000000000 ) ) ;
#195601=DIRECTION ( 'NONE',  ( 1.000000000000000000, 0.000000000000000000, 0.000000000000000000 ) ) ;
#195627=DIRECTION ( 'NONE',  ( 0.000000000000000000, 0.000000000000000000, -1.000000000000000000 ) ) ;
#195643=CARTESIAN_POINT ( 'NONE',  ( 23.48529157249599919, 32.32473071737754111, -2.700000000000000622 ) ) ;
#195651=AXIS2_PLACEMENT_3D ( 'NONE', #14328, #44676, #106329 ) ;
#195762=CARTESIAN_POINT ( 'NONE',  ( -23.31738231874055245, -16.94106989632524574, 140.1999999999999886 ) ) ;
#195764=CARTESIAN_POINT ( 'NONE',  ( -23.31738231874055245, -16.94106989632524574, 138.4500000054623570 ) ) ;
#195780=ORIENTED_EDGE ( 'NONE', *, *, #65731, .T. ) ;
#195802=ADVANCED_FACE ( 'NONE', ( #61161 ), #122833, .F. ) ;
#195820=ORIENTED_EDGE ( 'NONE', *, *, #72341, .T. ) ;
#195880=LINE ( 'NONE', #9847, #140384 ) ;
#195896=CARTESIAN_POINT ( 'NONE',  ( 37.54768727782017379, -1.429952535790606882, 39.67699414429140603 ) ) ;
#195968=CARTESIAN_POINT ( 'NONE',  ( 25.79464582014989205, 26.76891920992428453, -8.000000000000003553 ) ) ;
#195987=FACE_OUTER_BOUND ( 'NONE', #152737, .T. ) ;
#195997=CARTESIAN_POINT ( 'NONE',  ( -26.63278688795740834, 27.10001173645601114, -8.000000000000000000 ) ) ;
#195999=CARTESIAN_POINT ( 'NONE',  ( -32.00000000000000711, -5.510910596163089556E-15, 42.29999999999999716 ) ) ;
#196019=CARTESIAN_POINT ( 'NONE',  ( -34.78522506798724123, 0.4969912795167322761, 52.50000000000002132 ) ) ;
#196036=CIRCLE ( 'NONE', #141149, 28.82186960331498682 ) ;
#196076=CIRCLE ( 'NONE', #118553, 0.2000000000000057288 ) ;
#196214=ORIENTED_EDGE ( 'NONE', *, *, #137780, .T. ) ;
#196245=CARTESIAN_POINT ( 'NONE',  ( 11.40812507854755253, -35.11059874428192273, -4.524999997268813523 ) ) ;
#196251=CARTESIAN_POINT ( 'NONE',  ( -33.90027759800518936, -5.214635694306275049, 93.21535130585120044 ) ) ;
#196252=CARTESIAN_POINT ( 'NONE',  ( -36.29667422526105725, -10.80772347165230052, -7.999999999999994671 ) ) ;
#196264=CARTESIAN_POINT ( 'NONE',  ( 29.86685920354754487, 21.69954338932564752, -1.924999997268813212 ) ) ;
#196433=CARTESIAN_POINT ( 'NONE',  ( 38.00000000000000711, -12.34694845685040754, -10.84999999453762598 ) ) ;
#196516=CARTESIAN_POINT ( 'NONE',  ( -37.55508611250748885, 1.249935417488349021, 39.64085810587564396 ) ) ;
#196528=CARTESIAN_POINT ( 'NONE',  ( 8.571926809382597767, 26.38167802310806209, 144.2750000027311899 ) ) ;
#196633=EDGE_LOOP ( 'NONE', ( #41780, #72073, #109450, #8406 ) ) ;
#196638=CARTESIAN_POINT ( 'NONE',  ( 11.74264578624800315, -36.14014761921581709, -3.400000000000000355 ) ) ;
#196641=PLANE ( 'NONE',  #56780 ) ;
#196757=CARTESIAN_POINT ( 'NONE',  ( 17.81289503416611453, -24.51734667627695785, 138.9500000054623570 ) ) ;
#196807=ADVANCED_FACE ( 'NONE', ( #148980 ), #25651, .F. ) ;
#196847=CIRCLE ( 'NONE', #112797, 0.1999999999999987899 ) ;
#196982=CARTESIAN_POINT ( 'NONE',  ( -27.73933785331498925, -9.013057229001049109, 143.4750000027311785 ) ) ;
#197007=CARTESIAN_POINT ( 'NONE',  ( -34.71410084532070073, 2.653616468751188506, 52.01918243487460103 ) ) ;
#197071=LINE ( 'NONE', #14016, #104796 ) ;
#197084=CARTESIAN_POINT ( 'NONE',  ( 37.99626262588765258, 2.893932880411085066E-14, -3.002157773949822861 ) ) ;
#197098=ORIENTED_EDGE ( 'NONE', *, *, #162675, .T. ) ;
#197168=EDGE_CURVE ( 'NONE', #157920, #97386, #167207, .T. ) ;
#197224=CARTESIAN_POINT ( 'NONE',  ( 11.40812507854754365, 35.11059874428196537, -5.724999997268812812 ) ) ;
#197230=CARTESIAN_POINT ( 'NONE',  ( -28.41048423428186354, -24.65169963600693492, -8.000000000000001776 ) ) ;
#197242=CARTESIAN_POINT ( 'NONE',  ( -29.86685920354755552, 21.69954338932564397, -1.324999997268813345 ) ) ;
#197263=CARTESIAN_POINT ( 'NONE',  ( -31.72709406046300629, -0.4963711039036964312, 102.5000000000000142 ) ) ;
#197333=DIRECTION ( 'NONE',  ( 0.000000000000000000, 0.000000000000000000, 1.000000000000000000 ) ) ;
#197411=CARTESIAN_POINT ( 'NONE',  ( 3.556970738554033499E-15, -38.81732327939057825, -2.624999997268812724 ) ) ;
#197422=ORIENTED_EDGE ( 'NONE', *, *, #176321, .F. ) ;
#197427=ORIENTED_EDGE ( 'NONE', *, *, #78948, .F. ) ;
#197481=ORIENTED_EDGE ( 'NONE', *, *, #108717, .F. ) ;
#197500=CARTESIAN_POINT ( 'NONE',  ( -27.73933785331498925, -9.013057229001049109, 146.9750000027311785 ) ) ;
#197505=CARTESIAN_POINT ( 'NONE',  ( -22.44159573604010305, 16.30477369853692338, 144.6750000027311671 ) ) ;
#197509=FACE_OUTER_BOUND ( 'NONE', #34625, .T. ) ;
#197614=CARTESIAN_POINT ( 'NONE',  ( 11.74264578624800315, -36.14014761921581709, -1.399999999999999689 ) ) ;
#197664=CARTESIAN_POINT ( 'NONE',  ( 34.78522506798722702, 0.4969912795167628072, 52.50000000000000000 ) ) ;
#197677=ORIENTED_EDGE ( 'NONE', *, *, #190781, .F. ) ;
#197732=CARTESIAN_POINT ( 'NONE',  ( -23.31738231874055600, 16.94106989632528837, 144.0500000054623513 ) ) ;
#197932=CARTESIAN_POINT ( 'NONE',  ( 18.55831789572370383, 32.36956839859214341, -7.999999999999994671 ) ) ;
#197962=CARTESIAN_POINT ( 'NONE',  ( -27.73933785331498925, -9.013057229001049109, 141.4750000027311785 ) ) ;
#197969=DIRECTION ( 'NONE',  ( 0.000000000000000000, 0.000000000000000000, -1.000000000000000000 ) ) ;
#197986=CARTESIAN_POINT ( 'NONE',  ( 8.906447517083057264, -27.41122689804191026, 144.8500000054623911 ) ) ;
#198005=CARTESIAN_POINT ( 'NONE',  ( -37.45873412500000654, 2.428612866367529932E-14, -0.3124999986344065839 ) ) ;
#198008=CARTESIAN_POINT ( 'NONE',  ( -3.573655867282028392E-15, 2.428612866367529932E-14, 2.000000000000000000 ) ) ;
#198023=ORIENTED_EDGE ( 'NONE', *, *, #12852, .F. ) ;
#198093=DIRECTION ( 'NONE',  ( 1.000000000000000000, -0.000000000000000000, -0.000000000000000000 ) ) ;
#198163=CARTESIAN_POINT ( 'NONE',  ( 16.41480162262169529, -33.15536704053023698, -8.000000000000000000 ) ) ;
#198178=DIRECTION ( 'NONE',  ( 0.000000000000000000, 0.000000000000000000, -1.000000000000000000 ) ) ;
#198204=CARTESIAN_POINT ( 'NONE',  ( -11.40812507854754720, -35.11059874428192273, -10.72499999726881548 ) ) ;
#198210=CARTESIAN_POINT ( 'NONE',  ( 34.02686120844015960, 4.767814797156205486, 92.23495037107730354 ) ) ;
#198249=CARTESIAN_POINT ( 'NONE',  ( 1.784210473542230573E-15, -29.16686587814331588, 139.8750000027311842 ) ) ;
#198292=CARTESIAN_POINT ( 'NONE',  ( 23.31738231874054890, -16.94106989632523508, 143.0500000054623513 ) ) ;
#198340=VECTOR ( 'NONE', #116621, 1000.000000000000000 ) ;
#198391=CARTESIAN_POINT ( 'NONE',  ( 22.81625015709509441, 31.40387420917330275, -5.824999997268813345 ) ) ;
#198404=AXIS2_PLACEMENT_3D ( 'NONE', #110861, #188719, #50203 ) ;
#198419=EDGE_CURVE ( 'NONE', #4689, #21447, #168377, .T. ) ;
#198462=VECTOR ( 'NONE', #66717, 1000.000000000000000 ) ;
#198485=CARTESIAN_POINT ( 'NONE',  ( -17.14385361876520264, -23.59649016807271593, 145.1750000027311387 ) ) ;
#198490=CARTESIAN_POINT ( 'NONE',  ( 1.784210473542230573E-15, -29.16686587814331588, 141.3750000027311557 ) ) ;
#198524=ORIENTED_EDGE ( 'NONE', *, *, #5174, .F. ) ;
#198565=CARTESIAN_POINT ( 'NONE',  ( -17.14385361876520975, 23.59649016807275856, 149.0750000027312012 ) ) ;
#198658=CARTESIAN_POINT ( 'NONE',  ( 34.87691056670618650, 6.486286472422006177, 41.22672555304436770 ) ) ;
#198726=AXIS2_PLACEMENT_3D ( 'NONE', #170895, #123379, #32387 ) ;
#198797=AXIS2_PLACEMENT_3D ( 'NONE', #84466, #131993, #23825 ) ;
#198957=CARTESIAN_POINT ( 'NONE',  ( 8.571926809382597767, 26.38167802310806209, 146.7750000027311899 ) ) ;
#198980=CARTESIAN_POINT ( 'NONE',  ( -28.82186960331499392, 9.364793116373565596, 146.1500000054623456 ) ) ;
#199007=DIRECTION ( 'NONE',  ( 1.000000000000000000, 0.000000000000000000, 0.000000000000000000 ) ) ;
#199065=CARTESIAN_POINT ( 'NONE',  ( -22.44159573604009950, -16.30477369853688430, 139.5750000027311728 ) ) ;
#199083=CARTESIAN_POINT ( 'NONE',  ( -11.74149087413295511, 36.13659316521247433, -2.402157773949822772 ) ) ;
#199091=( BOUNDED_CURVE ( )  B_SPLINE_CURVE ( 2, ( #171730, #91871, #48393, #153564, #109053, #183917, #49377, #138397, #110050, #2869, #154563 ),
 .UNSPECIFIED., .F., .F. ) 
 B_SPLINE_CURVE_WITH_KNOTS ( ( 3, 2, 2, 2, 2, 3 ),
 ( 0.6000000000000005329, 0.6200000000000005507, 0.6400000000000005684, 0.6600000000000006972, 0.6800000000000007150, 0.7000000000000006217 ),
 .UNSPECIFIED. ) 
 CURVE ( )  GEOMETRIC_REPRESENTATION_ITEM ( )  RATIONAL_B_SPLINE_CURVE ( ( 0.9999999999999986677, 0.9510565162951548634, 1.000000000000000000, 0.9510565162951535312, 1.000000000000000000, 0.9510565162951535312, 1.000000000000000000, 0.9510565162951535312, 1.000000000000000000, 0.9510565162951518658, 1.000000000000001554 ) ) 
 REPRESENTATION_ITEM ( '' )  );
#199104=DIRECTION ( 'NONE',  ( 0.000000000000000000, 0.000000000000000000, 1.000000000000000000 ) ) ;
#199195=CARTESIAN_POINT ( 'NONE',  ( -36.91746825000001309, 11.99521256947798342, -7.224999997268814589 ) ) ;
#199202=CARTESIAN_POINT ( 'NONE',  ( 34.16333257229420894, 4.138830072290155648, 91.36021987110629539 ) ) ;
#199213=CARTESIAN_POINT ( 'NONE',  ( 3.556970738554034288E-15, -38.81732327939057114, -6.624999997268814056 ) ) ;
#199310=CARTESIAN_POINT ( 'NONE',  ( 67.00000000000000000, -1.163414459189985801E-14, 95.00000000000000000 ) ) ;
#199313=ORIENTED_EDGE ( 'NONE', *, *, #156518, .F. ) ;
#199388=CARTESIAN_POINT ( 'NONE',  ( -29.86685920354755197, -21.69954338932560134, -8.924999997268812990 ) ) ;
#199405=ORIENTED_EDGE ( 'NONE', *, *, #116835, .T. ) ;
#199457=ORIENTED_EDGE ( 'NONE', *, *, #56324, .F. ) ;
#199478=CARTESIAN_POINT ( 'NONE',  ( 22.44159573604009594, -16.30477369853687364, 147.6750000027311671 ) ) ;
#199483=CARTESIAN_POINT ( 'NONE',  ( 8.571926809382597767, 26.38167802310806209, 146.2750000027311899 ) ) ;
#199514=ORIENTED_EDGE ( 'NONE', *, *, #149523, .T. ) ;
#199644=CARTESIAN_POINT ( 'NONE',  ( -3.573655867282028392E-15, 2.428612866367529932E-14, 2.000000000000000000 ) ) ;
#199664=EDGE_CURVE ( 'NONE', #44725, #50285, #150851, .T. ) ;
#199672=DIRECTION ( 'NONE',  ( 1.000000000000000000, 0.000000000000000000, 0.000000000000000000 ) ) ;
#199677=ADVANCED_FACE ( 'NONE', ( #15953 ), #181391, .F. ) ;
#199732=VERTEX_POINT ( 'NONE', #96254 ) ;
#199836=CARTESIAN_POINT ( 'NONE',  ( 22.81625015709509441, 31.40387420917330275, -3.324999997268812901 ) ) ;
#199920=( BOUNDED_CURVE ( )  B_SPLINE_CURVE ( 2, ( #106972, #171641, #108967, #148773, #167672, #87087, #183832, #138316, #169649, #31145, #45322 ),
 .UNSPECIFIED., .F., .T. ) 
 B_SPLINE_CURVE_WITH_KNOTS ( ( 3, 2, 2, 2, 2, 3 ),
 ( 0.5000000000000001110, 0.5200000000000001288, 0.5400000000000001465, 0.5600000000000001643, 0.5800000000000000711, 0.6000000000000000888 ),
 .UNSPECIFIED. ) 
 CURVE ( )  GEOMETRIC_REPRESENTATION_ITEM ( )  RATIONAL_B_SPLINE_CURVE ( ( 0.9999999999999997780, 0.9510565162951537532, 1.000000000000000000, 0.9510565162951535312, 1.000000000000000000, 0.9510565162951535312, 1.000000000000000000, 0.9510565162951535312, 1.000000000000000000, 0.9510565162951533091, 1.000000000000000222 ) ) 
 REPRESENTATION_ITEM ( '' )  );
#199924=CARTESIAN_POINT ( 'NONE',  ( -36.78376627615639904, -4.378768456387976293, 48.34741972342521166 ) ) ;
#199953=CARTESIAN_POINT ( 'NONE',  ( 27.73933785331498925, -9.013057229001033122, 144.2750000027311899 ) ) ;
#199975=CARTESIAN_POINT ( 'NONE',  ( -28.82186960331499392, -9.364793116373526516, 140.0999999999999943 ) ) ;
#199976=CARTESIAN_POINT ( 'NONE',  ( -5.429308488886486681E-15, 30.30510711980690175, 145.7500000054623115 ) ) ;
#199993=FACE_OUTER_BOUND ( 'NONE', #31159, .T. ) ;
#199996=DIRECTION ( 'NONE',  ( -1.000000000000000000, 0.000000000000000000, 0.000000000000000000 ) ) ;
#200018=VERTEX_POINT ( 'NONE', #37579 ) ;
#200063=CARTESIAN_POINT ( 'NONE',  ( -27.73933785331498925, 9.013057229001088189, 146.7750000027311899 ) ) ;
#200078=CARTESIAN_POINT ( 'NONE',  ( 37.99626262588768810, 12.34573411038912027, -4.647842220587803830 ) ) ;
#200080=CARTESIAN_POINT ( 'NONE',  ( -6.019987952026120409E-15, 39.95163481335720235, -6.502157773949823749 ) ) ;
#200116=CARTESIAN_POINT ( 'NONE',  ( 28.82186960331500813, 9.364793116373537174, 149.0999999999999943 ) ) ;
#200142=CARTESIAN_POINT ( 'NONE',  ( 22.55659503568693580, -29.32441354047577065, -8.000000000000001776 ) ) ;
#200184=CARTESIAN_POINT ( 'NONE',  ( -29.86685920354755552, 21.69954338932564397, -9.324999997268813345 ) ) ;
ENDSEC;
END-ISO-10303-21;
